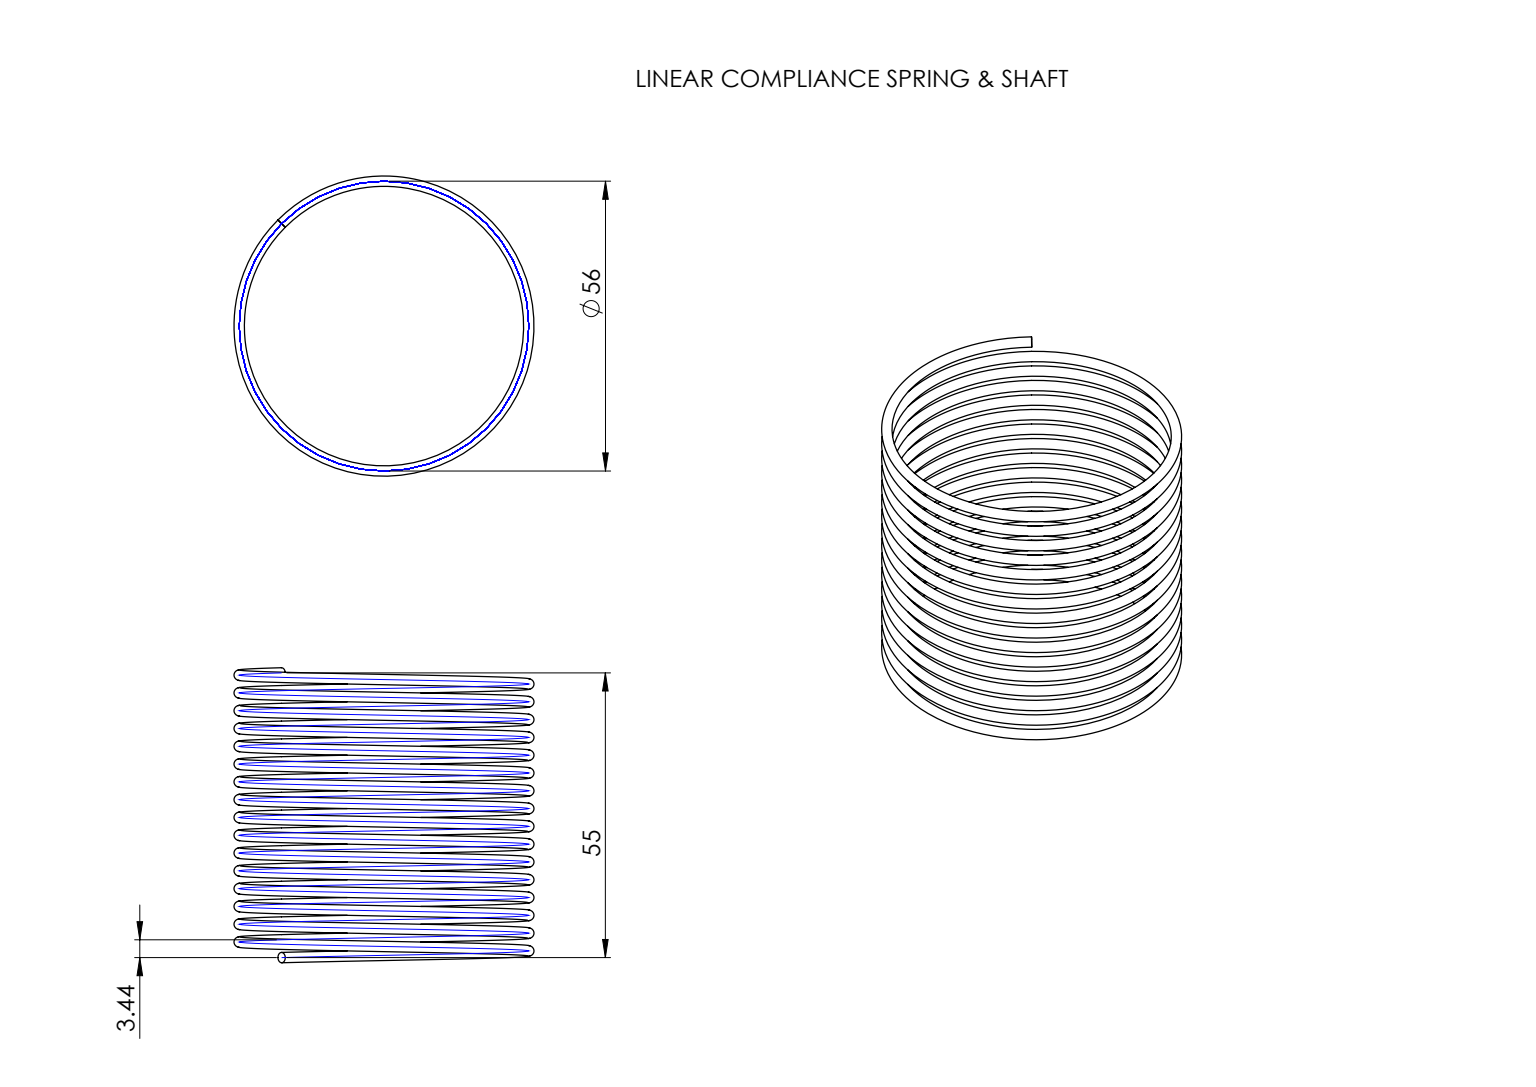
ISO-10303-21;
HEADER;
FILE_DESCRIPTION (('STEP AP214'),
    '1' );
FILE_NAME ('Linear Compliance Spring & Shaft.step',
    '2026-10-02T18:08:48',
    ( '' ),
    ( '' ),
    'SwSTEP 2.0',
    'SolidWorks 2026',
    '' );
FILE_SCHEMA (( 'AUTOMOTIVE_DESIGN' ));
ENDSEC;

DATA;
#1=CARTESIAN_POINT ( 'NONE',  ( -2.584737979205441561E-13, 22.74218749999999645, -30.02300923189239512 ) ) ;
#5=CARTESIAN_POINT ( 'NONE',  ( 0.04044903254992426173, 37.93006916759064495, -30.02300923189239867 ) ) ;
#8=CARTESIAN_POINT ( 'NONE',  ( -2.584737979205441561E-13, 43.36718749999999289, -30.02300923189239512 ) ) ;
#20=CARTESIAN_POINT ( 'NONE',  ( 28.01184896238290278, 23.45833333333333215, -7.505752307973347470 ) ) ;
#25=CARTESIAN_POINT ( 'NONE',  ( -13.94119854578892514, 33.62201416574269075, 24.22776226481266448 ) ) ;
#32=CARTESIAN_POINT ( 'NONE',  ( -26.07999730980477437, 56.11458333333332860, 6.988114217768305103 ) ) ;
#37=CARTESIAN_POINT ( 'NONE',  ( -6.988114217767819270, 38.35416666666666430, 26.07999730980490583 ) ) ;
#38=CARTESIAN_POINT ( 'NONE',  ( 30.02300923189239867, 28.47694416759064495, 0.04044903254992252006 ) ) ;
#39=CARTESIAN_POINT ( 'NONE',  ( 7.543491769121922985, 16.00482666574268720, 28.00173670424535644 ) ) ;
#44=CARTESIAN_POINT ( 'NONE',  ( -14.01125832528328985, 48.51784749907601935, -24.18731323226223040 ) ) ;
#50=CARTESIAN_POINT ( 'NONE',  ( -24.22776226481240514, 43.65923583425730925, 13.94119854578937812 ) ) ;
#54=CARTESIAN_POINT ( 'NONE',  ( 15.01150461594596308, 19.59114583333332149, -26.00068869287367335 ) ) ;
#58=CARTESIAN_POINT ( 'NONE',  ( -7.505752307973343918, 46.66145833333332860, -28.01184896238290989 ) ) ;
#63=CARTESIAN_POINT ( 'NONE',  ( 7.543491769121922985, 64.12982666574268364, 28.00173670424535644 ) ) ;
#69=CARTESIAN_POINT ( 'NONE',  ( 27.95245687107223276, 61.41406250000000711, -2.463307335887066074E-13 ) ) ;
#72=CARTESIAN_POINT ( 'NONE',  ( 24.20753774853731244, 30.19010416666665719, -13.97622843553632599 ) ) ;
#80=CARTESIAN_POINT ( 'NONE',  ( 13.94119854578937812, 56.54986083425731636, 24.22776226481240514 ) ) ;
#91=CARTESIAN_POINT ( 'NONE',  ( -0.04044903254992426173, 15.58631916759064495, 27.95245687107223276 ) ) ;
#95=CARTESIAN_POINT ( 'NONE',  ( 7.505752307972854531, 43.51041666666666430, -28.01184896238303423 ) ) ;
#99=CARTESIAN_POINT ( 'NONE',  ( 28.01184896238304134, 16.86979166666666075, 7.505752307972846538 ) ) ;
#104=CARTESIAN_POINT ( 'NONE',  ( -7.543491769121917656, 31.47357666574268364, -28.00173670424536354 ) ) ;
#106=CARTESIAN_POINT ( 'NONE',  ( 28.01184896238304134, 37.49479166666666430, 7.505752307972846538 ) ) ;
#111=CARTESIAN_POINT ( 'NONE',  ( -24.18731323226221974, 61.40847249907603356, 14.01125832528330406 ) ) ;
#116=CARTESIAN_POINT ( 'NONE',  ( 26.07999730980477437, 16.58333333333333215, -6.988114217768290004 ) ) ;
#125=CARTESIAN_POINT ( 'NONE',  ( 24.22776226481265383, 22.45013916574269075, 13.94119854578893580 ) ) ;
#129=CARTESIAN_POINT ( 'NONE',  ( -19.09188309203694445, 42.93750000000000000, -19.09188309203661049 ) ) ;
#134=CARTESIAN_POINT ( 'NONE',  ( -15.04653450569291984, 63.99777750092396644, 25.98046417659859486 ) ) ;
#135=CARTESIAN_POINT ( 'NONE',  ( -30.02300923189239867, 16.44569416759064140, -0.04044903254991731589 ) ) ;
#146=( LENGTH_UNIT ( ) NAMED_UNIT ( * ) SI_UNIT ( .MILLI., .METRE. ) );
#156=CARTESIAN_POINT ( 'NONE',  ( 0.04044903254993986036, 31.05506916759064495, -27.95245687107223986 ) ) ;
#164=CARTESIAN_POINT ( 'NONE',  ( -7.543491769121917656, 48.66107666574268364, -28.00173670424536354 ) ) ;
#168=CARTESIAN_POINT ( 'NONE',  ( 27.95245687107222921, 20.16406249999999645, -2.463307335887066074E-13 ) ) ;
#171=CARTESIAN_POINT ( 'NONE',  ( 15.01150461594596308, 19.59114583333332149, -26.00068869287367335 ) ) ;
#175=CARTESIAN_POINT ( 'NONE',  ( -0.04044903254990864921, 43.08631916759065916, 30.02300923189239867 ) ) ;
#177=CARTESIAN_POINT ( 'NONE',  ( -26.00068869287368756, 53.10677083333331439, -15.01150461594595775 ) ) ;
#189=CARTESIAN_POINT ( 'NONE',  ( -7.505752307973343918, 26.03645833333333215, -28.01184896238290989 ) ) ;
#194=CARTESIAN_POINT ( 'NONE',  ( 7.025853678916867295, 36.62982666574267654, 26.06988505166722803 ) ) ;
#201=CARTESIAN_POINT ( 'NONE',  ( 19.09188309203694800, 58.40625000000000711, 19.09188309203660694 ) ) ;
#205=CARTESIAN_POINT ( 'NONE',  ( -19.09188309203694445, 42.93750000000000000, -19.09188309203661049 ) ) ;
#206=CARTESIAN_POINT ( 'NONE',  ( -20.47846945139902175, 34.06288166759063785, -20.53372385742072481 ) ) ;
#207=CARTESIAN_POINT ( 'NONE',  ( -25.98046417659831420, 16.72097249907602290, 15.04653450569339945 ) ) ;
#212=CARTESIAN_POINT ( 'NONE',  ( 19.11951029504797006, 43.21836833240935505, 19.06425588902558133 ) ) ;
#218=CARTESIAN_POINT ( 'NONE',  ( -24.18731323226248264, 44.23215250092398065, -14.01125832528284931 ) ) ;
#222=CARTESIAN_POINT ( 'NONE',  ( 15.01150461594643204, 27.61197916666666430, 26.00068869287340334 ) ) ;
#227=CARTESIAN_POINT ( 'NONE',  ( -7.505752307972844761, 48.66666666666666430, 28.01184896238304134 ) ) ;
#235=CARTESIAN_POINT ( 'NONE',  ( -30.02300923189239867, 61.69493083240936926, 0.04044903255044988294 ) ) ;
#241=CARTESIAN_POINT ( 'NONE',  ( 13.97622843553589966, 57.40364583333332860, -24.20753774853756113 ) ) ;
#244=CARTESIAN_POINT ( 'NONE',  ( -27.95245687107222921, 32.19531250000000000, 2.498001805406602216E-13 ) ) ;
#251=CARTESIAN_POINT ( 'NONE',  ( -13.94119854578936923, 54.83111083425730214, -24.22776226481241224 ) ) ;
#262=CARTESIAN_POINT ( 'NONE',  ( 19.06425588902592239, 11.71913166759064318, 19.11951029504763611 ) ) ;
#267=CARTESIAN_POINT ( 'NONE',  ( 28.01184896238290278, 44.08333333333332860, -7.505752307973347470 ) ) ;
#271=CARTESIAN_POINT ( 'NONE',  ( -28.01184896238304134, 25.46354166666666430, -7.505752307972844761 ) ) ;
#277=CARTESIAN_POINT ( 'NONE',  ( -20.53372385742107653, 31.18711833240935150, -20.47846945139867003 ) ) ;
#279=CARTESIAN_POINT ( 'NONE',  ( -20.50609665441004736, 53.25000000000000000, -20.50609665440969565 ) ) ;
#285=CARTESIAN_POINT ( 'NONE',  ( 6.950374756619257965, 62.69753499907601224, -26.09010956794244507 ) ) ;
#291=CARTESIAN_POINT ( 'NONE',  ( -19.09188309203660694, 18.01562499999999645, 19.09188309203694800 ) ) ;
#299=CARTESIAN_POINT ( 'NONE',  ( -7.025853678916861966, 17.72357666574268720, -26.06988505166722803 ) ) ;
#303=CARTESIAN_POINT ( 'NONE',  ( 19.09188309203694800, 48.09375000000000000, 19.09188309203660694 ) ) ;
#307=CARTESIAN_POINT ( 'NONE',  ( -30.02300923189239512, 15.00781249999999467, 2.654126918244515359E-13 ) ) ;
#308=CARTESIAN_POINT ( 'NONE',  ( -25.98046417659859486, 13.29465250092397532, -15.04653450569291628 ) ) ;
#318=SURFACE_SIDE_STYLE ('',( #28646 ) ) ;
#331=CARTESIAN_POINT ( 'NONE',  ( 13.94119854578937812, 25.61236083425731636, 24.22776226481240514 ) ) ;
#339=CARTESIAN_POINT ( 'NONE',  ( 30.02300923189239867, 42.78868083240935505, -0.04044903255044467877 ) ) ;
#343=CARTESIAN_POINT ( 'NONE',  ( 13.97622843553633665, 13.86197916666666430, 24.20753774853730889 ) ) ;
#346=CARTESIAN_POINT ( 'NONE',  ( -7.505752307972844761, 21.16666666666666430, 28.01184896238304134 ) ) ;
#351=CARTESIAN_POINT ( 'NONE',  ( -26.02091320914849959, 36.78423583425730214, 14.97647472619947528 ) ) ;
#353=CARTESIAN_POINT ( 'NONE',  ( -28.01184896238304134, 52.96354166666666430, -7.505752307972844761 ) ) ;
#363=CARTESIAN_POINT ( 'NONE',  ( 7.505752307972854531, 22.88541666666666430, -28.01184896238303423 ) ) ;
#368=CARTESIAN_POINT ( 'NONE',  ( -0.04044903255042732459, 35.05430583240935505, -27.95245687107223986 ) ) ;
#376=CARTESIAN_POINT ( 'NONE',  ( -24.20753774853730889, 62.84635416666667851, 13.97622843553633842 ) ) ;
#380=CARTESIAN_POINT ( 'NONE',  ( -27.95245687107223276, 42.50781249999998579, 2.498001805406602216E-13 ) ) ;
#381=CARTESIAN_POINT ( 'NONE',  ( 0.04044903254992426173, 31.05506916759064495, -30.02300923189239867 ) ) ;
#383=CARTESIAN_POINT ( 'NONE',  ( -20.47846945139866648, 23.45274333240935150, 20.53372385742108008 ) ) ;
#387=CARTESIAN_POINT ( 'NONE',  ( -19.06425588902558133, 44.07774333240935505, 19.11951029504797006 ) ) ;
#393=CARTESIAN_POINT ( 'NONE',  ( 26.09010956794232428, 52.39621500092398065, -6.950374756619718042 ) ) ;
#397=CARTESIAN_POINT ( 'NONE',  ( -7.505752307972844761, 28.04166666666666075, 28.01184896238304134 ) ) ;
#400=CARTESIAN_POINT ( 'NONE',  ( -15.01150461594595775, 45.37239583333333570, 26.00068869287368756 ) ) ;
#407=CARTESIAN_POINT ( 'NONE',  ( -26.02091320914878025, 65.41888916574268364, -14.97647472619899389 ) ) ;
#412=CARTESIAN_POINT ( 'NONE',  ( -6.988114217767819270, 62.41666666666666430, 26.07999730980490583 ) ) ;
#415=CARTESIAN_POINT ( 'NONE',  ( -6.988114217767819270, 31.47916666666666075, 26.07999730980490583 ) ) ;
#420=CARTESIAN_POINT ( 'NONE',  ( -26.06988505166735237, 54.40142333425730925, -7.025853678916388567 ) ) ;
#434=CARTESIAN_POINT ( 'NONE',  ( 27.95245687107223986, 25.03944416759064495, 0.04044903254993640479 ) ) ;
#439=CARTESIAN_POINT ( 'NONE',  ( -28.01184896238304134, 46.08854166666666430, -7.505752307972844761 ) ) ;
#442=CARTESIAN_POINT ( 'NONE',  ( -7.505752307973343918, 19.16145833333332860, -28.01184896238290989 ) ) ;
#449=CARTESIAN_POINT ( 'NONE',  ( -7.468012846824272799, 36.91628499907601224, 28.02196122052058413 ) ) ;
#451=CARTESIAN_POINT ( 'NONE',  ( -26.00068869287340334, 49.09635416666666430, 15.01150461594643559 ) ) ;
#457=CARTESIAN_POINT ( 'NONE',  ( 26.06988505166722803, 63.27045166574269075, -7.025853678916862854 ) ) ;
#463=CARTESIAN_POINT ( 'NONE',  ( 19.09188309203694800, 24.03124999999999645, 19.09188309203660694 ) ) ;
#470=CARTESIAN_POINT ( 'NONE',  ( -19.06425588902558133, 26.89024333240934439, 19.11951029504797006 ) ) ;
#473=CARTESIAN_POINT ( 'NONE',  ( -13.97622843553588901, 48.80989583333332860, 24.20753774853756823 ) ) ;
#477=CARTESIAN_POINT ( 'NONE',  ( 28.01184896238304134, 16.86979166666666075, 7.505752307972846538 ) ) ;
#478=CARTESIAN_POINT ( 'NONE',  ( -7.543491769121417612, 15.72954833425730925, 28.00173670424549499 ) ) ;
#500=CARTESIAN_POINT ( 'NONE',  ( -26.09010956794232428, 36.92746500092395934, 6.950374756619732253 ) ) ;
#508=CARTESIAN_POINT ( 'NONE',  ( 26.02091320914876960, 53.38763916574269786, 14.97647472619900455 ) ) ;
#512=CARTESIAN_POINT ( 'NONE',  ( 19.09188309203694800, 13.71874999999999467, 19.09188309203660694 ) ) ;
#514=CARTESIAN_POINT ( 'NONE',  ( -15.01150461594595775, 17.87239583333332149, 26.00068869287368756 ) ) ;
#517=CARTESIAN_POINT ( 'NONE',  ( 28.02196122052045268, 42.08371500092398065, -7.468012846824774620 ) ) ;
#519=CARTESIAN_POINT ( 'NONE',  ( 28.01184896238304134, 51.24479166666666430, 7.505752307972846538 ) ) ;
#520=CARTESIAN_POINT ( 'NONE',  ( -26.00068869287340334, 66.28385416666662877, 15.01150461594643382 ) ) ;
#529=CARTESIAN_POINT ( 'NONE',  ( 7.505752307973351023, 20.88020833333333215, 28.01184896238290278 ) ) ;
#540=CARTESIAN_POINT ( 'NONE',  ( -2.428612866367529427E-13, 60.55468749999999289, -27.95245687107222921 ) ) ;
#544=CARTESIAN_POINT ( 'NONE',  ( -19.09188309203660694, 42.07812499999999289, 19.09188309203694800 ) ) ;
#546=CARTESIAN_POINT ( 'NONE',  ( -14.97647472619946285, 30.76861083425731280, -26.02091320914851025 ) ) ;
#547=CARTESIAN_POINT ( 'NONE',  ( 7.468012846824281681, 18.01003499907601935, -28.02196122052058058 ) ) ;
#553=CARTESIAN_POINT ( 'NONE',  ( 0.04044903255044120238, 47.08555583240935505, 27.95245687107223276 ) ) ;
#559=CARTESIAN_POINT ( 'NONE',  ( -24.22776226481240514, 50.53423583425731636, 13.94119854578937812 ) ) ;
#563=CARTESIAN_POINT ( 'NONE',  ( -20.50609665440969209, 24.89062500000000000, 20.50609665441005092 ) ) ;
#567=CARTESIAN_POINT ( 'NONE',  ( -7.505752307973343918, 50.09895833333332860, -28.01184896238290989 ) ) ;
#573=CARTESIAN_POINT ( 'NONE',  ( -7.543491769121917656, 58.97357666574269786, -28.00173670424536354 ) ) ;
#577=CARTESIAN_POINT ( 'NONE',  ( -19.09188309203694445, 63.56249999999999289, -19.09188309203661049 ) ) ;
#580=CARTESIAN_POINT ( 'NONE',  ( -24.20753774853756823, 29.04427083333332504, -13.97622843553588723 ) ) ;
#585=CARTESIAN_POINT ( 'NONE',  ( 27.95245687107223986, 59.41444416759064495, 0.04044903254993640479 ) ) ;
#596=CARTESIAN_POINT ( 'NONE',  ( 26.06988505166735592, 25.18267333425730214, 7.025853678916393896 ) ) ;
#600=AXIS2_PLACEMENT_3D ( 'NONE', #12178, #2052, #12527 ) ;
#602=CARTESIAN_POINT ( 'NONE',  ( -30.02300923189239512, 56.25781249999997868, 2.654126918244515359E-13 ) ) ;
#606=CARTESIAN_POINT ( 'NONE',  ( 20.50609665441005092, 24.03124999999999645, 20.50609665440969209 ) ) ;
#614=CARTESIAN_POINT ( 'NONE',  ( -28.02196122052058413, 30.90065999907601579, -7.468012846824272799 ) ) ;
#617=CARTESIAN_POINT ( 'NONE',  ( -15.01150461594595775, 45.37239583333332860, 26.00068869287368756 ) ) ;
#621=CARTESIAN_POINT ( 'NONE',  ( -14.01125832528328985, 62.26784749907602645, -24.18731323226223040 ) ) ;
#627=CARTESIAN_POINT ( 'NONE',  ( 24.20753774853731244, 23.31510416666666430, -13.97622843553633132 ) ) ;
#634=CARTESIAN_POINT ( 'NONE',  ( 7.025853678916867295, 29.75482666574269075, 26.06988505166722803 ) ) ;
#638=CARTESIAN_POINT ( 'NONE',  ( -26.07999730980490583, 52.96354166666666430, -6.988114217767815717 ) ) ;
#643=CARTESIAN_POINT ( 'NONE',  ( 26.00068869287340334, 19.87760416666666430, -15.01150461594642316 ) ) ;
#644=CARTESIAN_POINT ( 'NONE',  ( -20.53372385742071771, 19.45350666759063785, 20.47846945139902530 ) ) ;
#665=CARTESIAN_POINT ( 'NONE',  ( -14.01125832528285109, 43.37277750092397355, 24.18731323226248264 ) ) ;
#672=CARTESIAN_POINT ( 'NONE',  ( -26.02091320914878025, 58.54388916574269075, -14.97647472619899389 ) ) ;
#678=CARTESIAN_POINT ( 'NONE',  ( 6.988114217768294445, 24.31770833333332504, 26.07999730980477437 ) ) ;
#682=CARTESIAN_POINT ( 'NONE',  ( -15.01150461594642138, 32.76822916666666430, -26.00068869287340334 ) ) ;
#685=CARTESIAN_POINT ( 'NONE',  ( 30.02300923189239867, 42.22694416759065206, 0.04044903254992252006 ) ) ;
#687=CARTESIAN_POINT ( 'NONE',  ( 20.50609665441005092, 51.53124999999999289, 20.50609665440969209 ) ) ;
#688=CARTESIAN_POINT ( 'NONE',  ( 2.740863092043355209E-13, 65.71093749999997158, 30.02300923189239512 ) ) ;
#707=CARTESIAN_POINT ( 'NONE',  ( 26.09010956794232428, 14.58371500092397710, -6.950374756619718042 ) ) ;
#712=CARTESIAN_POINT ( 'NONE',  ( -13.97622843553632777, 53.39322916666665719, -24.20753774853731599 ) ) ;
#713=CARTESIAN_POINT ( 'NONE',  ( -15.04653450569291984, 33.06027750092398776, 25.98046417659859486 ) ) ;
#714=CARTESIAN_POINT ( 'NONE',  ( 28.02196122052058413, 32.61940999907601224, 7.468012846824272799 ) ) ;
#718=CARTESIAN_POINT ( 'NONE',  ( 24.22776226481265383, 43.07513916574269786, 13.94119854578893580 ) ) ;
#724=CARTESIAN_POINT ( 'NONE',  ( 26.09010956794232428, 48.95871500092396644, -6.950374756619718042 ) ) ;
#729=CARTESIAN_POINT ( 'NONE',  ( 30.02300923189239512, 23.60156250000000000, -2.619432448724977703E-13 ) ) ;
#733=CARTESIAN_POINT ( 'NONE',  ( 26.00068869287340334, 57.69010416666667140, -15.01150461594642316 ) ) ;
#738=CARTESIAN_POINT ( 'NONE',  ( -13.94119854578892514, 16.43451416574268720, 24.22776226481266448 ) ) ;
#746=CARTESIAN_POINT ( 'NONE',  ( 13.97622843553589966, 40.21614583333332860, -24.20753774853756113 ) ) ;
#753=CARTESIAN_POINT ( 'NONE',  ( 7.025853678916403666, 55.26079833425730214, -26.06988505166735237 ) ) ;
#758=CARTESIAN_POINT ( 'NONE',  ( -15.01150461594642138, 53.39322916666665009, -26.00068869287340334 ) ) ;
#770=CARTESIAN_POINT ( 'NONE',  ( -6.950374756619716266, 24.03684000092397000, -26.09010956794232428 ) ) ;
#775=CARTESIAN_POINT ( 'NONE',  ( -28.01184896238290278, 52.67708333333333570, 7.505752307973363457 ) ) ;
#779=CARTESIAN_POINT ( 'NONE',  ( -26.00068869287368756, 25.60677083333332149, -15.01150461594595775 ) ) ;
#785=CARTESIAN_POINT ( 'NONE',  ( -7.468012846824272799, 40.35378499907601935, 28.02196122052058413 ) ) ;
#787=CARTESIAN_POINT ( 'NONE',  ( -28.01184896238290278, 49.23958333333332860, 7.505752307973363457 ) ) ;
#790=CARTESIAN_POINT ( 'NONE',  ( 0.04044903255044120238, 60.83555583240935505, 27.95245687107223276 ) ) ;
#796=CARTESIAN_POINT ( 'NONE',  ( 13.97622843553589966, 19.59114583333332504, -24.20753774853756113 ) ) ;
#804=CARTESIAN_POINT ( 'NONE',  ( 19.06425588902558133, 28.60899333240935150, -19.11951029504797006 ) ) ;
#809=CARTESIAN_POINT ( 'NONE',  ( 6.988114217767829928, 50.38541666666666430, -26.07999730980489872 ) ) ;
#813=CARTESIAN_POINT ( 'NONE',  ( 26.00068869287340334, 26.75260416666666430, -15.01150461594642316 ) ) ;
#814=CARTESIAN_POINT ( 'NONE',  ( -15.04653450569291984, 22.74777750092397355, 25.98046417659859486 ) ) ;
#832=CARTESIAN_POINT ( 'NONE',  ( -27.95245687107223986, 37.07069416759063785, -0.04044903254993292840 ) ) ;
#839=CARTESIAN_POINT ( 'NONE',  ( -7.468012846824272799, 54.10378499907602645, 28.02196122052058413 ) ) ;
#845=CARTESIAN_POINT ( 'NONE',  ( -27.95245687107222921, 28.75781249999999645, 2.498001805406602216E-13 ) ) ;
#848=CARTESIAN_POINT ( 'NONE',  ( -7.505752307972844761, 28.04166666666666075, 28.01184896238304134 ) ) ;
#851=CARTESIAN_POINT ( 'NONE',  ( -28.00173670424549499, 50.96392333425730925, -7.543491769121417612 ) ) ;
#854=CARTESIAN_POINT ( 'NONE',  ( -28.01184896238290278, 56.11458333333332860, 7.505752307973363457 ) ) ;
#873=CARTESIAN_POINT ( 'NONE',  ( -6.950374756619716266, 13.72434000092397532, -26.09010956794232428 ) ) ;
#879=CARTESIAN_POINT ( 'NONE',  ( 19.09188309203661049, 54.10937499999999289, -19.09188309203694445 ) ) ;
#880=CARTESIAN_POINT ( 'NONE',  ( -20.53372385742071771, 43.51600666759065206, 20.47846945139902530 ) ) ;
#881=CARTESIAN_POINT ( 'NONE',  ( 28.02196122052058413, 25.74440999907601935, 7.468012846824272799 ) ) ;
#884=CARTESIAN_POINT ( 'NONE',  ( 13.94119854578893580, 59.40326416574269075, -24.22776226481265383 ) ) ;
#891=CARTESIAN_POINT ( 'NONE',  ( -24.22776226481240514, 47.09673583425730214, 13.94119854578937812 ) ) ;
#895=CARTESIAN_POINT ( 'NONE',  ( -30.02300923189239512, 25.32031250000000000, 2.654126918244515359E-13 ) ) ;
#899=CARTESIAN_POINT ( 'NONE',  ( -26.00068869287368756, 56.54427083333332149, -15.01150461594595775 ) ) ;
#905=CARTESIAN_POINT ( 'NONE',  ( -6.950374756619247307, 16.29128499907601579, 26.09010956794245217 ) ) ;
#913=CARTESIAN_POINT ( 'NONE',  ( -6.988114217768288228, 43.22395833333332860, -26.07999730980477437 ) ) ;
#919=CARTESIAN_POINT ( 'NONE',  ( -14.97647472619946285, 10.14361083425730925, -26.02091320914851025 ) ) ;
#920=CARTESIAN_POINT ( 'NONE',  ( 28.01184896238304134, 54.68229166666665719, 7.505752307972846538 ) ) ;
#931=CARTESIAN_POINT ( 'NONE',  ( 24.22776226481241224, 21.31548583425730925, -13.94119854578936923 ) ) ;
#937=CARTESIAN_POINT ( 'NONE',  ( -7.505752307972844761, 48.66666666666666430, 28.01184896238304134 ) ) ;
#941=CARTESIAN_POINT ( 'NONE',  ( 20.50609665441005092, 30.90624999999999645, 20.50609665440969209 ) ) ;
#946=CARTESIAN_POINT ( 'NONE',  ( 26.02091320914876960, 39.63763916574268364, 14.97647472619900455 ) ) ;
#948=CARTESIAN_POINT ( 'NONE',  ( 26.00068869287367690, 44.51302083333332860, 15.01150461594596486 ) ) ;
#951=CARTESIAN_POINT ( 'NONE',  ( -6.988114217768288228, 15.72395833333332860, -26.07999730980477437 ) ) ;
#957=CARTESIAN_POINT ( 'NONE',  ( -6.988114217767819270, 24.60416666666666430, 26.07999730980490583 ) ) ;
#964=CARTESIAN_POINT ( 'NONE',  ( 27.95245687107223276, 32.47618083240936215, -0.04044903255042905932 ) ) ;
#968=CARTESIAN_POINT ( 'NONE',  ( 27.95245687107222921, 51.10156249999998579, -2.463307335887066074E-13 ) ) ;
#973=CARTESIAN_POINT ( 'NONE',  ( -20.50609665440969209, 24.89062500000000000, 20.50609665441005092 ) ) ;
#974=CARTESIAN_POINT ( 'NONE',  ( 7.468012846824777284, 22.31809000092397000, 28.02196122052045268 ) ) ;
#982=CARTESIAN_POINT ( 'NONE',  ( -7.468012846824771955, 58.41184000092398065, -28.02196122052045624 ) ) ;
#987=CARTESIAN_POINT ( 'NONE',  ( -0.04044903255042732459, 41.92930583240936215, -27.95245687107223986 ) ) ;
#993=CARTESIAN_POINT ( 'NONE',  ( -14.01125832528285109, 39.93527750092397355, 24.18731323226248264 ) ) ;
#1001=CARTESIAN_POINT ( 'NONE',  ( 7.543491769121922985, 57.25482666574269075, 28.00173670424535644 ) ) ;
#1005=CARTESIAN_POINT ( 'NONE',  ( 26.07999730980477437, 26.89583333333332860, -6.988114217768290004 ) ) ;
#1007=CARTESIAN_POINT ( 'NONE',  ( 15.01150461594596308, 29.90364583333332504, -26.00068869287367335 ) ) ;
#1010=CARTESIAN_POINT ( 'NONE',  ( 26.02091320914851025, 48.81548583425731636, -14.97647472619946463 ) ) ;
#1012=CARTESIAN_POINT ( 'NONE',  ( -30.02300923189239512, 63.13281250000000000, 2.654126918244515359E-13 ) ) ;
#1024=EDGE_CURVE ( 'NONE', #11003, #21772, #28714, .T. ) ;
#1034=CARTESIAN_POINT ( 'NONE',  ( -26.09010956794232428, 16.30246500092397355, 6.950374756619732253 ) ) ;
#1039=CARTESIAN_POINT ( 'NONE',  ( 26.07999730980477437, 47.52083333333332860, -6.988114217768290004 ) ) ;
#1040=CARTESIAN_POINT ( 'NONE',  ( -7.543491769121417612, 36.35454833425730925, 28.00173670424549499 ) ) ;
#1041=CARTESIAN_POINT ( 'NONE',  ( -26.02091320914878025, 24.16888916574269075, -14.97647472619899389 ) ) ;
#1044=CARTESIAN_POINT ( 'NONE',  ( 24.22776226481265383, 60.26263916574269786, 13.94119854578893580 ) ) ;
#1053=CARTESIAN_POINT ( 'NONE',  ( -28.01184896238290278, 32.05208333333332860, 7.505752307973363457 ) ) ;
#1058=CARTESIAN_POINT ( 'NONE',  ( 7.505752307972854531, 53.82291666666666430, -28.01184896238303423 ) ) ;
#1066=CARTESIAN_POINT ( 'NONE',  ( 20.53372385742108008, 67.28086833240935505, 20.47846945139866648 ) ) ;
#1074=CARTESIAN_POINT ( 'NONE',  ( -6.988114217767819270, 38.35416666666666430, 26.07999730980490583 ) ) ;
#1080=CARTESIAN_POINT ( 'NONE',  ( 7.543491769121427382, 10.57329833425730747, -28.00173670424548433 ) ) ;
#1081=CARTESIAN_POINT ( 'NONE',  ( 7.505752307972854531, 50.38541666666666430, -28.01184896238303423 ) ) ;
#1092=CARTESIAN_POINT ( 'NONE',  ( -24.18731323226248264, 20.16965250092397355, -14.01125832528284931 ) ) ;
#1097=CARTESIAN_POINT ( 'NONE',  ( 28.01184896238304134, 51.24479166666666430, 7.505752307972846538 ) ) ;
#1101=CARTESIAN_POINT ( 'NONE',  ( 30.02300923189239512, 33.91406249999997158, -2.619432448724977703E-13 ) ) ;
#1106=CARTESIAN_POINT ( 'NONE',  ( 15.04653450569339945, 39.92409749907602645, 25.98046417659831775 ) ) ;
#1108=CARTESIAN_POINT ( 'NONE',  ( 2.740863092043355209E-13, 62.27343749999999289, 30.02300923189239867 ) ) ;
#1111=CARTESIAN_POINT ( 'NONE',  ( 19.09188309203694800, 17.15624999999999645, 19.09188309203660694 ) ) ;
#1117=CARTESIAN_POINT ( 'NONE',  ( 26.07999730980490227, 30.61979166666666075, 6.988114217767821046 ) ) ;
#1123=CARTESIAN_POINT ( 'NONE',  ( 30.02300923189239867, 22.16368083240936215, -0.04044903255044467877 ) ) ;
#1125=CARTESIAN_POINT ( 'NONE',  ( 0.04044903255044120238, 29.89805583240935860, 27.95245687107223276 ) ) ;
#1129=CARTESIAN_POINT ( 'NONE',  ( 24.20753774853731244, 50.81510416666667140, -13.97622843553632599 ) ) ;
#1134=CARTESIAN_POINT ( 'NONE',  ( 30.02300923189239512, 23.60156250000000000, -2.619432448724977703E-13 ) ) ;
#1135=CARTESIAN_POINT ( 'NONE',  ( -14.97647472619946285, 27.33111083425731280, -26.02091320914851025 ) ) ;
#1146=CARTESIAN_POINT ( 'NONE',  ( -15.04653450569291984, 60.56027750092398065, 25.98046417659859486 ) ) ;
#1149=CARTESIAN_POINT ( 'NONE',  ( -15.01150461594642316, 25.89322916666666430, -26.00068869287341045 ) ) ;
#1154=CARTESIAN_POINT ( 'NONE',  ( 27.95245687107223276, 42.78868083240935505, -0.04044903255042905932 ) ) ;
#1161=CARTESIAN_POINT ( 'NONE',  ( 24.18731323226247554, 42.51340250092398065, 14.01125832528285997 ) ) ;
#1171=CARTESIAN_POINT ( 'NONE',  ( 25.98046417659831775, 59.68972249907602645, -15.04653450569338879 ) ) ;
#1174=CARTESIAN_POINT ( 'NONE',  ( 13.97622843553633665, 24.17447916666666785, 24.20753774853730889 ) ) ;
#1177=CARTESIAN_POINT ( 'NONE',  ( 7.505752307973351023, 34.63020833333332860, 28.01184896238290278 ) ) ;
#1180=CARTESIAN_POINT ( 'NONE',  ( -0.04044903254990864921, 53.39881916759064495, 30.02300923189239867 ) ) ;
#1182=CARTESIAN_POINT ( 'NONE',  ( 20.50609665441005092, 58.40625000000000711, 20.50609665440969209 ) ) ;
#1201=CARTESIAN_POINT ( 'NONE',  ( -19.09188309203694445, 67.00000000000000000, -19.09188309203661049 ) ) ;
#1206=CARTESIAN_POINT ( 'NONE',  ( 19.09188309203661049, 50.67187500000000000, -19.09188309203694445 ) ) ;
#1207=CARTESIAN_POINT ( 'NONE',  ( 15.04653450569292872, 38.21652750092398065, -25.98046417659857710 ) ) ;
#1208=CARTESIAN_POINT ( 'NONE',  ( 25.98046417659831775, 28.75222249907602290, -15.04653450569338879 ) ) ;
#1211=CARTESIAN_POINT ( 'NONE',  ( 0.04044903255044120238, 57.39805583240935505, 27.95245687107223276 ) ) ;
#1215=EDGE_CURVE ( 'NONE', #11003, #16033, #29845, .T. ) ;
#1220=CARTESIAN_POINT ( 'NONE',  ( -28.01184896238304134, 32.33854166666666430, -7.505752307972844761 ) ) ;
#1226=CARTESIAN_POINT ( 'NONE',  ( 28.01184896238290278, 54.39583333333332860, -7.505752307973347470 ) ) ;
#1235=CARTESIAN_POINT ( 'NONE',  ( -19.11951029504797006, 13.99961833240935327, -19.06425588902558133 ) ) ;
#1243=CARTESIAN_POINT ( 'NONE',  ( 13.97622843553633665, 41.36197916666666430, 24.20753774853730889 ) ) ;
#1248=CARTESIAN_POINT ( 'NONE',  ( -14.01125832528285109, 63.99777750092396644, 24.18731323226248264 ) ) ;
#1249=CARTESIAN_POINT ( 'NONE',  ( 30.02300923189239512, 51.10156249999998579, -2.619432448724977703E-13 ) ) ;
#1261=CARTESIAN_POINT ( 'NONE',  ( 6.950374756619721595, 32.63059000092395934, 26.09010956794232428 ) ) ;
#1267=CARTESIAN_POINT ( 'NONE',  ( 15.01150461594643204, 48.23697916666665719, 26.00068869287340334 ) ) ;
#1271=CARTESIAN_POINT ( 'NONE',  ( 2.740863092043355209E-13, 31.33593749999999289, 30.02300923189239512 ) ) ;
#1276=CARTESIAN_POINT ( 'NONE',  ( -7.468012846824272799, 43.79128499907601935, 28.02196122052058413 ) ) ;
#1278=CARTESIAN_POINT ( 'NONE',  ( 30.02300923189239867, 61.41406250000000711, -2.619432448724978208E-13 ) ) ;
#1283=CARTESIAN_POINT ( 'NONE',  ( -27.95245687107223986, 68.56993083240934084, 0.04044903255043252877 ) ) ;
#1289=CARTESIAN_POINT ( 'NONE',  ( -26.07999730980490583, 35.77604166666666430, -6.988114217767815717 ) ) ;
#1294=CARTESIAN_POINT ( 'NONE',  ( 0.04044903255045854962, 26.46055583240935505, 30.02300923189239867 ) ) ;
#1296=CARTESIAN_POINT ( 'NONE',  ( -7.025853678916861966, 41.78607666574268364, -26.06988505166722803 ) ) ;
#1301=CARTESIAN_POINT ( 'NONE',  ( 24.20753774853731244, 54.25260416666666430, -13.97622843553632599 ) ) ;
#1306=CARTESIAN_POINT ( 'NONE',  ( -28.01184896238290278, 21.73958333333332860, 7.505752307973363457 ) ) ;
#1307=CARTESIAN_POINT ( 'NONE',  ( -26.02091320914849959, 26.47173583425730925, 14.97647472619947528 ) ) ;
#1316=CARTESIAN_POINT ( 'NONE',  ( 25.98046417659858420, 56.26340250092398065, 15.04653450569292872 ) ) ;
#1319=CARTESIAN_POINT ( 'NONE',  ( -15.01150461594595775, 31.62239583333333215, 26.00068869287368756 ) ) ;
#1323=MECHANICAL_DESIGN_GEOMETRIC_PRESENTATION_REPRESENTATION('',(#9004),#18345);
#1326=CARTESIAN_POINT ( 'NONE',  ( -27.95245687107223986, 41.06993083240934794, 0.04044903255043252877 ) ) ;
#1332=CARTESIAN_POINT ( 'NONE',  ( 24.18731323226247554, 49.38840250092398776, 14.01125832528285997 ) ) ;
#1340=CARTESIAN_POINT ( 'NONE',  ( 7.543491769121922985, 64.12982666574268364, 28.00173670424535644 ) ) ;
#1344=CARTESIAN_POINT ( 'NONE',  ( -27.95245687107222921, 21.88281249999999645, 2.498001805406602216E-13 ) ) ;
#1347=CARTESIAN_POINT ( 'NONE',  ( 2.740863092043355209E-13, 27.89843750000000000, 30.02300923189239512 ) ) ;
#1351=CARTESIAN_POINT ( 'NONE',  ( -28.02196122052045268, 47.23996500092398065, 7.468012846824790607 ) ) ;
#1354=CARTESIAN_POINT ( 'NONE',  ( 15.01150461594596308, 60.84114583333332860, -26.00068869287367335 ) ) ;
#1376=AXIS2_PLACEMENT_3D ( 'NONE', #6186, #27460, #21818 ) ;
#1377=CARTESIAN_POINT ( 'NONE',  ( 19.11951029504763611, 14.29725666759064318, -19.06425588902591173 ) ) ;
#1382=CARTESIAN_POINT ( 'NONE',  ( 2.584737979205442066E-13, 51.96093750000000000, 27.95245687107223276 ) ) ;
#1383=CARTESIAN_POINT ( 'NONE',  ( -30.02300923189239867, 37.07069416759063785, -0.04044903254991731589 ) ) ;
#1385=CARTESIAN_POINT ( 'NONE',  ( 7.468012846824281681, 28.32253499907601579, -28.02196122052058058 ) ) ;
#1389=CARTESIAN_POINT ( 'NONE',  ( -24.22776226481266448, 51.66888916574269075, -13.94119854578892514 ) ) ;
#1398=CARTESIAN_POINT ( 'NONE',  ( -20.50609665440969209, 38.64062500000000000, 20.50609665441005092 ) ) ;
#1402=CARTESIAN_POINT ( 'NONE',  ( 20.50609665440969565, 57.54687500000000000, -20.50609665441004736 ) ) ;
#1410=CARTESIAN_POINT ( 'NONE',  ( 24.18731323226221974, 18.43972249907602290, -14.01125832528328985 ) ) ;
#1418=CARTESIAN_POINT ( 'NONE',  ( 19.09188309203661049, 43.79687500000000000, -19.09188309203694445 ) ) ;
#1423=CARTESIAN_POINT ( 'NONE',  ( -20.47846945139902175, 13.43788166759064140, -20.53372385742072481 ) ) ;
#1424=CARTESIAN_POINT ( 'NONE',  ( 26.00068869287340334, 57.69010416666667140, -15.01150461594642316 ) ) ;
#1433=CARTESIAN_POINT ( 'NONE',  ( 26.06988505166735592, 28.62017333425730925, 7.025853678916393896 ) ) ;
#1441=CARTESIAN_POINT ( 'NONE',  ( 20.50609665441005092, 61.84374999999998579, 20.50609665440969209 ) ) ;
#1445=CARTESIAN_POINT ( 'NONE',  ( 28.01184896238304134, 27.18229166666666430, 7.505752307972846538 ) ) ;
#1450=CARTESIAN_POINT ( 'NONE',  ( -7.468012846824272799, 47.22878499907602645, 28.02196122052058413 ) ) ;
#1452=CARTESIAN_POINT ( 'NONE',  ( -15.01150461594595775, 62.55989583333332149, 26.00068869287368756 ) ) ;
#1456=CARTESIAN_POINT ( 'NONE',  ( 26.06988505166722803, 66.70795166574268364, -7.025853678916862854 ) ) ;
#1469=CARTESIAN_POINT ( 'NONE',  ( -7.543491769121917656, 21.16107666574269075, -28.00173670424536354 ) ) ;
#1472=CARTESIAN_POINT ( 'NONE',  ( -19.11951029504797006, 38.06211833240934084, -19.06425588902558133 ) ) ;
#1476=CARTESIAN_POINT ( 'NONE',  ( -13.97622843553588901, 62.55989583333332860, 24.20753774853756823 ) ) ;
#1481=CARTESIAN_POINT ( 'NONE',  ( -7.505752307973343918, 36.34895833333333570, -28.01184896238290989 ) ) ;
#1482=CARTESIAN_POINT ( 'NONE',  ( -28.02196122052045268, 30.05246500092397000, 7.468012846824790607 ) ) ;
#1491=CARTESIAN_POINT ( 'NONE',  ( -26.02091320914849959, 53.97173583425732346, 14.97647472619947528 ) ) ;
#1494=CARTESIAN_POINT ( 'NONE',  ( -20.50609665440969209, 31.76562499999999289, 20.50609665441005092 ) ) ;
#1498=CARTESIAN_POINT ( 'NONE',  ( -13.94119854578892514, 43.93451416574269075, 24.22776226481266448 ) ) ;
#1504=CARTESIAN_POINT ( 'NONE',  ( 24.22776226481241224, 45.37798583425732346, -13.94119854578936923 ) ) ;
#1511=CARTESIAN_POINT ( 'NONE',  ( -0.04044903255044120238, 62.55430583240935505, -30.02300923189239867 ) ) ;
#1516=CARTESIAN_POINT ( 'NONE',  ( 6.988114217768294445, 31.19270833333333215, 26.07999730980477437 ) ) ;
#1519=CARTESIAN_POINT ( 'NONE',  ( 7.505752307972854531, 36.63541666666666430, -28.01184896238303423 ) ) ;
#1523=CARTESIAN_POINT ( 'NONE',  ( 26.02091320914851025, 52.25298583425730925, -14.97647472619946463 ) ) ;
#1524=CARTESIAN_POINT ( 'NONE',  ( 26.09010956794232428, 55.83371500092398065, -6.950374756619718042 ) ) ;
#1526=CARTESIAN_POINT ( 'NONE',  ( 15.01150461594643204, 61.98697916666665009, 26.00068869287340334 ) ) ;
#1544=CARTESIAN_POINT ( 'NONE',  ( 26.06988505166735592, 21.74517333425730925, 7.025853678916393896 ) ) ;
#1549=CARTESIAN_POINT ( 'NONE',  ( 27.95245687107223276, 54.53906249999999289, -2.463307335887066074E-13 ) ) ;
#1550=CARTESIAN_POINT ( 'NONE',  ( -30.02300923189239867, 43.94569416759065206, -0.04044903254991731589 ) ) ;
#1551=CARTESIAN_POINT ( 'NONE',  ( -26.02091320914878025, 34.48138916574268364, -14.97647472619899389 ) ) ;
#1554=CARTESIAN_POINT ( 'NONE',  ( 26.06988505166722803, 66.70795166574268364, -7.025853678916862854 ) ) ;
#1556=CARTESIAN_POINT ( 'NONE',  ( 28.01184896238290278, 13.14583333333332860, -7.505752307973347470 ) ) ;
#1562=CARTESIAN_POINT ( 'NONE',  ( 26.00068869287340334, 33.62760416666665719, -15.01150461594642316 ) ) ;
#1568=CARTESIAN_POINT ( 'NONE',  ( 20.50609665440969565, 64.42187499999998579, -20.50609665441004736 ) ) ;
#1576=CARTESIAN_POINT ( 'NONE',  ( -24.22776226481266448, 20.73138916574268720, -13.94119854578892514 ) ) ;
#1584=CARTESIAN_POINT ( 'NONE',  ( 19.09188309203661049, 50.67187500000000000, -19.09188309203694445 ) ) ;
#1589=CARTESIAN_POINT ( 'NONE',  ( 28.00173670424549499, 14.87017333425730747, 7.543491769121417612 ) ) ;
#1590=CARTESIAN_POINT ( 'NONE',  ( 20.50609665440969565, 60.98437499999999289, -20.50609665441004736 ) ) ;
#1602=CARTESIAN_POINT ( 'NONE',  ( -26.09010956794232428, 36.92746500092395934, 6.950374756619732253 ) ) ;
#1606=CARTESIAN_POINT ( 'NONE',  ( 15.01150461594596308, 57.40364583333333570, -26.00068869287367335 ) ) ;
#1610=CARTESIAN_POINT ( 'NONE',  ( 30.02300923189239512, 27.03906250000000000, -2.619432448724977703E-13 ) ) ;
#1615=CARTESIAN_POINT ( 'NONE',  ( 20.53372385742108008, 53.53086833240935505, 20.47846945139866648 ) ) ;
#1617=CARTESIAN_POINT ( 'NONE',  ( 2.740863092043355209E-13, 55.39843749999999289, 30.02300923189239867 ) ) ;
#1622=CARTESIAN_POINT ( 'NONE',  ( -24.22776226481266448, 68.85638916574269786, -13.94119854578892514 ) ) ;
#1632=CARTESIAN_POINT ( 'NONE',  ( 28.00173670424535644, 25.45795166574268364, -7.543491769121920321 ) ) ;
#1635=CARTESIAN_POINT ( 'NONE',  ( -0.04044903255042732459, 38.49180583240935505, -27.95245687107223986 ) ) ;
#1640=CARTESIAN_POINT ( 'NONE',  ( 24.20753774853731244, 61.12760416666665719, -13.97622843553632599 ) ) ;
#1646=CARTESIAN_POINT ( 'NONE',  ( 26.00068869287340334, 37.06510416666666430, -15.01150461594642316 ) ) ;
#1647=CARTESIAN_POINT ( 'NONE',  ( 15.04653450569292872, 34.77902750092397355, -25.98046417659857710 ) ) ;
#1657=CARTESIAN_POINT ( 'NONE',  ( 25.98046417659858420, 59.70090250092397355, 15.04653450569292872 ) ) ;
#1660=CARTESIAN_POINT ( 'NONE',  ( 30.02300923189239867, 27.03906250000000000, -2.619432448724978208E-13 ) ) ;
#1665=CARTESIAN_POINT ( 'NONE',  ( 24.18731323226221974, 45.93972249907602645, -14.01125832528328985 ) ) ;
#1672=CARTESIAN_POINT ( 'NONE',  ( -6.950374756619716266, 51.53684000092397355, -26.09010956794232428 ) ) ;
#1679=CARTESIAN_POINT ( 'NONE',  ( -7.468012846824272799, 67.85378499907602645, 28.02196122052058413 ) ) ;
#1685=CARTESIAN_POINT ( 'NONE',  ( -19.09188309203660694, 31.76562499999999289, 19.09188309203694800 ) ) ;
#1688=CARTESIAN_POINT ( 'NONE',  ( 15.01150461594596308, 40.21614583333332860, -26.00068869287367335 ) ) ;
#1691=CARTESIAN_POINT ( 'NONE',  ( 15.04653450569292872, 58.84152750092397355, -25.98046417659857710 ) ) ;
#1692=CARTESIAN_POINT ( 'NONE',  ( -19.06425588902591173, 65.00038166759063074, -19.11951029504763611 ) ) ;
#1695=CARTESIAN_POINT ( 'NONE',  ( 26.00068869287367335, 58.26302083333332149, 15.01150461594596308 ) ) ;
#1714=CARTESIAN_POINT ( 'NONE',  ( -14.01125832528285109, 22.74777750092397355, 24.18731323226248264 ) ) ;
#1719=CARTESIAN_POINT ( 'NONE',  ( -30.02300923189239867, 47.38319416759065206, -0.04044903254991731589 ) ) ;
#1720=CARTESIAN_POINT ( 'NONE',  ( 7.543491769121922985, 40.06732666574268364, 28.00173670424535644 ) ) ;
#1723=CARTESIAN_POINT ( 'NONE',  ( 26.09010956794244507, 66.99440999907601224, 6.950374756619249084 ) ) ;
#1726=CARTESIAN_POINT ( 'NONE',  ( 28.01184896238290278, 16.58333333333333215, -7.505752307973347470 ) ) ;
#1733=CARTESIAN_POINT ( 'NONE',  ( -15.01150461594595775, 31.62239583333332860, 26.00068869287368756 ) ) ;
#1741=CARTESIAN_POINT ( 'NONE',  ( -20.50609665441004736, 15.43749999999999645, -20.50609665440969565 ) ) ;
#1746=CARTESIAN_POINT ( 'NONE',  ( 27.95245687107223276, 29.03868083240935505, -0.04044903255042905932 ) ) ;
#1754=CARTESIAN_POINT ( 'NONE',  ( -2.428612866367529427E-13, 46.80468750000000000, -27.95245687107222921 ) ) ;
#1759=CARTESIAN_POINT ( 'NONE',  ( 7.543491769121427382, 20.88579833425730925, -28.00173670424548433 ) ) ;
#1760=CARTESIAN_POINT ( 'NONE',  ( -28.01184896238290278, 59.55208333333332149, 7.505752307973363457 ) ) ;
#1772=CARTESIAN_POINT ( 'NONE',  ( 13.94119854578937812, 32.48736083425731636, 24.22776226481240514 ) ) ;
#1781=CARTESIAN_POINT ( 'NONE',  ( -7.505752307972844761, 38.35416666666666430, 28.01184896238304134 ) ) ;
#1787=CARTESIAN_POINT ( 'NONE',  ( 25.98046417659831775, 56.25222249907602645, -15.04653450569338879 ) ) ;
#1789=CARTESIAN_POINT ( 'NONE',  ( 28.01184896238290278, 61.27083333333332860, -7.505752307973347470 ) ) ;
#1795=CARTESIAN_POINT ( 'NONE',  ( 24.20753774853756113, 27.32552083333332860, 13.97622843553589789 ) ) ;
#1808=CARTESIAN_POINT ( 'NONE',  ( -28.00173670424535644, 27.17670166574268009, 7.543491769121936308 ) ) ;
#1810=CARTESIAN_POINT ( 'NONE',  ( 0.04044903255044120238, 33.33555583240935505, 27.95245687107223276 ) ) ;
#1814=CARTESIAN_POINT ( 'NONE',  ( 24.20753774853756113, 61.70052083333331439, 13.97622843553589789 ) ) ;
#1819=CARTESIAN_POINT ( 'NONE',  ( 15.01150461594596308, 29.90364583333332504, -26.00068869287367335 ) ) ;
#1820=CARTESIAN_POINT ( 'NONE',  ( -0.04044903254990864921, 29.33631916759064850, 30.02300923189239867 ) ) ;
#1831=CARTESIAN_POINT ( 'NONE',  ( 28.01184896238290278, 16.58333333333333215, -7.505752307973347470 ) ) ;
#1834=CARTESIAN_POINT ( 'NONE',  ( -15.01150461594642316, 32.76822916666666430, -26.00068869287341045 ) ) ;
#1839=CARTESIAN_POINT ( 'NONE',  ( 27.95245687107223276, 49.66368083240936215, -0.04044903255042905932 ) ) ;
#1846=CARTESIAN_POINT ( 'NONE',  ( 19.06425588902592239, 52.96913166759063785, 19.11951029504763611 ) ) ;
#1856=CARTESIAN_POINT ( 'NONE',  ( -14.97647472619899389, 67.99701416574269786, 26.02091320914878025 ) ) ;
#1861=CARTESIAN_POINT ( 'NONE',  ( -26.07999730980490583, 32.33854166666666430, -6.988114217767815717 ) ) ;
#1863=CARTESIAN_POINT ( 'NONE',  ( -28.01184896238304134, 39.21354166666666430, -7.505752307972844761 ) ) ;
#1866=CARTESIAN_POINT ( 'NONE',  ( -0.04044903254990864921, 56.83631916759064495, 30.02300923189239867 ) ) ;
#1867=CARTESIAN_POINT ( 'NONE',  ( -26.09010956794232428, 57.55246500092398065, 6.950374756619732253 ) ) ;
#1869=CARTESIAN_POINT ( 'NONE',  ( -0.04044903255044120238, 17.86680583240935860, -30.02300923189239867 ) ) ;
#1890=CARTESIAN_POINT ( 'NONE',  ( 7.025853678916403666, 17.44829833425730925, -26.06988505166735237 ) ) ;
#1896=CARTESIAN_POINT ( 'NONE',  ( -30.02300923189239867, 50.82069416759063785, -0.04044903254991731589 ) ) ;
#1899=CARTESIAN_POINT ( 'NONE',  ( -15.04653450569338524, 38.20534749907601935, -25.98046417659831775 ) ) ;
#1902=CARTESIAN_POINT ( 'NONE',  ( -14.01125832528328985, 65.70534749907602645, -24.18731323226223040 ) ) ;
#1911=CARTESIAN_POINT ( 'NONE',  ( 7.505752307972854531, 46.94791666666666430, -28.01184896238303423 ) ) ;
#1919=CARTESIAN_POINT ( 'NONE',  ( 20.50609665440969565, 12.85937500000000000, -20.50609665441004736 ) ) ;
#1925=CARTESIAN_POINT ( 'NONE',  ( 24.18731323226221974, 21.87722249907602290, -14.01125832528328985 ) ) ;
#1933=CARTESIAN_POINT ( 'NONE',  ( -19.09188309203694445, 49.81249999999999289, -19.09188309203661049 ) ) ;
#1937=CARTESIAN_POINT ( 'NONE',  ( -26.07999730980490583, 28.90104166666666785, -6.988114217767815717 ) ) ;
#1939=CARTESIAN_POINT ( 'NONE',  ( 20.47846945139902530, 22.03163166759064495, 20.53372385742071771 ) ) ;
#1941=CARTESIAN_POINT ( 'NONE',  ( -28.01184896238304134, 59.83854166666666430, -7.505752307972844761 ) ) ;
#1955=CARTESIAN_POINT ( 'NONE',  ( -14.01125832528285109, 33.06027750092398776, 24.18731323226248264 ) ) ;
#1959=CARTESIAN_POINT ( 'NONE',  ( -26.00068869287340334, 18.15885416666666075, 15.01150461594643382 ) ) ;
#1964=CARTESIAN_POINT ( 'NONE',  ( 15.01150461594596308, 36.77864583333332860, -26.00068869287367335 ) ) ;
#1969=CARTESIAN_POINT ( 'NONE',  ( 0.04044903255045854962, 53.96055583240936926, 30.02300923189239867 ) ) ;
#1971=CARTESIAN_POINT ( 'NONE',  ( 2.740863092043355209E-13, 65.71093749999998579, 30.02300923189239867 ) ) ;
#1976=CARTESIAN_POINT ( 'NONE',  ( -19.09188309203660694, 24.89062500000000000, 19.09188309203694800 ) ) ;
#1988=CARTESIAN_POINT ( 'NONE',  ( -13.94119854578892514, 37.05951416574268364, 24.22776226481266448 ) ) ;
#1992=CARTESIAN_POINT ( 'NONE',  ( 2.584737979205441561E-13, 62.27343749999999289, 27.95245687107222921 ) ) ;
#1997=CARTESIAN_POINT ( 'NONE',  ( -26.00068869287340334, 35.34635416666666430, 15.01150461594643382 ) ) ;
#1998=CARTESIAN_POINT ( 'NONE',  ( 7.543491769121427382, 31.19829833425730570, -28.00173670424548433 ) ) ;
#2008=CARTESIAN_POINT ( 'NONE',  ( 7.468012846824777284, 63.56809000092398065, 28.02196122052045268 ) ) ;
#2011=CARTESIAN_POINT ( 'NONE',  ( 2.740863092043355209E-13, 34.77343750000000000, 30.02300923189239867 ) ) ;
#2017=CARTESIAN_POINT ( 'NONE',  ( -19.11951029504797006, 48.37461833240936215, -19.06425588902558133 ) ) ;
#2030=DIRECTION ( 'NONE',  ( -0.7071067811865526798, 0.000000000000000000, -0.7071067811865423547 ) ) ;
#2032=CARTESIAN_POINT ( 'NONE',  ( -15.04653450569338524, 62.26784749907602645, -25.98046417659831775 ) ) ;
#2037=CARTESIAN_POINT ( 'NONE',  ( 26.07999730980477437, 33.77083333333333570, -6.988114217768290004 ) ) ;
#2040=CARTESIAN_POINT ( 'NONE',  ( -7.505752307973343918, 36.34895833333333570, -28.01184896238290989 ) ) ;
#2043=CARTESIAN_POINT ( 'NONE',  ( 7.543491769121427382, 55.26079833425730214, -28.00173670424548433 ) ) ;
#2044=CARTESIAN_POINT ( 'NONE',  ( -14.01125832528285109, 57.12277750092398065, 24.18731323226248264 ) ) ;
#2046=CARTESIAN_POINT ( 'NONE',  ( -0.04044903255044120238, 14.42930583240935505, -30.02300923189239867 ) ) ;
#2052=DIRECTION ( 'NONE',  ( -0.7069718413157907166, -0.01953538259431466736, 0.7069718413158010417 ) ) ;
#2065=CARTESIAN_POINT ( 'NONE',  ( 6.950374756619721595, 18.88059000092397355, 26.09010956794232428 ) ) ;
#2070=CARTESIAN_POINT ( 'NONE',  ( 15.04653450569292872, 45.09152750092398065, -25.98046417659857710 ) ) ;
#2072=CARTESIAN_POINT ( 'NONE',  ( 14.97647472619900455, 38.77826416574269075, -26.02091320914876960 ) ) ;
#2077=CARTESIAN_POINT ( 'NONE',  ( 7.025853678916867295, 67.56732666574268364, 26.06988505166722803 ) ) ;
#2080=CARTESIAN_POINT ( 'NONE',  ( -15.01150461594595775, 14.43489583333332682, 26.00068869287368756 ) ) ;
#2086=CARTESIAN_POINT ( 'NONE',  ( 28.01184896238304134, 40.93229166666666430, 7.505752307972846538 ) ) ;
#2093=ADVANCED_FACE ( 'NONE', ( #12724 ), #6400, .T. ) ;
#2096=CARTESIAN_POINT ( 'NONE',  ( -15.01150461594642316, 12.14322916666666430, -26.00068869287341045 ) ) ;
#2101=CARTESIAN_POINT ( 'NONE',  ( 26.06988505166722803, 22.02045166574269075, -7.025853678916862854 ) ) ;
#2109=CARTESIAN_POINT ( 'NONE',  ( -13.97622843553588901, 52.24739583333332860, 24.20753774853756823 ) ) ;
#2113=CARTESIAN_POINT ( 'NONE',  ( -24.20753774853730889, 31.90885416666666785, 13.97622843553634020 ) ) ;
#2114=CARTESIAN_POINT ( 'NONE',  ( 7.468012846824777284, 22.31809000092397000, 28.02196122052045268 ) ) ;
#2115=CARTESIAN_POINT ( 'NONE',  ( -30.02300923189239512, 63.13281250000000000, 2.654126918244515359E-13 ) ) ;
#2124=CARTESIAN_POINT ( 'NONE',  ( 6.950374756619721595, 39.50559000092398065, 26.09010956794232428 ) ) ;
#2128=CARTESIAN_POINT ( 'NONE',  ( -7.505752307972844761, 14.29166666666666430, 28.01184896238304134 ) ) ;
#2133=CARTESIAN_POINT ( 'NONE',  ( 28.01184896238290278, 37.20833333333332860, -7.505752307973347470 ) ) ;
#2138=CARTESIAN_POINT ( 'NONE',  ( 0.04044903255045854962, 50.52305583240934794, 30.02300923189239867 ) ) ;
#2145=CARTESIAN_POINT ( 'NONE',  ( 24.20753774853756113, 20.45052083333332504, 13.97622843553589789 ) ) ;
#2161=CARTESIAN_POINT ( 'NONE',  ( -24.22776226481240514, 16.15923583425731636, 13.94119854578937812 ) ) ;
#2165=CARTESIAN_POINT ( 'NONE',  ( -28.01184896238290278, 35.48958333333332860, 7.505752307973363457 ) ) ;
#2177=CARTESIAN_POINT ( 'NONE',  ( -15.01150461594642138, 12.14322916666666430, -26.00068869287340334 ) ) ;
#2180=CARTESIAN_POINT ( 'NONE',  ( -28.01184896238290278, 38.92708333333333570, 7.505752307973363457 ) ) ;
#2185=CARTESIAN_POINT ( 'NONE',  ( 26.09010956794244507, 56.68190999907602645, 6.950374756619249084 ) ) ;
#2190=CARTESIAN_POINT ( 'NONE',  ( 26.07999730980490227, 16.86979166666666075, 6.988114217767821046 ) ) ;
#2198=CARTESIAN_POINT ( 'NONE',  ( 24.18731323226221974, 15.00222249907602112, -14.01125832528328985 ) ) ;
#2202=CARTESIAN_POINT ( 'NONE',  ( 6.988114217767829928, 33.19791666666665719, -26.07999730980489872 ) ) ;
#2205=CARTESIAN_POINT ( 'NONE',  ( -20.50609665440969209, 48.95312500000000000, 20.50609665441005092 ) ) ;
#2208=CARTESIAN_POINT ( 'NONE',  ( 14.97647472619947351, 59.98736083425730925, 26.02091320914850314 ) ) ;
#2209=CARTESIAN_POINT ( 'NONE',  ( -0.04044903254992426173, 56.83631916759064495, 27.95245687107223276 ) ) ;
#2211=CARTESIAN_POINT ( 'NONE',  ( -20.50609665441004736, 67.00000000000000000, -20.50609665440969565 ) ) ;
#2216=CARTESIAN_POINT ( 'NONE',  ( -26.00068869287368756, 63.41927083333333570, -15.01150461594595775 ) ) ;
#2235=CARTESIAN_POINT ( 'NONE',  ( 27.95245687107223986, 25.03944416759064495, 0.04044903254993640479 ) ) ;
#2240=CARTESIAN_POINT ( 'NONE',  ( -28.00173670424549499, 50.96392333425730925, -7.543491769121417612 ) ) ;
#2243=CARTESIAN_POINT ( 'NONE',  ( -15.04653450569338524, 41.64284749907602645, -25.98046417659831775 ) ) ;
#2247=CARTESIAN_POINT ( 'NONE',  ( 14.01125832528330051, 63.98659749907601935, 24.18731323226221974 ) ) ;
#2250=CARTESIAN_POINT ( 'NONE',  ( 2.740863092043355209E-13, 14.14843749999999289, 30.02300923189239512 ) ) ;
#2257=CARTESIAN_POINT ( 'NONE',  ( -30.02300923189239512, 39.07031249999997868, 2.654126918244515359E-13 ) ) ;
#2258=CARTESIAN_POINT ( 'NONE',  ( -15.01150461594595775, 59.12239583333333570, 26.00068869287368756 ) ) ;
#2274=CARTESIAN_POINT ( 'NONE',  ( 13.94119854578893580, 21.59076416574269430, -24.22776226481265383 ) ) ;
#2282=CARTESIAN_POINT ( 'NONE',  ( 26.07999730980477437, 54.39583333333332860, -6.988114217768290004 ) ) ;
#2286=CARTESIAN_POINT ( 'NONE',  ( -2.428612866367529427E-13, 33.05468750000000000, -27.95245687107223276 ) ) ;
#2288=CARTESIAN_POINT ( 'NONE',  ( 28.02196122052045268, 18.02121500092397710, -7.468012846824774620 ) ) ;
#2289=CARTESIAN_POINT ( 'NONE',  ( 26.00068869287367335, 65.13802083333334281, 15.01150461594596308 ) ) ;
#2301=CARTESIAN_POINT ( 'NONE',  ( -19.11951029504763611, 40.07850666759064495, 19.06425588902592239 ) ) ;
#2305=CARTESIAN_POINT ( 'NONE',  ( 28.01184896238304134, 20.30729166666666430, 7.505752307972846538 ) ) ;
#2309=CARTESIAN_POINT ( 'NONE',  ( 15.01150461594643204, 37.92447916666666430, 26.00068869287340334 ) ) ;
#2314=CARTESIAN_POINT ( 'NONE',  ( -0.04044903255044120238, 52.24180583240936215, -30.02300923189239867 ) ) ;
#2321=CARTESIAN_POINT ( 'NONE',  ( 6.988114217767829928, 22.88541666666666430, -26.07999730980489872 ) ) ;
#2338=CARTESIAN_POINT ( 'NONE',  ( 26.06988505166735592, 11.43267333425730925, 7.025853678916393896 ) ) ;
#2343=CARTESIAN_POINT ( 'NONE',  ( 30.02300923189239512, 44.22656249999997868, -2.619432448724977703E-13 ) ) ;
#2354=CARTESIAN_POINT ( 'NONE',  ( 20.53372385742072481, 62.42225666759065206, -20.47846945139902175 ) ) ;
#2355=CARTESIAN_POINT ( 'NONE',  ( 15.01150461594596486, 40.21614583333332860, -26.00068869287367690 ) ) ;
#2362=CARTESIAN_POINT ( 'NONE',  ( -24.22776226481266448, 48.23138916574269786, -13.94119854578892514 ) ) ;
#2369=CARTESIAN_POINT ( 'NONE',  ( 13.97622843553633842, 17.29947916666666430, 24.20753774853730889 ) ) ;
#2376=CARTESIAN_POINT ( 'NONE',  ( 24.22776226481265383, 19.01263916574269075, 13.94119854578893580 ) ) ;
#2382=CARTESIAN_POINT ( 'NONE',  ( -13.97622843553632421, 43.08072916666666430, -24.20753774853731599 ) ) ;
#2386=CARTESIAN_POINT ( 'NONE',  ( 15.01150461594643204, 44.79947916666667140, 26.00068869287340334 ) ) ;
#2388=CARTESIAN_POINT ( 'NONE',  ( -25.98046417659859486, 61.41965250092398776, -15.04653450569291628 ) ) ;
#2389=CARTESIAN_POINT ( 'NONE',  ( -24.22776226481240514, 60.84673583425731636, 13.94119854578937812 ) ) ;
#2392=CARTESIAN_POINT ( 'NONE',  ( -28.00173670424535644, 20.30170166574269075, 7.543491769121936308 ) ) ;
#2398=CARTESIAN_POINT ( 'NONE',  ( -20.50609665441004736, 67.00000000000000000, -20.50609665440969565 ) ) ;
#2414=CARTESIAN_POINT ( 'NONE',  ( 27.95245687107223986, 31.91444416759064495, 0.04044903254993640479 ) ) ;
#2420=CARTESIAN_POINT ( 'NONE',  ( 20.47846945139867003, 49.23399333240936215, -20.53372385742107653 ) ) ;
#2424=CARTESIAN_POINT ( 'NONE',  ( -13.97622843553632421, 15.58072916666666607, -24.20753774853731599 ) ) ;
#2427=CARTESIAN_POINT ( 'NONE',  ( -28.01184896238304134, 22.02604166666666430, -7.505752307972844761 ) ) ;
#2434=CARTESIAN_POINT ( 'NONE',  ( -15.01150461594595775, 45.37239583333333570, 26.00068869287368756 ) ) ;
#2435=CARTESIAN_POINT ( 'NONE',  ( 26.00068869287367335, 61.70052083333331439, 15.01150461594596308 ) ) ;
#2450=CARTESIAN_POINT ( 'NONE',  ( -19.06425588902558133, 37.20274333240935505, 19.11951029504797006 ) ) ;
#2458=CARTESIAN_POINT ( 'NONE',  ( -2.428612866367529427E-13, 57.11718750000000711, -27.95245687107222921 ) ) ;
#2462=CARTESIAN_POINT ( 'NONE',  ( -6.988114217767819270, 41.79166666666666430, 26.07999730980490583 ) ) ;
#2463=CARTESIAN_POINT ( 'NONE',  ( 28.02196122052045268, 24.89621500092397710, -7.468012846824774620 ) ) ;
#2464=CARTESIAN_POINT ( 'NONE',  ( 26.02091320914876960, 19.01263916574269075, 14.97647472619900455 ) ) ;
#2475=CARTESIAN_POINT ( 'NONE',  ( -26.06988505166735237, 40.65142333425730214, -7.025853678916388567 ) ) ;
#2479=CARTESIAN_POINT ( 'NONE',  ( -28.01184896238304134, 18.58854166666666430, -7.505752307972844761 ) ) ;
#2484=CARTESIAN_POINT ( 'NONE',  ( -15.01150461594595775, 48.80989583333332860, 26.00068869287368756 ) ) ;
#2488=CARTESIAN_POINT ( 'NONE',  ( 7.543491769121922985, 60.69232666574269075, 28.00173670424535644 ) ) ;
#2490=CARTESIAN_POINT ( 'NONE',  ( -20.50609665441004736, 67.00000000000000000, -20.50609665440969565 ) ) ;
#2493=CARTESIAN_POINT ( 'NONE',  ( -13.97622843553632777, 56.83072916666665719, -24.20753774853731599 ) ) ;
#2496=CARTESIAN_POINT ( 'NONE',  ( 13.97622843553589966, 26.46614583333332149, -24.20753774853756113 ) ) ;
#2503=CARTESIAN_POINT ( 'NONE',  ( 7.025853678916403666, 44.94829833425730925, -26.06988505166735237 ) ) ;
#2516=CARTESIAN_POINT ( 'NONE',  ( 26.06988505166735592, 14.87017333425730747, 7.025853678916393896 ) ) ;
#2520=CARTESIAN_POINT ( 'NONE',  ( -20.50609665441004736, 42.93750000000000000, -20.50609665440969565 ) ) ;
#2531=CARTESIAN_POINT ( 'NONE',  ( 15.01150461594643204, 13.86197916666666430, 26.00068869287340334 ) ) ;
#2533=CARTESIAN_POINT ( 'NONE',  ( -20.50609665441004736, 39.49999999999999289, -20.50609665440969565 ) ) ;
#2540=CARTESIAN_POINT ( 'NONE',  ( -26.06988505166722803, 54.67670166574269075, 7.025853678916877953 ) ) ;
#2546=CARTESIAN_POINT ( 'NONE',  ( 19.09188309203661049, 12.85937500000000000, -19.09188309203694445 ) ) ;
#2554=CARTESIAN_POINT ( 'NONE',  ( -0.04044903255042732459, 21.30430583240935860, -27.95245687107223986 ) ) ;
#2558=CARTESIAN_POINT ( 'NONE',  ( -19.09188309203694445, 46.37500000000000000, -19.09188309203661049 ) ) ;
#2561=CARTESIAN_POINT ( 'NONE',  ( -15.01150461594642138, 46.51822916666666430, -26.00068869287340334 ) ) ;
#2563=CARTESIAN_POINT ( 'NONE',  ( 15.01150461594596308, 12.71614583333333037, -26.00068869287367335 ) ) ;
#2564=CARTESIAN_POINT ( 'NONE',  ( 0.04044903254992426173, 10.43006916759064495, -30.02300923189239867 ) ) ;
#2574=CARTESIAN_POINT ( 'NONE',  ( -28.01184896238290278, 66.42708333333332860, 7.505752307973363457 ) ) ;
#2588=CARTESIAN_POINT ( 'NONE',  ( -24.22776226481240514, 33.34673583425730214, 13.94119854578937812 ) ) ;
#2595=CARTESIAN_POINT ( 'NONE',  ( 0.04044903255045854962, 47.08555583240935505, 30.02300923189239867 ) ) ;
#2599=CARTESIAN_POINT ( 'NONE',  ( 19.09188309203694800, 20.59374999999999645, 19.09188309203660694 ) ) ;
#2603=CARTESIAN_POINT ( 'NONE',  ( 15.01150461594643204, 17.29947916666666430, 26.00068869287340334 ) ) ;
#2607=CARTESIAN_POINT ( 'NONE',  ( 20.47846945139902530, 42.65663166759063785, 20.53372385742071771 ) ) ;
#2609=CARTESIAN_POINT ( 'NONE',  ( -15.01150461594642138, 46.51822916666666430, -26.00068869287340334 ) ) ;
#2610=CARTESIAN_POINT ( 'NONE',  ( 26.00068869287367335, 65.13802083333334281, 15.01150461594596308 ) ) ;
#2619=CARTESIAN_POINT ( 'NONE',  ( -28.01184896238290278, 21.73958333333332860, 7.505752307973363457 ) ) ;
#2624=CARTESIAN_POINT ( 'NONE',  ( -24.22776226481266448, 37.91888916574269075, -13.94119854578892514 ) ) ;
#2632=CARTESIAN_POINT ( 'NONE',  ( 19.09188309203661049, 57.54687500000000000, -19.09188309203694445 ) ) ;
#2636=CARTESIAN_POINT ( 'NONE',  ( 2.584737979205442066E-13, 38.21093750000000000, 27.95245687107223276 ) ) ;
#2637=CARTESIAN_POINT ( 'NONE',  ( -20.53372385742071771, 29.76600666759063429, 20.47846945139902530 ) ) ;
#2638=CARTESIAN_POINT ( 'NONE',  ( 0.04044903255045854962, 19.58555583240935860, 30.02300923189239867 ) ) ;
#2642=CARTESIAN_POINT ( 'NONE',  ( 6.950374756619257965, 45.51003499907601935, -26.09010956794244507 ) ) ;
#2648=CARTESIAN_POINT ( 'NONE',  ( 26.09010956794232428, 42.08371500092398065, -6.950374756619718042 ) ) ;
#2653=CARTESIAN_POINT ( 'NONE',  ( 30.02300923189239512, 13.28906249999999289, -2.619432448724977703E-13 ) ) ;
#2657=CARTESIAN_POINT ( 'NONE',  ( -20.50609665440969209, 52.39062499999999289, 20.50609665441005092 ) ) ;
#2663=CARTESIAN_POINT ( 'NONE',  ( -28.00173670424535644, 61.55170166574269786, 7.543491769121936308 ) ) ;
#2669=CARTESIAN_POINT ( 'NONE',  ( 26.07999730980477437, 64.70833333333334281, -6.988114217768290004 ) ) ;
#2672=CARTESIAN_POINT ( 'NONE',  ( -2.428612866367529427E-13, 29.61718749999999645, -27.95245687107222921 ) ) ;
#2679=CARTESIAN_POINT ( 'NONE',  ( 27.95245687107223986, 55.97694416759064495, 0.04044903254993640479 ) ) ;
#2689=CARTESIAN_POINT ( 'NONE',  ( 26.09010956794232428, 11.14621500092397532, -6.950374756619718042 ) ) ;
#2693=CARTESIAN_POINT ( 'NONE',  ( -2.584737979205441561E-13, 43.36718749999999289, -30.02300923189239512 ) ) ;
#2697=CARTESIAN_POINT ( 'NONE',  ( -20.50609665441004736, 18.87499999999999645, -20.50609665440969565 ) ) ;
#2703=CARTESIAN_POINT ( 'NONE',  ( 7.543491769121922985, 33.19232666574268364, 28.00173670424535644 ) ) ;
#2705=CARTESIAN_POINT ( 'NONE',  ( 15.01150461594643382, 37.92447916666666430, 26.00068869287340334 ) ) ;
#2710=CARTESIAN_POINT ( 'NONE',  ( -6.950374756619247307, 64.41628499907602645, 26.09010956794245217 ) ) ;
#2714=DIRECTION ( 'NONE',  ( 0.7069718413157916048, 0.01953538259431456675, -0.7069718413158002646 ) ) ;
#2722=CARTESIAN_POINT ( 'NONE',  ( 24.22776226481265383, 15.57513916574268720, 13.94119854578893580 ) ) ;
#2726=CARTESIAN_POINT ( 'NONE',  ( 26.07999730980477437, 44.08333333333332860, -6.988114217768290004 ) ) ;
#2730=CARTESIAN_POINT ( 'NONE',  ( -15.01150461594642138, 19.01822916666666785, -26.00068869287340334 ) ) ;
#2731=CARTESIAN_POINT ( 'NONE',  ( -7.468012846824771955, 10.28684000092397532, -28.02196122052045624 ) ) ;
#2738=CARTESIAN_POINT ( 'NONE',  ( 15.01150461594596308, 64.27864583333332860, -26.00068869287367335 ) ) ;
#2750=CARTESIAN_POINT ( 'NONE',  ( 6.950374756619721595, 25.75559000092397710, 26.09010956794232428 ) ) ;
#2757=CARTESIAN_POINT ( 'NONE',  ( -14.97647472619899389, 43.93451416574269075, 26.02091320914878025 ) ) ;
#2761=CARTESIAN_POINT ( 'NONE',  ( -6.988114217768288228, 15.72395833333332860, -26.07999730980477437 ) ) ;
#2766=CARTESIAN_POINT ( 'NONE',  ( -28.01184896238304134, 18.58854166666666430, -7.505752307972844761 ) ) ;
#2771=CARTESIAN_POINT ( 'NONE',  ( 20.53372385742072481, 38.35975666759064495, -20.47846945139902175 ) ) ;
#2773=CARTESIAN_POINT ( 'NONE',  ( 2.740863092043355209E-13, 51.96093750000000000, 30.02300923189239512 ) ) ;
#2783=CARTESIAN_POINT ( 'NONE',  ( -30.02300923189239867, 25.32031250000000000, 2.654126918244514854E-13 ) ) ;
#2788=CARTESIAN_POINT ( 'NONE',  ( -19.11951029504797006, 34.62461833240934794, -19.06425588902558133 ) ) ;
#2795=CARTESIAN_POINT ( 'NONE',  ( 2.584737979205441561E-13, 55.39843749999999289, 27.95245687107222921 ) ) ;
#2799=CARTESIAN_POINT ( 'NONE',  ( -19.09188309203694445, 39.49999999999999289, -19.09188309203661049 ) ) ;
#2800=CARTESIAN_POINT ( 'NONE',  ( 7.468012846824777284, 32.63059000092395934, 28.02196122052045268 ) ) ;
#2801=CARTESIAN_POINT ( 'NONE',  ( 30.02300923189239867, 15.28868083240935505, -0.04044903255044467877 ) ) ;
#2805=CARTESIAN_POINT ( 'NONE',  ( 26.06988505166722803, 49.52045166574269075, -7.025853678916862854 ) ) ;
#2811=CARTESIAN_POINT ( 'NONE',  ( 7.025853678916403666, 41.51079833425730214, -26.06988505166735237 ) ) ;
#2815=CARTESIAN_POINT ( 'NONE',  ( -28.01184896238290278, 28.61458333333333215, 7.505752307973363457 ) ) ;
#2819=CARTESIAN_POINT ( 'NONE',  ( -30.02300923189239512, 52.82031249999997868, 2.654126918244515359E-13 ) ) ;
#2826=CARTESIAN_POINT ( 'NONE',  ( 26.02091320914876960, 60.26263916574269786, 14.97647472619900455 ) ) ;
#2831=CARTESIAN_POINT ( 'NONE',  ( -19.09188309203694445, 60.12500000000000000, -19.09188309203661049 ) ) ;
#2834=CARTESIAN_POINT ( 'NONE',  ( -24.20753774853730889, 35.34635416666666430, 13.97622843553633842 ) ) ;
#2841=CARTESIAN_POINT ( 'NONE',  ( 24.22776226481241224, 59.12798583425730925, -13.94119854578936923 ) ) ;
#2852=CARTESIAN_POINT ( 'NONE',  ( 7.025853678916403666, 14.01079833425730747, -26.06988505166735237 ) ) ;
#2858=CARTESIAN_POINT ( 'NONE',  ( 7.505752307973351023, 41.50520833333333570, 28.01184896238290278 ) ) ;
#2862=CARTESIAN_POINT ( 'NONE',  ( 7.505752307973351023, 17.44270833333333215, 28.01184896238290278 ) ) ;
#2870=CARTESIAN_POINT ( 'NONE',  ( -28.02196122052058413, 34.33815999907601224, -7.468012846824272799 ) ) ;
#2872=CARTESIAN_POINT ( 'NONE',  ( 28.01184896238290278, 44.08333333333332860, -7.505752307973347470 ) ) ;
#2879=CARTESIAN_POINT ( 'NONE',  ( -0.04044903255042732459, 62.55430583240935505, -27.95245687107223986 ) ) ;
#2886=CARTESIAN_POINT ( 'NONE',  ( -26.07999730980477437, 25.17708333333332860, 6.988114217768305103 ) ) ;
#2893=CARTESIAN_POINT ( 'NONE',  ( 6.950374756619257965, 18.01003499907601935, -26.09010956794244507 ) ) ;
#2897=CARTESIAN_POINT ( 'NONE',  ( 27.95245687107222921, 40.78906249999998579, -2.463307335887066074E-13 ) ) ;
#2901=CARTESIAN_POINT ( 'NONE',  ( -20.50609665440969209, 14.57812499999999645, 20.50609665441005092 ) ) ;
#2902=CARTESIAN_POINT ( 'NONE',  ( 7.543491769121427382, 17.44829833425730925, -28.00173670424548433 ) ) ;
#2923=CARTESIAN_POINT ( 'NONE',  ( -26.09010956794232428, 30.05246500092397000, 6.950374756619732253 ) ) ;
#2931=CARTESIAN_POINT ( 'NONE',  ( -0.04044903255044120238, 48.80430583240936215, -30.02300923189239867 ) ) ;
#2935=CARTESIAN_POINT ( 'NONE',  ( 27.95245687107222921, 13.28906249999999289, -2.463307335887066074E-13 ) ) ;
#2937=CARTESIAN_POINT ( 'NONE',  ( 28.01184896238304134, 20.30729166666666430, 7.505752307972846538 ) ) ;
#2941=CARTESIAN_POINT ( 'NONE',  ( -28.00173670424549499, 37.21392333425730214, -7.543491769121417612 ) ) ;
#2943=CARTESIAN_POINT ( 'NONE',  ( -20.50609665440969209, 52.39062499999999289, 20.50609665441005092 ) ) ;
#2944=CARTESIAN_POINT ( 'NONE',  ( -20.50609665441004736, 67.00000000000000000, -20.50609665440969565 ) ) ;
#2954=CARTESIAN_POINT ( 'NONE',  ( -15.01150461594595775, 21.30989583333332504, 26.00068869287368756 ) ) ;
#2960=CARTESIAN_POINT ( 'NONE',  ( -26.06988505166722803, 34.05170166574267654, 7.025853678916877953 ) ) ;
#2968=CARTESIAN_POINT ( 'NONE',  ( -13.97622843553588901, 62.55989583333332860, 24.20753774853756823 ) ) ;
#2972=CARTESIAN_POINT ( 'NONE',  ( 13.97622843553633842, 41.36197916666665719, 24.20753774853730889 ) ) ;
#2974=CARTESIAN_POINT ( 'NONE',  ( -30.02300923189239867, 30.19569416759064140, -0.04044903254991731589 ) ) ;
#2975=CARTESIAN_POINT ( 'NONE',  ( 15.04653450569339945, 22.73659749907601935, 25.98046417659831775 ) ) ;
#2980=CARTESIAN_POINT ( 'NONE',  ( 26.06988505166722803, 46.08295166574269075, -7.025853678916862854 ) ) ;
#2986=CARTESIAN_POINT ( 'NONE',  ( 27.95245687107223986, 49.10194416759064495, 0.04044903254993640479 ) ) ;
#2990=CARTESIAN_POINT ( 'NONE',  ( -15.01150461594595775, 24.74739583333332504, 26.00068869287368756 ) ) ;
#2993=CARTESIAN_POINT ( 'NONE',  ( -28.01184896238290278, 45.80208333333333570, 7.505752307973363457 ) ) ;
#3000=CARTESIAN_POINT ( 'NONE',  ( -30.02300923189239867, 58.25743083240935505, 0.04044903255044988294 ) ) ;
#3005=CARTESIAN_POINT ( 'NONE',  ( 26.07999730980490227, 61.55729166666666430, 6.988114217767821046 ) ) ;
#3009=CARTESIAN_POINT ( 'NONE',  ( 24.20753774853756113, 30.76302083333332504, 13.97622843553589789 ) ) ;
#3014=CARTESIAN_POINT ( 'NONE',  ( 14.01125832528286352, 58.84152750092397355, -24.18731323226246843 ) ) ;
#3027=CARTESIAN_POINT ( 'NONE',  ( -13.94119854578936923, 23.89361083425731280, -24.22776226481241224 ) ) ;
#3031=EDGE_LOOP ( 'NONE', ( #5870, #24956 ) ) ;
#3032=CARTESIAN_POINT ( 'NONE',  ( -15.01150461594595775, 45.37239583333333570, 26.00068869287368756 ) ) ;
#3036=CARTESIAN_POINT ( 'NONE',  ( 28.01184896238304134, 23.74479166666666430, 7.505752307972846538 ) ) ;
#3043=CARTESIAN_POINT ( 'NONE',  ( -15.04653450569338524, 31.33034749907602290, -25.98046417659831775 ) ) ;
#3045=CARTESIAN_POINT ( 'NONE',  ( 26.00068869287341045, 50.81510416666666430, -15.01150461594642493 ) ) ;
#3051=CARTESIAN_POINT ( 'NONE',  ( -13.94119854578892514, 61.12201416574268364, 24.22776226481266448 ) ) ;
#3057=CARTESIAN_POINT ( 'NONE',  ( 13.97622843553633842, 20.73697916666666075, 24.20753774853730889 ) ) ;
#3066=CARTESIAN_POINT ( 'NONE',  ( 14.01125832528330051, 26.17409749907601935, 24.18731323226221974 ) ) ;
#3069=CARTESIAN_POINT ( 'NONE',  ( 6.988114217768294445, 48.38020833333332860, 26.07999730980477437 ) ) ;
#3074=CARTESIAN_POINT ( 'NONE',  ( -2.584737979205441561E-13, 12.42968749999999289, -30.02300923189239512 ) ) ;
#3075=CARTESIAN_POINT ( 'NONE',  ( -0.04044903254990864921, 19.02381916759064495, 30.02300923189239867 ) ) ;
#3097=CARTESIAN_POINT ( 'NONE',  ( 19.06425588902592239, 28.90663166759063785, 19.11951029504763611 ) ) ;
#3105=CARTESIAN_POINT ( 'NONE',  ( 30.02300923189239867, 46.22618083240936215, -0.04044903255044467877 ) ) ;
#3109=CARTESIAN_POINT ( 'NONE',  ( 24.20753774853731244, 16.44010416666666430, -13.97622843553632599 ) ) ;
#3111=CARTESIAN_POINT ( 'NONE',  ( 26.00068869287340334, 19.87760416666666430, -15.01150461594642316 ) ) ;
#3114=CARTESIAN_POINT ( 'NONE',  ( 28.02196122052045268, 38.64621500092395934, -7.468012846824774620 ) ) ;
#3116=CARTESIAN_POINT ( 'NONE',  ( 2.740863092043355209E-13, 48.52343750000000000, 30.02300923189239512 ) ) ;
#3125=CARTESIAN_POINT ( 'NONE',  ( 20.50609665441005092, 17.15624999999999645, 20.50609665440969209 ) ) ;
#3137=CARTESIAN_POINT ( 'NONE',  ( 13.97622843553589966, 64.27864583333332860, -24.20753774853756113 ) ) ;
#3141=CARTESIAN_POINT ( 'NONE',  ( -24.20753774853730889, 42.22135416666666430, 13.97622843553634020 ) ) ;
#3142=CARTESIAN_POINT ( 'NONE',  ( -7.468012846824771955, 30.91184000092396644, -28.02196122052045624 ) ) ;
#3144=CARTESIAN_POINT ( 'NONE',  ( 28.00173670424535644, 18.58295166574268364, -7.543491769121920321 ) ) ;
#3148=CARTESIAN_POINT ( 'NONE',  ( 13.94119854578893580, 49.09076416574269786, -24.22776226481265383 ) ) ;
#3155=CARTESIAN_POINT ( 'NONE',  ( -26.06988505166735237, 54.40142333425730925, -7.025853678916388567 ) ) ;
#3160=CARTESIAN_POINT ( 'NONE',  ( 26.00068869287367335, 20.45052083333332504, 15.01150461594596308 ) ) ;
#3164=CARTESIAN_POINT ( 'NONE',  ( -15.01150461594642138, 49.95572916666665009, -26.00068869287340334 ) ) ;
#3171=CARTESIAN_POINT ( 'NONE',  ( 15.04653450569339945, 63.98659749907601935, 25.98046417659831775 ) ) ;
#3176=CARTESIAN_POINT ( 'NONE',  ( -26.07999730980477437, 62.98958333333332149, 6.988114217768305103 ) ) ;
#3179=CARTESIAN_POINT ( 'NONE',  ( 19.09188309203661049, 30.04687500000000000, -19.09188309203694445 ) ) ;
#3184=CARTESIAN_POINT ( 'NONE',  ( 24.18731323226247554, 59.70090250092397355, 14.01125832528285997 ) ) ;
#3197=CARTESIAN_POINT ( 'NONE',  ( -27.95245687107223986, 19.88319416759064495, -0.04044903254993292840 ) ) ;
#3203=CARTESIAN_POINT ( 'NONE',  ( 20.50609665441005092, 48.09375000000000000, 20.50609665440969209 ) ) ;
#3207=CARTESIAN_POINT ( 'NONE',  ( 26.00068869287367335, 20.45052083333332504, 15.01150461594596308 ) ) ;
#3213=CARTESIAN_POINT ( 'NONE',  ( 20.53372385742108008, 32.90586833240934794, 20.47846945139866648 ) ) ;
#3215=CARTESIAN_POINT ( 'NONE',  ( 20.50609665440969565, 47.23437499999999289, -20.50609665441004736 ) ) ;
#3218=CARTESIAN_POINT ( 'NONE',  ( 13.94119854578893580, 59.40326416574269075, -24.22776226481265383 ) ) ;
#3224=CARTESIAN_POINT ( 'NONE',  ( -6.988114217767819270, 21.16666666666666430, 26.07999730980490583 ) ) ;
#3231=CARTESIAN_POINT ( 'NONE',  ( 19.11951029504797006, 26.03086833240935860, 19.06425588902558133 ) ) ;
#3234=CARTESIAN_POINT ( 'NONE',  ( -26.07999730980477437, 52.67708333333333570, 6.988114217768305103 ) ) ;
#3238=CARTESIAN_POINT ( 'NONE',  ( 15.01150461594643204, 27.61197916666666430, 26.00068869287340334 ) ) ;
#3239=CARTESIAN_POINT ( 'NONE',  ( 28.02196122052045268, 28.33371500092397355, -7.468012846824774620 ) ) ;
#3258=CARTESIAN_POINT ( 'NONE',  ( 26.09010956794232428, 42.08371500092398065, -6.950374756619718042 ) ) ;
#3265=CARTESIAN_POINT ( 'NONE',  ( -15.04653450569338524, 55.39284749907604066, -25.98046417659831775 ) ) ;
#3269=CARTESIAN_POINT ( 'NONE',  ( 24.20753774853731244, 26.75260416666666430, -13.97622843553632599 ) ) ;
#3272=CARTESIAN_POINT ( 'NONE',  ( 15.01150461594643204, 34.48697916666667140, 26.00068869287340334 ) ) ;
#3275=CARTESIAN_POINT ( 'NONE',  ( 7.543491769121427382, 38.07329833425730925, -28.00173670424548433 ) ) ;
#3278=CARTESIAN_POINT ( 'NONE',  ( -15.01150461594595775, 55.68489583333332860, 26.00068869287368756 ) ) ;
#3279=CARTESIAN_POINT ( 'NONE',  ( -7.505752307972844761, 65.85416666666665719, 28.01184896238304134 ) ) ;
#3301=CARTESIAN_POINT ( 'NONE',  ( -24.18731323226248264, 13.29465250092397532, -14.01125832528284931 ) ) ;
#3306=CARTESIAN_POINT ( 'NONE',  ( 2.584737979205442066E-13, 48.52343749999999289, 27.95245687107223276 ) ) ;
#3308=CARTESIAN_POINT ( 'NONE',  ( -15.04653450569291984, 26.18527750092397710, 25.98046417659859486 ) ) ;
#3309=CARTESIAN_POINT ( 'NONE',  ( -26.02091320914878025, 31.04388916574268364, -14.97647472619899389 ) ) ;
#3313=CARTESIAN_POINT ( 'NONE',  ( 7.025853678916867295, 43.50482666574268364, 26.06988505166722803 ) ) ;
#3319=CARTESIAN_POINT ( 'NONE',  ( -7.025853678916393008, 50.10454833425731636, 26.06988505166735592 ) ) ;
#3323=CARTESIAN_POINT ( 'NONE',  ( -20.50609665440969209, 21.45312499999999645, 20.50609665441005092 ) ) ;
#3327=CARTESIAN_POINT ( 'NONE',  ( -28.01184896238290278, 56.11458333333332860, 7.505752307973363457 ) ) ;
#3332=CARTESIAN_POINT ( 'NONE',  ( -27.95245687107223986, 17.00743083240935860, 0.04044903255043252877 ) ) ;
#3339=CARTESIAN_POINT ( 'NONE',  ( -6.988114217768288228, 29.47395833333332860, -26.07999730980477437 ) ) ;
#3347=CARTESIAN_POINT ( 'NONE',  ( 19.11951029504763611, 55.54725666759064495, -19.06425588902591173 ) ) ;
#3359=CARTESIAN_POINT ( 'NONE',  ( -26.09010956794232428, 19.73996500092397355, 6.950374756619732253 ) ) ;
#3364=CARTESIAN_POINT ( 'NONE',  ( -7.505752307972844761, 52.10416666666666430, 28.01184896238304134 ) ) ;
#3368=CARTESIAN_POINT ( 'NONE',  ( -28.01184896238304134, 22.02604166666666430, -7.505752307972844761 ) ) ;
#3374=CARTESIAN_POINT ( 'NONE',  ( -20.47846945139866648, 47.51524333240936215, 20.53372385742108008 ) ) ;
#3377=CARTESIAN_POINT ( 'NONE',  ( -26.00068869287340334, 45.65885416666666430, 15.01150461594643559 ) ) ;
#3380=CARTESIAN_POINT ( 'NONE',  ( 0.04044903255044120238, 57.39805583240935505, 27.95245687107223276 ) ) ;
#3381=ADVANCED_FACE ( 'NONE', ( #15366 ), #7797, .T. ) ;
#3388=CARTESIAN_POINT ( 'NONE',  ( 13.97622843553633842, 24.17447916666666075, 24.20753774853730889 ) ) ;
#3395=CARTESIAN_POINT ( 'NONE',  ( -19.11951029504797006, 24.31211833240934794, -19.06425588902558133 ) ) ;
#3399=CARTESIAN_POINT ( 'NONE',  ( 6.988114217767829928, 57.26041666666666430, -26.07999730980489872 ) ) ;
#3403=CARTESIAN_POINT ( 'NONE',  ( 15.01150461594596308, 23.02864583333332149, -26.00068869287367335 ) ) ;
#3404=CARTESIAN_POINT ( 'NONE',  ( -28.02196122052045268, 19.73996500092397355, 7.468012846824790607 ) ) ;
#3423=CARTESIAN_POINT ( 'NONE',  ( -26.09010956794232428, 43.80246500092398776, 6.950374756619732253 ) ) ;
#3430=CARTESIAN_POINT ( 'NONE',  ( 30.02300923189239867, 59.97618083240934794, -0.04044903255044467877 ) ) ;
#3435=CARTESIAN_POINT ( 'NONE',  ( 24.20753774853731244, 23.31510416666666430, -13.97622843553632599 ) ) ;
#3439=CARTESIAN_POINT ( 'NONE',  ( 15.01150461594643204, 27.61197916666666430, 26.00068869287340334 ) ) ;
#3442=CARTESIAN_POINT ( 'NONE',  ( -30.02300923189239867, 47.38319416759065206, -0.04044903254991731589 ) ) ;
#3444=CARTESIAN_POINT ( 'NONE',  ( 26.00068869287340334, 54.25260416666666430, -15.01150461594642316 ) ) ;
#3464=CARTESIAN_POINT ( 'NONE',  ( 6.950374756619721595, 15.44309000092397355, 26.09010956794232428 ) ) ;
#3469=CARTESIAN_POINT ( 'NONE',  ( -24.20753774853730889, 49.09635416666666430, 13.97622843553634020 ) ) ;
#3470=CARTESIAN_POINT ( 'NONE',  ( -20.53372385742071771, 40.07850666759064495, 20.47846945139902530 ) ) ;
#3471=CARTESIAN_POINT ( 'NONE',  ( 7.468012846824281681, 31.76003499907602290, -28.02196122052058058 ) ) ;
#3474=CARTESIAN_POINT ( 'NONE',  ( 14.01125832528330051, 57.11159749907603356, 24.18731323226221974 ) ) ;
#3480=CARTESIAN_POINT ( 'NONE',  ( 19.11951029504763611, 55.54725666759064495, -19.06425588902591173 ) ) ;
#3484=AXIS2_PLACEMENT_3D ( 'NONE', #33078, #25029, #2030 ) ;
#3486=CARTESIAN_POINT ( 'NONE',  ( 26.00068869287340334, 26.75260416666666430, -15.01150461594642316 ) ) ;
#3490=CARTESIAN_POINT ( 'NONE',  ( 30.02300923189239512, 54.53906249999998579, -2.619432448724977703E-13 ) ) ;
#3496=CARTESIAN_POINT ( 'NONE',  ( 19.11951029504797006, 15.71836833240935327, 19.06425588902558133 ) ) ;
#3503=CARTESIAN_POINT ( 'NONE',  ( -24.20753774853730889, 45.65885416666666430, 13.97622843553633842 ) ) ;
#3509=CARTESIAN_POINT ( 'NONE',  ( 30.02300923189239867, 11.28944416759064140, 0.04044903254992252006 ) ) ;
#3511=CARTESIAN_POINT ( 'NONE',  ( -26.00068869287368756, 56.54427083333332149, -15.01150461594595775 ) ) ;
#3522=CARTESIAN_POINT ( 'NONE',  ( 27.95245687107223986, 21.60194416759064495, 0.04044903254993640479 ) ) ;
#3527=CARTESIAN_POINT ( 'NONE',  ( -15.01150461594642138, 53.39322916666665009, -26.00068869287340334 ) ) ;
#3531=CARTESIAN_POINT ( 'NONE',  ( -30.02300923189239512, 32.19531250000000000, 2.654126918244515359E-13 ) ) ;
#3537=CARTESIAN_POINT ( 'NONE',  ( -25.98046417659831420, 44.22097249907603356, 15.04653450569339945 ) ) ;
#3539=CARTESIAN_POINT ( 'NONE',  ( -15.01150461594595775, 52.24739583333332860, 26.00068869287368756 ) ) ;
#3542=CARTESIAN_POINT ( 'NONE',  ( 26.09010956794244507, 66.99440999907601224, 6.950374756619249084 ) ) ;
#3548=CARTESIAN_POINT ( 'NONE',  ( -19.09188309203694445, 18.87499999999999645, -19.09188309203661049 ) ) ;
#3555=CARTESIAN_POINT ( 'NONE',  ( 14.01125832528330051, 29.61159749907602290, 24.18731323226221974 ) ) ;
#3560=CARTESIAN_POINT ( 'NONE',  ( -2.428612866367529427E-13, 53.67968750000000000, -27.95245687107222921 ) ) ;
#3566=CARTESIAN_POINT ( 'NONE',  ( 2.740863092043355209E-13, 24.46093749999999645, 30.02300923189239512 ) ) ;
#3567=CARTESIAN_POINT ( 'NONE',  ( -25.98046417659859486, 20.16965250092397355, -15.04653450569291628 ) ) ;
#3577=CARTESIAN_POINT ( 'NONE',  ( 26.02091320914851025, 59.12798583425730925, -14.97647472619946463 ) ) ;
#3583=CARTESIAN_POINT ( 'NONE',  ( -24.18731323226221974, 33.90847249907601935, 14.01125832528330406 ) ) ;
#3588=CARTESIAN_POINT ( 'NONE',  ( 26.09010956794232428, 38.64621500092395934, -6.950374756619718042 ) ) ;
#3595=CARTESIAN_POINT ( 'NONE',  ( 20.53372385742108008, 56.96836833240936215, 20.47846945139866648 ) ) ;
#3600=CARTESIAN_POINT ( 'NONE',  ( 26.07999730980490227, 23.74479166666666430, 6.988114217767821046 ) ) ;
#3603=CARTESIAN_POINT ( 'NONE',  ( 26.00068869287367335, 30.76302083333332504, 15.01150461594596308 ) ) ;
#3607=CARTESIAN_POINT ( 'NONE',  ( 7.543491769121427382, 51.82329833425730925, -28.00173670424548433 ) ) ;
#3610=CARTESIAN_POINT ( 'NONE',  ( -30.02300923189239512, 59.69531250000000711, 2.654126918244515359E-13 ) ) ;
#3630=CARTESIAN_POINT ( 'NONE',  ( 0.04044903254993986036, 10.43006916759064495, -27.95245687107223986 ) ) ;
#3635=CARTESIAN_POINT ( 'NONE',  ( -19.09188309203660694, 45.51562500000000000, 19.09188309203694800 ) ) ;
#3636=CARTESIAN_POINT ( 'NONE',  ( -7.543491769121417612, 39.79204833425731636, 28.00173670424549499 ) ) ;
#3637=CARTESIAN_POINT ( 'NONE',  ( 7.543491769121922985, 29.75482666574269075, 28.00173670424535644 ) ) ;
#3640=CARTESIAN_POINT ( 'NONE',  ( 13.94119854578893580, 55.96576416574269786, -24.22776226481265383 ) ) ;
#3645=CARTESIAN_POINT ( 'NONE',  ( 14.01125832528286352, 55.40402750092397355, -24.18731323226246843 ) ) ;
#3649=CARTESIAN_POINT ( 'NONE',  ( 7.505752307972854531, 29.76041666666666430, -28.01184896238303423 ) ) ;
#3653=CARTESIAN_POINT ( 'NONE',  ( 15.01150461594643204, 58.54947916666665009, 26.00068869287340334 ) ) ;
#3661=CARTESIAN_POINT ( 'NONE',  ( -25.98046417659831420, 68.28347249907602645, 15.04653450569339945 ) ) ;
#3670=CARTESIAN_POINT ( 'NONE',  ( -27.95245687107222921, 45.94531249999997868, 2.498001805406602216E-13 ) ) ;
#3676=CARTESIAN_POINT ( 'NONE',  ( 24.22776226481241224, 62.56548583425730925, -13.94119854578936923 ) ) ;
#3677=CARTESIAN_POINT ( 'NONE',  ( -7.505752307972844761, 52.10416666666666430, 28.01184896238304134 ) ) ;
#3688=CARTESIAN_POINT ( 'NONE',  ( 0.04044903254993986036, 27.61756916759064140, -27.95245687107223986 ) ) ;
#3694=CARTESIAN_POINT ( 'NONE',  ( -7.505752307972844761, 55.54166666666667140, 28.01184896238304134 ) ) ;
#3698=CARTESIAN_POINT ( 'NONE',  ( -7.505752307972844761, 31.47916666666666075, 28.01184896238304134 ) ) ;
#3704=CARTESIAN_POINT ( 'NONE',  ( -26.02091320914878025, 48.23138916574269786, -14.97647472619899389 ) ) ;
#3706=CARTESIAN_POINT ( 'NONE',  ( -28.01184896238304134, 52.96354166666666430, -7.505752307972844761 ) ) ;
#3711=CARTESIAN_POINT ( 'NONE',  ( -19.09188309203660694, 14.57812499999999645, 19.09188309203694800 ) ) ;
#3717=CARTESIAN_POINT ( 'NONE',  ( 13.97622843553633842, 34.48697916666666430, 24.20753774853730889 ) ) ;
#3724=CARTESIAN_POINT ( 'NONE',  ( 20.53372385742108008, 26.03086833240935860, 20.47846945139866648 ) ) ;
#3726=CARTESIAN_POINT ( 'NONE',  ( -13.94119854578892514, 30.18451416574268720, 24.22776226481266448 ) ) ;
#3730=CARTESIAN_POINT ( 'NONE',  ( 26.07999730980477437, 50.95833333333332860, -6.988114217768290004 ) ) ;
#3735=CARTESIAN_POINT ( 'NONE',  ( 20.50609665441005092, 27.46875000000000000, 20.50609665440969209 ) ) ;
#3736=CARTESIAN_POINT ( 'NONE',  ( -28.00173670424549499, 26.90142333425731280, -7.543491769121417612 ) ) ;
#3744=CARTESIAN_POINT ( 'NONE',  ( 0.04044903254992426173, 55.11756916759064495, -30.02300923189239867 ) ) ;
#3746=CARTESIAN_POINT ( 'NONE',  ( -28.01184896238290278, 25.17708333333332860, 7.505752307973363457 ) ) ;
#3750=CARTESIAN_POINT ( 'NONE',  ( -6.950374756619247307, 47.22878499907602645, 26.09010956794245217 ) ) ;
#3756=CARTESIAN_POINT ( 'NONE',  ( -13.94119854578936923, 37.64361083425730925, -24.22776226481241224 ) ) ;
#3766=CARTESIAN_POINT ( 'NONE',  ( -28.00173670424535644, 54.67670166574269075, 7.543491769121936308 ) ) ;
#3769=CARTESIAN_POINT ( 'NONE',  ( 26.07999730980477437, 23.45833333333333215, -6.988114217768290004 ) ) ;
#3772=CARTESIAN_POINT ( 'NONE',  ( -2.584737979205441561E-13, 29.61718749999999645, -30.02300923189239512 ) ) ;
#3775=CARTESIAN_POINT ( 'NONE',  ( -15.04653450569291984, 50.24777750092398065, 25.98046417659859486 ) ) ;
#3777=CARTESIAN_POINT ( 'NONE',  ( -7.505752307972844761, 62.41666666666666430, 28.01184896238304134 ) ) ;
#3796=CARTESIAN_POINT ( 'NONE',  ( -26.07999730980490583, 66.71354166666665719, -6.988114217767815717 ) ) ;
#3802=CARTESIAN_POINT ( 'NONE',  ( 6.988114217767829928, 50.38541666666666430, -26.07999730980489872 ) ) ;
#3803=CARTESIAN_POINT ( 'NONE',  ( -7.468012846824771955, 37.78684000092396644, -28.02196122052045624 ) ) ;
#3805=CARTESIAN_POINT ( 'NONE',  ( 14.97647472619900455, 28.46576416574268720, -26.02091320914876960 ) ) ;
#3808=CARTESIAN_POINT ( 'NONE',  ( 24.18731323226221974, 52.81472249907603356, -14.01125832528328985 ) ) ;
#3816=CARTESIAN_POINT ( 'NONE',  ( 7.505752307972854531, 33.19791666666665719, -28.01184896238303423 ) ) ;
#3820=CARTESIAN_POINT ( 'NONE',  ( -20.50609665440969209, 59.26562500000000000, 20.50609665441005092 ) ) ;
#3827=CARTESIAN_POINT ( 'NONE',  ( -19.11951029504797006, 17.43711833240935505, -19.06425588902558133 ) ) ;
#3835=CARTESIAN_POINT ( 'NONE',  ( 24.20753774853731244, 37.06510416666666430, -13.97622843553632599 ) ) ;
#3840=CARTESIAN_POINT ( 'NONE',  ( 26.06988505166735592, 62.99517333425730214, 7.025853678916393896 ) ) ;
#3841=CARTESIAN_POINT ( 'NONE',  ( -28.01184896238304134, 52.96354166666666430, -7.505752307972844761 ) ) ;
#3852=CARTESIAN_POINT ( 'NONE',  ( 26.06988505166735592, 35.49517333425730214, 7.025853678916393896 ) ) ;
#3860=CARTESIAN_POINT ( 'NONE',  ( 7.505752307973351023, 48.38020833333332860, 28.01184896238290278 ) ) ;
#3864=CARTESIAN_POINT ( 'NONE',  ( 26.00068869287367335, 30.76302083333332504, 15.01150461594596308 ) ) ;
#3869=CARTESIAN_POINT ( 'NONE',  ( 0.04044903255045854962, 43.64805583240936215, 30.02300923189239867 ) ) ;
#3871=CARTESIAN_POINT ( 'NONE',  ( -2.584737979205442066E-13, 53.67968750000000000, -30.02300923189239867 ) ) ;
#3875=CARTESIAN_POINT ( 'NONE',  ( 2.584737979205441561E-13, 14.14843749999999289, 27.95245687107222921 ) ) ;
#3881=CARTESIAN_POINT ( 'NONE',  ( -26.07999730980477437, 35.48958333333332860, 6.988114217768305103 ) ) ;
#3886=CARTESIAN_POINT ( 'NONE',  ( -0.04044903255044120238, 21.30430583240935860, -30.02300923189239867 ) ) ;
#3889=CARTESIAN_POINT ( 'NONE',  ( -24.22776226481266448, 41.35638916574269075, -13.94119854578892514 ) ) ;
#3893=CARTESIAN_POINT ( 'NONE',  ( 24.20753774853731244, 57.69010416666667140, -13.97622843553632599 ) ) ;
#3899=CARTESIAN_POINT ( 'NONE',  ( 15.01150461594643204, 20.73697916666666075, 26.00068869287340334 ) ) ;
#3900=CARTESIAN_POINT ( 'NONE',  ( -28.00173670424549499, 20.02642333425731280, -7.543491769121417612 ) ) ;
#3910=CARTESIAN_POINT ( 'NONE',  ( -25.98046417659859486, 57.98215250092397355, -15.04653450569291628 ) ) ;
#3913=CARTESIAN_POINT ( 'NONE',  ( 28.01184896238304134, 30.61979166666666075, 7.505752307972846538 ) ) ;
#3917=CARTESIAN_POINT ( 'NONE',  ( -14.01125832528328985, 45.08034749907603356, -24.18731323226223040 ) ) ;
#3923=CARTESIAN_POINT ( 'NONE',  ( 24.22776226481241224, 35.06548583425731636, -13.94119854578936923 ) ) ;
#3931=CARTESIAN_POINT ( 'NONE',  ( -25.98046417659831420, 54.53347249907601935, 15.04653450569339945 ) ) ;
#3935=CARTESIAN_POINT ( 'NONE',  ( 24.20753774853731244, 30.19010416666665719, -13.97622843553632599 ) ) ;
#3938=CARTESIAN_POINT ( 'NONE',  ( -20.50609665441004736, 32.62500000000000000, -20.50609665440969565 ) ) ;
#3941=CARTESIAN_POINT ( 'NONE',  ( -28.00173670424549499, 54.40142333425730925, -7.543491769121417612 ) ) ;
#3943=CARTESIAN_POINT ( 'NONE',  ( 30.02300923189239512, 64.85156249999998579, -2.619432448724977703E-13 ) ) ;
#3962=CARTESIAN_POINT ( 'NONE',  ( 24.22776226481241224, 14.44048583425730925, -13.94119854578936923 ) ) ;
#3968=CARTESIAN_POINT ( 'NONE',  ( 24.20753774853756113, 51.38802083333332860, 13.97622843553589789 ) ) ;
#3969=CARTESIAN_POINT ( 'NONE',  ( -14.97647472619946285, 37.64361083425730925, -26.02091320914851025 ) ) ;
#3971=CARTESIAN_POINT ( 'NONE',  ( -14.97647472619899389, 30.18451416574268720, 26.02091320914878025 ) ) ;
#3974=CARTESIAN_POINT ( 'NONE',  ( -24.22776226481266448, 58.54388916574269075, -13.94119854578892514 ) ) ;
#3982=CARTESIAN_POINT ( 'NONE',  ( 20.50609665440969565, 33.48437500000000000, -20.50609665441004736 ) ) ;
#3987=CARTESIAN_POINT ( 'NONE',  ( -2.584737979205441561E-13, 60.55468749999999289, -30.02300923189239512 ) ) ;
#3995=CARTESIAN_POINT ( 'NONE',  ( -26.06988505166722803, 16.86420166574268720, 7.025853678916877953 ) ) ;
#4003=CARTESIAN_POINT ( 'NONE',  ( -24.20753774853756823, 42.79427083333331439, -13.97622843553588723 ) ) ;
#4008=CARTESIAN_POINT ( 'NONE',  ( -28.02196122052045268, 12.86496500092397710, 7.468012846824790607 ) ) ;
#4009=CARTESIAN_POINT ( 'NONE',  ( -26.00068869287340334, 55.97135416666665719, 15.01150461594643382 ) ) ;
#4020=CARTESIAN_POINT ( 'NONE',  ( 0.04044903254993986036, 31.05506916759064495, -27.95245687107223986 ) ) ;
#4025=CARTESIAN_POINT ( 'NONE',  ( 15.01150461594643204, 58.54947916666665009, 26.00068869287340334 ) ) ;
#4029=CARTESIAN_POINT ( 'NONE',  ( 15.01150461594596308, 33.34114583333332860, -26.00068869287367335 ) ) ;
#4034=CARTESIAN_POINT ( 'NONE',  ( -28.02196122052058413, 41.21315999907602645, -7.468012846824272799 ) ) ;
#4036=CARTESIAN_POINT ( 'NONE',  ( 7.505752307973351023, 55.25520833333333570, 28.01184896238290278 ) ) ;
#4041=CARTESIAN_POINT ( 'NONE',  ( -13.97622843553632421, 15.58072916666666607, -24.20753774853731599 ) ) ;
#4051=CARTESIAN_POINT ( 'NONE',  ( -0.04044903255044120238, 24.74180583240935505, -30.02300923189239867 ) ) ;
#4054=CARTESIAN_POINT ( 'NONE',  ( 7.025853678916867295, 36.62982666574267654, 26.06988505166722803 ) ) ;
#4060=CARTESIAN_POINT ( 'NONE',  ( 6.988114217768294445, 62.13020833333334281, 26.07999730980477437 ) ) ;
#4065=CARTESIAN_POINT ( 'NONE',  ( 26.00068869287367335, 37.63802083333331439, 15.01150461594596308 ) ) ;
#4066=CARTESIAN_POINT ( 'NONE',  ( 25.98046417659858420, 35.63840250092398065, 15.04653450569292872 ) ) ;
#4075=CARTESIAN_POINT ( 'NONE',  ( -28.02196122052045268, 57.55246500092398065, 7.468012846824790607 ) ) ;
#4078=CARTESIAN_POINT ( 'NONE',  ( -15.01150461594595775, 35.05989583333332860, 26.00068869287368756 ) ) ;
#4084=CARTESIAN_POINT ( 'NONE',  ( -24.22776226481266448, 41.35638916574269075, -13.94119854578892514 ) ) ;
#4090=CARTESIAN_POINT ( 'NONE',  ( 24.22776226481241224, 48.81548583425731636, -13.94119854578936923 ) ) ;
#4097=CARTESIAN_POINT ( 'NONE',  ( -30.02300923189239867, 65.13243083240935505, 0.04044903255044988294 ) ) ;
#4102=CARTESIAN_POINT ( 'NONE',  ( -19.09188309203694445, 32.62500000000000000, -19.09188309203661049 ) ) ;
#4105=CARTESIAN_POINT ( 'NONE',  ( -2.584737979205441561E-13, 43.36718749999999289, -30.02300923189239512 ) ) ;
#4109=CARTESIAN_POINT ( 'NONE',  ( 20.53372385742072481, 48.67225666759065206, -20.47846945139902175 ) ) ;
#4111=CARTESIAN_POINT ( 'NONE',  ( 7.505752307973351023, 65.56770833333332860, 28.01184896238290278 ) ) ;
#4132=CARTESIAN_POINT ( 'NONE',  ( 0.04044903254993986036, 17.30506916759064140, -27.95245687107223986 ) ) ;
#4137=CARTESIAN_POINT ( 'NONE',  ( -6.988114217767819270, 55.54166666666667140, 26.07999730980490583 ) ) ;
#4138=CARTESIAN_POINT ( 'NONE',  ( 28.02196122052045268, 42.08371500092398065, -7.468012846824774620 ) ) ;
#4139=CARTESIAN_POINT ( 'NONE',  ( 20.47846945139867003, 38.92149333240934794, -20.53372385742107653 ) ) ;
#4143=CARTESIAN_POINT ( 'NONE',  ( -14.01125832528328985, 55.39284749907604066, -24.18731323226223040 ) ) ;
#4152=CARTESIAN_POINT ( 'NONE',  ( -7.505752307972844761, 31.47916666666666075, 28.01184896238304134 ) ) ;
#4167=CARTESIAN_POINT ( 'NONE',  ( -14.01125832528328985, 24.45534749907602290, -24.18731323226223040 ) ) ;
#4175=CARTESIAN_POINT ( 'NONE',  ( -26.07999730980490583, 42.65104166666666430, -6.988114217767815717 ) ) ;
#4180=CARTESIAN_POINT ( 'NONE',  ( -0.04044903254990864921, 15.58631916759064495, 30.02300923189239867 ) ) ;
#4181=CARTESIAN_POINT ( 'NONE',  ( 2.740863092043355209E-13, 51.96093750000000000, 30.02300923189239512 ) ) ;
#4192=CARTESIAN_POINT ( 'NONE',  ( 26.06988505166735592, 32.05767333425730214, 7.025853678916393896 ) ) ;
#4198=CARTESIAN_POINT ( 'NONE',  ( -20.50609665440969209, 62.70312500000000000, 20.50609665441005092 ) ) ;
#4201=CARTESIAN_POINT ( 'NONE',  ( -28.01184896238290278, 28.61458333333333215, 7.505752307973363457 ) ) ;
#4206=CARTESIAN_POINT ( 'NONE',  ( -28.00173670424535644, 54.67670166574269075, 7.543491769121936308 ) ) ;
#4208=CARTESIAN_POINT ( 'NONE',  ( 28.01184896238304134, 54.68229166666665719, 7.505752307972846538 ) ) ;
#4213=CARTESIAN_POINT ( 'NONE',  ( -27.95245687107222921, 15.00781249999999467, 2.498001805406602216E-13 ) ) ;
#4224=CARTESIAN_POINT ( 'NONE',  ( -28.02196122052058413, 24.02565999907602290, -7.468012846824272799 ) ) ;
#4227=CARTESIAN_POINT ( 'NONE',  ( 14.01125832528330051, 36.48659749907601935, 24.18731323226221974 ) ) ;
#4230=CARTESIAN_POINT ( 'NONE',  ( -24.20753774853756823, 66.85677083333334281, -13.97622843553588723 ) ) ;
#4235=CARTESIAN_POINT ( 'NONE',  ( 30.02300923189239512, 33.91406249999997158, -2.619432448724977703E-13 ) ) ;
#4236=CARTESIAN_POINT ( 'NONE',  ( -20.53372385742071771, 33.20350666759063074, 20.47846945139902530 ) ) ;
#4245=CARTESIAN_POINT ( 'NONE',  ( 20.53372385742072481, 52.10975666759065206, -20.47846945139902175 ) ) ;
#4248=CARTESIAN_POINT ( 'NONE',  ( 20.50609665440969565, 33.48437500000000000, -20.50609665441004736 ) ) ;
#4252=CARTESIAN_POINT ( 'NONE',  ( 19.06425588902558133, 45.79649333240935505, -19.11951029504797006 ) ) ;
#4259=CARTESIAN_POINT ( 'NONE',  ( -26.09010956794232428, 47.23996500092398065, 6.950374756619732253 ) ) ;
#4266=CARTESIAN_POINT ( 'NONE',  ( 7.468012846824281681, 66.13503499907601224, -28.02196122052058058 ) ) ;
#4271=CARTESIAN_POINT ( 'NONE',  ( 13.97622843553633665, 37.92447916666666430, 24.20753774853730889 ) ) ;
#4274=CARTESIAN_POINT ( 'NONE',  ( 28.01184896238304134, 44.36979166666666430, 7.505752307972846538 ) ) ;
#4277=CARTESIAN_POINT ( 'NONE',  ( -14.97647472619946285, 58.26861083425732346, -26.02091320914851025 ) ) ;
#4278=CARTESIAN_POINT ( 'NONE',  ( -26.06988505166735237, 64.71392333425730214, -7.025853678916388567 ) ) ;
#4280=CARTESIAN_POINT ( 'NONE',  ( 2.740863092043355209E-13, 62.27343749999999289, 30.02300923189239512 ) ) ;
#4299=CARTESIAN_POINT ( 'NONE',  ( -26.06988505166735237, 16.58892333425730570, -7.025853678916388567 ) ) ;
#4304=CARTESIAN_POINT ( 'NONE',  ( -7.543491769121417612, 46.66704833425730925, 28.00173670424549499 ) ) ;
#4305=CARTESIAN_POINT ( 'NONE',  ( 30.02300923189239867, 39.35118083240935505, -0.04044903255044467877 ) ) ;
#4308=CARTESIAN_POINT ( 'NONE',  ( -7.025853678916861966, 65.84857666574268364, -26.06988505166722803 ) ) ;
#4320=CARTESIAN_POINT ( 'NONE',  ( 7.505752307973351023, 34.63020833333332860, 28.01184896238290278 ) ) ;
#4326=CARTESIAN_POINT ( 'NONE',  ( -28.01184896238290278, 62.98958333333332149, 7.505752307973363457 ) ) ;
#4330=CARTESIAN_POINT ( 'NONE',  ( -2.584737979205442066E-13, 12.42968749999999822, -30.02300923189239867 ) ) ;
#4335=CARTESIAN_POINT ( 'NONE',  ( 7.025853678916867295, 22.87982666574268720, 26.06988505166722803 ) ) ;
#4342=CARTESIAN_POINT ( 'NONE',  ( -26.07999730980490583, 46.08854166666666430, -6.988114217767815717 ) ) ;
#4347=CARTESIAN_POINT ( 'NONE',  ( 0.04044903254992426173, 20.74256916759064495, -30.02300923189239867 ) ) ;
#4348=CARTESIAN_POINT ( 'NONE',  ( -20.50609665440969209, 66.14062500000000000, 20.50609665441005092 ) ) ;
#4355=CARTESIAN_POINT ( 'NONE',  ( -13.97622843553588901, 65.99739583333332860, 24.20753774853756823 ) ) ;
#4361=CARTESIAN_POINT ( 'NONE',  ( 26.09010956794232428, 31.77121500092397000, -6.950374756619718042 ) ) ;
#4368=CARTESIAN_POINT ( 'NONE',  ( -30.02300923189239512, 42.50781249999997868, 2.654126918244515359E-13 ) ) ;
#4374=CARTESIAN_POINT ( 'NONE',  ( -26.02091320914878025, 51.66888916574269075, -14.97647472619899389 ) ) ;
#4376=CARTESIAN_POINT ( 'NONE',  ( -2.584737979205442066E-13, 60.55468749999998579, -30.02300923189239867 ) ) ;
#4380=CARTESIAN_POINT ( 'NONE',  ( 26.07999730980490227, 27.18229166666666430, 6.988114217767821046 ) ) ;
#4391=CARTESIAN_POINT ( 'NONE',  ( 7.468012846824281681, 28.32253499907601579, -28.02196122052058058 ) ) ;
#4392=CARTESIAN_POINT ( 'NONE',  ( 6.988114217768294445, 20.88020833333333215, 26.07999730980477437 ) ) ;
#4394=CARTESIAN_POINT ( 'NONE',  ( 19.06425588902558133, 35.48399333240935505, -19.11951029504797006 ) ) ;
#4398=CARTESIAN_POINT ( 'NONE',  ( -13.97622843553632421, 63.70572916666667140, -24.20753774853731599 ) ) ;
#4403=CARTESIAN_POINT ( 'NONE',  ( -26.00068869287368756, 29.04427083333332504, -15.01150461594595775 ) ) ;
#4404=CARTESIAN_POINT ( 'NONE',  ( -15.04653450569291984, 33.06027750092398776, 25.98046417659859486 ) ) ;
#4414=CARTESIAN_POINT ( 'NONE',  ( 14.97647472619947351, 63.42486083425730925, 26.02091320914850314 ) ) ;
#4417=CARTESIAN_POINT ( 'NONE',  ( 26.00068869287367690, 30.76302083333332860, 15.01150461594596486 ) ) ;
#4422=CARTESIAN_POINT ( 'NONE',  ( 19.06425588902558133, 52.67149333240935505, -19.11951029504797006 ) ) ;
#4429=CARTESIAN_POINT ( 'NONE',  ( -24.22776226481240514, 50.53423583425731636, 13.94119854578937812 ) ) ;
#4435=CARTESIAN_POINT ( 'NONE',  ( 28.02196122052058413, 63.55690999907603356, 7.468012846824272799 ) ) ;
#4439=CARTESIAN_POINT ( 'NONE',  ( -27.95245687107222921, 39.07031249999997868, 2.498001805406602216E-13 ) ) ;
#4442=CARTESIAN_POINT ( 'NONE',  ( -2.584737979205441561E-13, 36.49218750000000000, -30.02300923189239512 ) ) ;
#4445=CARTESIAN_POINT ( 'NONE',  ( -20.53372385742071771, 60.70350666759063785, 20.47846945139902530 ) ) ;
#4446=CARTESIAN_POINT ( 'NONE',  ( -14.01125832528285109, 60.56027750092398065, 24.18731323226248264 ) ) ;
#4448=CARTESIAN_POINT ( 'NONE',  ( 26.02091320914876960, 15.57513916574268720, 14.97647472619900455 ) ) ;
#4472=CARTESIAN_POINT ( 'NONE',  ( -19.11951029504763611, 19.45350666759063785, 19.06425588902592239 ) ) ;
#4477=CARTESIAN_POINT ( 'NONE',  ( -20.53372385742071771, 46.95350666759064495, 20.47846945139902530 ) ) ;
#4479=CARTESIAN_POINT ( 'NONE',  ( -20.53372385742107653, 38.06211833240934084, -20.47846945139867003 ) ) ;
#4482=CARTESIAN_POINT ( 'NONE',  ( 19.11951029504797006, 60.40586833240935505, 19.06425588902558133 ) ) ;
#4485=CARTESIAN_POINT ( 'NONE',  ( -20.50609665441004736, 15.43749999999999645, -20.50609665440969565 ) ) ;
#4491=CARTESIAN_POINT ( 'NONE',  ( -26.00068869287340334, 42.22135416666666430, 15.01150461594643382 ) ) ;
#4505=CARTESIAN_POINT ( 'NONE',  ( 7.025853678916867295, 29.75482666574269075, 26.06988505166722803 ) ) ;
#4513=CARTESIAN_POINT ( 'NONE',  ( -6.988114217767819270, 52.10416666666666430, 26.07999730980490583 ) ) ;
#4517=CARTESIAN_POINT ( 'NONE',  ( -6.988114217767819270, 28.04166666666666075, 26.07999730980490583 ) ) ;
#4519=CARTESIAN_POINT ( 'NONE',  ( -28.00173670424549499, 23.46392333425730570, -7.543491769121417612 ) ) ;
#4520=CARTESIAN_POINT ( 'NONE',  ( 7.505752307972854531, 64.13541666666667140, -28.01184896238303423 ) ) ;
#4533=CARTESIAN_POINT ( 'NONE',  ( -19.06425588902591173, 37.50038166759063074, -19.11951029504763611 ) ) ;
#4541=CARTESIAN_POINT ( 'NONE',  ( -30.02300923189239512, 35.63281249999998579, 2.654126918244515359E-13 ) ) ;
#4545=CARTESIAN_POINT ( 'NONE',  ( -0.04044903255044120238, 48.80430583240936215, -30.02300923189239867 ) ) ;
#4547=CARTESIAN_POINT ( 'NONE',  ( -7.505752307972844761, 65.85416666666665719, 28.01184896238304134 ) ) ;
#4552=CARTESIAN_POINT ( 'NONE',  ( 19.09188309203694800, 24.03124999999999645, 19.09188309203660694 ) ) ;
#4566=CARTESIAN_POINT ( 'NONE',  ( -14.01125832528328985, 34.76784749907601935, -24.18731323226223040 ) ) ;
#4570=CARTESIAN_POINT ( 'NONE',  ( -6.988114217767819270, 58.97916666666666430, 26.07999730980490583 ) ) ;
#4575=CARTESIAN_POINT ( 'NONE',  ( -2.584737979205441561E-13, 33.05468750000000000, -30.02300923189239512 ) ) ;
#4576=CARTESIAN_POINT ( 'NONE',  ( 7.468012846824777284, 36.06809000092397355, 28.02196122052045268 ) ) ;
#4587=CARTESIAN_POINT ( 'NONE',  ( 20.47846945139902530, 63.28163166759064495, 20.53372385742071771 ) ) ;
#4589=CARTESIAN_POINT ( 'NONE',  ( 20.50609665441005092, 34.34374999999999289, 20.50609665440969209 ) ) ;
#4594=CARTESIAN_POINT ( 'NONE',  ( 14.01125832528330051, 53.67409749907601935, 24.18731323226221974 ) ) ;
#4607=CARTESIAN_POINT ( 'NONE',  ( -20.47846945139866648, 61.26524333240935505, 20.53372385742108008 ) ) ;
#4612=CARTESIAN_POINT ( 'NONE',  ( 24.20753774853731244, 37.06510416666666430, -13.97622843553632599 ) ) ;
#4616=CARTESIAN_POINT ( 'NONE',  ( -15.01150461594595775, 41.93489583333333570, 26.00068869287368756 ) ) ;
#4619=CARTESIAN_POINT ( 'NONE',  ( 28.00173670424549499, 56.12017333425732346, 7.543491769121417612 ) ) ;
#4620=CARTESIAN_POINT ( 'NONE',  ( -19.11951029504763611, 60.70350666759063785, 19.06425588902592239 ) ) ;
#4622=CARTESIAN_POINT ( 'NONE',  ( -20.47846945139866648, 16.57774333240934794, 20.53372385742108008 ) ) ;
#4628=FACE_OUTER_BOUND ( 'NONE', #33439, .T. ) ;
#4642=CARTESIAN_POINT ( 'NONE',  ( -26.09010956794232428, 23.17746500092398065, 6.950374756619732253 ) ) ;
#4647=CARTESIAN_POINT ( 'NONE',  ( 7.543491769121427382, 48.38579833425730925, -28.00173670424548433 ) ) ;
#4649=CARTESIAN_POINT ( 'NONE',  ( 26.02091320914876960, 36.20013916574269075, 14.97647472619900455 ) ) ;
#4654=CARTESIAN_POINT ( 'NONE',  ( 19.06425588902558133, 66.42149333240935505, -19.11951029504797006 ) ) ;
#4663=CARTESIAN_POINT ( 'NONE',  ( 7.505752307972854531, 40.07291666666666430, -28.01184896238303423 ) ) ;
#4677=CARTESIAN_POINT ( 'NONE',  ( -13.94119854578892514, 26.74701416574268720, 24.22776226481266448 ) ) ;
#4685=CARTESIAN_POINT ( 'NONE',  ( -6.988114217768288228, 50.09895833333332860, -26.07999730980477437 ) ) ;
#4689=CARTESIAN_POINT ( 'NONE',  ( 27.95245687107223276, 30.47656250000000355, -2.463307335887066074E-13 ) ) ;
#4690=CARTESIAN_POINT ( 'NONE',  ( 20.53372385742072481, 21.17225666759064850, -20.47846945139902175 ) ) ;
#4691=CARTESIAN_POINT ( 'NONE',  ( -15.01150461594642138, 63.70572916666667140, -26.00068869287340334 ) ) ;
#4701=CARTESIAN_POINT ( 'NONE',  ( -19.06425588902591173, 40.93788166759063785, -19.11951029504763611 ) ) ;
#4705=CARTESIAN_POINT ( 'NONE',  ( 26.00068869287340334, 19.87760416666666430, -15.01150461594642316 ) ) ;
#4710=CARTESIAN_POINT ( 'NONE',  ( 26.00068869287340334, 43.94010416666665719, -15.01150461594642316 ) ) ;
#4715=CARTESIAN_POINT ( 'NONE',  ( -20.53372385742107653, 48.37461833240936215, -20.47846945139867003 ) ) ;
#4717=CARTESIAN_POINT ( 'NONE',  ( -26.00068869287340334, 62.84635416666667140, 15.01150461594643559 ) ) ;
#4722=CARTESIAN_POINT ( 'NONE',  ( 13.97622843553633665, 20.73697916666666075, 24.20753774853730889 ) ) ;
#4733=CARTESIAN_POINT ( 'NONE',  ( 6.950374756619257965, 42.07253499907601935, -26.09010956794244507 ) ) ;
#4737=CARTESIAN_POINT ( 'NONE',  ( -26.07999730980490583, 63.27604166666667140, -6.988114217767815717 ) ) ;
#4742=CARTESIAN_POINT ( 'NONE',  ( 15.01150461594596308, 36.77864583333332860, -26.00068869287367335 ) ) ;
#4743=CARTESIAN_POINT ( 'NONE',  ( 0.04044903254992426173, 31.05506916759064495, -30.02300923189239867 ) ) ;
#4756=CARTESIAN_POINT ( 'NONE',  ( -25.98046417659859486, 61.41965250092398776, -15.04653450569291628 ) ) ;
#4759=CARTESIAN_POINT ( 'NONE',  ( 26.00068869287341045, 37.06510416666667140, -15.01150461594642493 ) ) ;
#4764=CARTESIAN_POINT ( 'NONE',  ( 7.025853678916867295, 50.37982666574269075, 26.06988505166722803 ) ) ;
#4770=CARTESIAN_POINT ( 'NONE',  ( -27.95245687107223276, 15.00781249999999645, 2.498001805406602216E-13 ) ) ;
#4778=CARTESIAN_POINT ( 'NONE',  ( -14.97647472619899389, 61.12201416574268364, 26.02091320914878025 ) ) ;
#4782=CARTESIAN_POINT ( 'NONE',  ( -24.20753774853756823, 35.91927083333332860, -13.97622843553588723 ) ) ;
#4785=CARTESIAN_POINT ( 'NONE',  ( -15.01150461594642138, 43.08072916666666430, -26.00068869287340334 ) ) ;
#4788=CARTESIAN_POINT ( 'NONE',  ( -7.468012846824771955, 54.97434000092398065, -28.02196122052045624 ) ) ;
#4789=CARTESIAN_POINT ( 'NONE',  ( -7.025853678916393008, 56.97954833425730925, 26.06988505166735592 ) ) ;
#4792=CARTESIAN_POINT ( 'NONE',  ( -28.01184896238304134, 66.71354166666665719, -7.505752307972844761 ) ) ;
#4812=CARTESIAN_POINT ( 'NONE',  ( -27.95245687107223986, 16.44569416759064140, -0.04044903254993292840 ) ) ;
#4817=CARTESIAN_POINT ( 'NONE',  ( -0.04044903254990864921, 49.96131916759065206, 30.02300923189239867 ) ) ;
#4819=CARTESIAN_POINT ( 'NONE',  ( -14.97647472619899389, 40.49701416574269786, 26.02091320914878025 ) ) ;
#4823=CARTESIAN_POINT ( 'NONE',  ( 19.11951029504797006, 67.28086833240935505, 19.06425588902558133 ) ) ;
#4826=CARTESIAN_POINT ( 'NONE',  ( 30.02300923189239512, 13.28906249999999289, -2.619432448724977703E-13 ) ) ;
#4832=CARTESIAN_POINT ( 'NONE',  ( 28.01184896238304134, 44.36979166666666430, 7.505752307972846538 ) ) ;
#4833=CARTESIAN_POINT ( 'NONE',  ( -7.505752307973343918, 56.97395833333333570, -28.01184896238290989 ) ) ;
#4849=CARTESIAN_POINT ( 'NONE',  ( -19.06425588902558133, 23.45274333240935150, 19.11951029504797006 ) ) ;
#4858=CARTESIAN_POINT ( 'NONE',  ( 6.988114217767829928, 53.82291666666666430, -26.07999730980489872 ) ) ;
#4862=CARTESIAN_POINT ( 'NONE',  ( 24.20753774853756113, 27.32552083333333215, 13.97622843553589789 ) ) ;
#4863=CARTESIAN_POINT ( 'NONE',  ( -25.98046417659859486, 20.16965250092397355, -15.04653450569291628 ) ) ;
#4864=CARTESIAN_POINT ( 'NONE',  ( -26.00068869287368756, 63.41927083333333570, -15.01150461594595775 ) ) ;
#4875=CARTESIAN_POINT ( 'NONE',  ( 24.18731323226247554, 45.95090250092398065, 14.01125832528285997 ) ) ;
#4879=CARTESIAN_POINT ( 'NONE',  ( -20.50609665441004736, 11.99999999999999645, -20.50609665440969565 ) ) ;
#4883=CARTESIAN_POINT ( 'NONE',  ( 30.02300923189239512, 37.35156249999997868, -2.619432448724977703E-13 ) ) ;
#4888=CARTESIAN_POINT ( 'NONE',  ( 30.02300923189239867, 56.53868083240936215, -0.04044903255044467877 ) ) ;
#4890=CARTESIAN_POINT ( 'NONE',  ( 26.00068869287367690, 65.13802083333334281, 15.01150461594596486 ) ) ;
#4896=CARTESIAN_POINT ( 'NONE',  ( -24.20753774853756823, 22.16927083333332504, -13.97622843553588723 ) ) ;
#4912=CARTESIAN_POINT ( 'NONE',  ( 26.09010956794232428, 18.02121500092397710, -6.950374756619718042 ) ) ;
#4917=CARTESIAN_POINT ( 'NONE',  ( -26.00068869287340334, 38.78385416666665719, 15.01150461594643382 ) ) ;
#4928=CARTESIAN_POINT ( 'NONE',  ( -28.02196122052045268, 60.98996500092398065, 7.468012846824790607 ) ) ;
#4930=CARTESIAN_POINT ( 'NONE',  ( -20.50609665440969209, 38.64062500000000000, 20.50609665441005092 ) ) ;
#4935=CARTESIAN_POINT ( 'NONE',  ( -26.09010956794245217, 54.96315999907602645, -6.950374756619243755 ) ) ;
#4940=CARTESIAN_POINT ( 'NONE',  ( 6.988114217767829928, 16.01041666666666075, -26.07999730980489872 ) ) ;
#4949=CARTESIAN_POINT ( 'NONE',  ( 27.95245687107223276, 15.28868083240935505, -0.04044903255042905932 ) ) ;
#4954=CARTESIAN_POINT ( 'NONE',  ( 6.988114217767829928, 43.51041666666666430, -26.07999730980489872 ) ) ;
#4958=CARTESIAN_POINT ( 'NONE',  ( 26.00068869287367335, 47.95052083333331439, 15.01150461594596308 ) ) ;
#4960=CARTESIAN_POINT ( 'NONE',  ( 26.02091320914851025, 62.56548583425730925, -14.97647472619946463 ) ) ;
#4961=CARTESIAN_POINT ( 'NONE',  ( 24.22776226481241224, 59.12798583425730925, -13.94119854578936923 ) ) ;
#4966=CARTESIAN_POINT ( 'NONE',  ( 7.468012846824281681, 14.57253499907601935, -28.02196122052058058 ) ) ;
#4985=CARTESIAN_POINT ( 'NONE',  ( -27.95245687107223986, 30.19569416759064140, -0.04044903254993292840 ) ) ;
#4991=CARTESIAN_POINT ( 'NONE',  ( 28.02196122052058413, 46.36940999907602645, 7.468012846824272799 ) ) ;
#4994=CARTESIAN_POINT ( 'NONE',  ( -19.06425588902558133, 64.70274333240935505, 19.11951029504797006 ) ) ;
#4997=CARTESIAN_POINT ( 'NONE',  ( -15.01150461594595775, 21.30989583333331794, 26.00068869287368756 ) ) ;
#5003=CARTESIAN_POINT ( 'NONE',  ( 30.02300923189239512, 40.78906249999998579, -2.619432448724977703E-13 ) ) ;
#5004=CARTESIAN_POINT ( 'NONE',  ( 28.01184896238304134, 64.99479166666665719, 7.505752307972846538 ) ) ;
#5014=CARTESIAN_POINT ( 'NONE',  ( -7.505752307973343918, 12.28645833333333037, -28.01184896238290989 ) ) ;
#5019=CARTESIAN_POINT ( 'NONE',  ( 26.06988505166722803, 32.33295166574267654, -7.025853678916862854 ) ) ;
#5027=CARTESIAN_POINT ( 'NONE',  ( -13.97622843553632421, 56.83072916666665009, -24.20753774853731599 ) ) ;
#5031=CARTESIAN_POINT ( 'NONE',  ( -24.20753774853756823, 39.35677083333333570, -13.97622843553588723 ) ) ;
#5033=CARTESIAN_POINT ( 'NONE',  ( -20.53372385742071771, 19.45350666759063785, 20.47846945139902530 ) ) ;
#5034=CARTESIAN_POINT ( 'NONE',  ( -28.00173670424535644, 23.73920166574268364, 7.543491769121936308 ) ) ;
#5040=CARTESIAN_POINT ( 'NONE',  ( 2.584737979205442066E-13, 65.71093749999998579, 27.95245687107223276 ) ) ;
#5045=CARTESIAN_POINT ( 'NONE',  ( 0.04044903254993986036, 37.93006916759064495, -27.95245687107223986 ) ) ;
#5050=CARTESIAN_POINT ( 'NONE',  ( -20.50609665440969209, 14.57812499999999645, 20.50609665441005092 ) ) ;
#5054=CARTESIAN_POINT ( 'NONE',  ( -7.505752307973343918, 36.34895833333333570, -28.01184896238290989 ) ) ;
#5058=CARTESIAN_POINT ( 'NONE',  ( -26.02091320914878025, 61.98138916574268364, -14.97647472619899389 ) ) ;
#5063=CARTESIAN_POINT ( 'NONE',  ( -6.988114217768288228, 60.41145833333332149, -26.07999730980477437 ) ) ;
#5066=CARTESIAN_POINT ( 'NONE',  ( -19.09188309203694445, 25.74999999999999645, -19.09188309203661049 ) ) ;
#5073=CARTESIAN_POINT ( 'NONE',  ( 19.06425588902592239, 46.09413166759064495, 19.11951029504763611 ) ) ;
#5085=CARTESIAN_POINT ( 'NONE',  ( -13.94119854578936923, 17.01861083425731280, -24.22776226481241224 ) ) ;
#5089=CARTESIAN_POINT ( 'NONE',  ( 20.50609665441005092, 41.21875000000000000, 20.50609665440969209 ) ) ;
#5100=CARTESIAN_POINT ( 'NONE',  ( -20.50609665440969209, 14.57812499999999645, 20.50609665441005092 ) ) ;
#5102=CARTESIAN_POINT ( 'NONE',  ( -15.01150461594595775, 41.93489583333333570, 26.00068869287368756 ) ) ;
#5103=PRODUCT_CONTEXT ( 'NONE', #5706, 'mechanical' ) ;
#5109=CARTESIAN_POINT ( 'NONE',  ( 13.94119854578893580, 52.52826416574268364, -24.22776226481265383 ) ) ;
#5122=CARTESIAN_POINT ( 'NONE',  ( 13.94119854578893580, 18.15326416574268720, -24.22776226481265383 ) ) ;
#5126=CARTESIAN_POINT ( 'NONE',  ( 13.97622843553633665, 41.36197916666666430, 24.20753774853730889 ) ) ;
#5130=CARTESIAN_POINT ( 'NONE',  ( -30.02300923189239512, 45.94531249999997868, 2.654126918244515359E-13 ) ) ;
#5132=CARTESIAN_POINT ( 'NONE',  ( 26.00068869287340334, 16.44010416666666430, -15.01150461594642316 ) ) ;
#5133=CARTESIAN_POINT ( 'NONE',  ( 7.468012846824777284, 18.88059000092397355, 28.02196122052045268 ) ) ;
#5139=CARTESIAN_POINT ( 'NONE',  ( 7.505752307972854531, 64.13541666666667140, -28.01184896238303423 ) ) ;
#5155=CARTESIAN_POINT ( 'NONE',  ( -19.11951029504763611, 29.76600666759063429, 19.06425588902592239 ) ) ;
#5162=CARTESIAN_POINT ( 'NONE',  ( -14.97647472619899389, 50.80951416574269075, 26.02091320914878025 ) ) ;
#5166=CARTESIAN_POINT ( 'NONE',  ( 6.988114217767829928, 19.44791666666666075, -26.07999730980489872 ) ) ;
#5170=CARTESIAN_POINT ( 'NONE',  ( -15.01150461594642138, 25.89322916666666430, -26.00068869287340334 ) ) ;
#5176=CARTESIAN_POINT ( 'NONE',  ( -20.47846945139902175, 37.50038166759063074, -20.53372385742072481 ) ) ;
#5179=CARTESIAN_POINT ( 'NONE',  ( -20.50609665441004736, 46.37500000000000000, -20.50609665440969565 ) ) ;
#5180=CARTESIAN_POINT ( 'NONE',  ( -30.02300923189239512, 63.13281250000000000, 2.654126918244515359E-13 ) ) ;
#5190=CARTESIAN_POINT ( 'NONE',  ( -28.01184896238304134, 22.02604166666666430, -7.505752307972844761 ) ) ;
#5194=CARTESIAN_POINT ( 'NONE',  ( -24.18731323226221974, 37.34597249907603356, 14.01125832528330406 ) ) ;
#5202=CARTESIAN_POINT ( 'NONE',  ( 13.97622843553589966, 57.40364583333333570, -24.20753774853756113 ) ) ;
#5206=CARTESIAN_POINT ( 'NONE',  ( 27.95245687107223276, 40.78906249999999289, -2.463307335887066074E-13 ) ) ;
#5207=CARTESIAN_POINT ( 'NONE',  ( 15.04653450569292872, 27.90402750092397355, -25.98046417659857710 ) ) ;
#5208=CARTESIAN_POINT ( 'NONE',  ( -28.02196122052058413, 17.15065999907602290, -7.468012846824272799 ) ) ;
#5217=CARTESIAN_POINT ( 'NONE',  ( -13.94119854578936923, 41.08111083425730214, -24.22776226481241224 ) ) ;
#5221=FACE_OUTER_BOUND ( 'NONE', #20420, .T. ) ;
#5222=MECHANICAL_DESIGN_GEOMETRIC_PRESENTATION_REPRESENTATION('',(#26044),#27111);
#5226=CARTESIAN_POINT ( 'NONE',  ( -26.00068869287340334, 52.53385416666666430, 15.01150461594643382 ) ) ;
#5231=CARTESIAN_POINT ( 'NONE',  ( 14.97647472619900455, 59.40326416574269075, -26.02091320914876960 ) ) ;
#5236=CARTESIAN_POINT ( 'NONE',  ( 24.20753774853731244, 61.12760416666666430, -13.97622843553633132 ) ) ;
#5239=CARTESIAN_POINT ( 'NONE',  ( 19.09188309203694800, 34.34374999999999289, 19.09188309203660694 ) ) ;
#5247=CARTESIAN_POINT ( 'NONE',  ( 0.04044903254993986036, 51.68006916759063785, -27.95245687107223986 ) ) ;
#5258=CARTESIAN_POINT ( 'NONE',  ( 0.04044903254993986036, 13.86756916759064318, -27.95245687107223986 ) ) ;
#5262=CARTESIAN_POINT ( 'NONE',  ( -7.505752307973343918, 43.22395833333332860, -28.01184896238290989 ) ) ;
#5266=CARTESIAN_POINT ( 'NONE',  ( 20.50609665440969565, 23.17187499999999289, -20.50609665441004736 ) ) ;
#5273=CARTESIAN_POINT ( 'NONE',  ( -28.02196122052058413, 37.77565999907600514, -7.468012846824272799 ) ) ;
#5275=CARTESIAN_POINT ( 'NONE',  ( -26.00068869287368756, 42.79427083333332149, -15.01150461594595775 ) ) ;
#5281=CARTESIAN_POINT ( 'NONE',  ( 27.95245687107223276, 63.41368083240934794, -0.04044903255042905932 ) ) ;
#5287=CARTESIAN_POINT ( 'NONE',  ( -6.988114217767819270, 14.29166666666666430, 26.07999730980490583 ) ) ;
#5295=CARTESIAN_POINT ( 'NONE',  ( -13.94119854578892514, 19.87201416574269075, 24.22776226481266448 ) ) ;
#5299=CARTESIAN_POINT ( 'NONE',  ( 19.09188309203694800, 41.21875000000000000, 19.09188309203660694 ) ) ;
#5303=CARTESIAN_POINT ( 'NONE',  ( 7.505752307972854531, 19.44791666666666075, -28.01184896238303423 ) ) ;
#5304=CARTESIAN_POINT ( 'NONE',  ( -0.04044903254990864921, 15.58631916759064495, 30.02300923189239867 ) ) ;
#5326=CARTESIAN_POINT ( 'NONE',  ( 27.95245687107223986, 28.47694416759064495, 0.04044903254993640479 ) ) ;
#5333=CARTESIAN_POINT ( 'NONE',  ( 7.543491769121922985, 43.50482666574268364, 28.00173670424535644 ) ) ;
#5336=CARTESIAN_POINT ( 'NONE',  ( -6.988114217767819270, 14.29166666666666430, 26.07999730980490583 ) ) ;
#5340=CARTESIAN_POINT ( 'NONE',  ( -26.00068869287340334, 25.03385416666666785, 15.01150461594643382 ) ) ;
#5345=CARTESIAN_POINT ( 'NONE',  ( -14.97647472619946285, 44.51861083425730214, -26.02091320914851025 ) ) ;
#5347=CARTESIAN_POINT ( 'NONE',  ( 15.01150461594596308, 53.96614583333333570, -26.00068869287367335 ) ) ;
#5348=CARTESIAN_POINT ( 'NONE',  ( -26.00068869287368756, 66.85677083333334281, -15.01150461594595775 ) ) ;
#5357=CARTESIAN_POINT ( 'NONE',  ( -20.50609665441004736, 22.31250000000000000, -20.50609665440969565 ) ) ;
#5362=CARTESIAN_POINT ( 'NONE',  ( 0.04044903255044120238, 33.33555583240935505, 27.95245687107223276 ) ) ;
#5369=CARTESIAN_POINT ( 'NONE',  ( -26.07999730980490583, 63.27604166666667140, -6.988114217767815717 ) ) ;
#5373=CARTESIAN_POINT ( 'NONE',  ( -13.97622843553588901, 38.49739583333332860, 24.20753774853756823 ) ) ;
#5375=CARTESIAN_POINT ( 'NONE',  ( 14.97647472619947351, 29.04986083425730570, 26.02091320914850314 ) ) ;
#5377=CARTESIAN_POINT ( 'NONE',  ( 20.47846945139867003, 14.85899333240935505, -20.53372385742107653 ) ) ;
#5381=CARTESIAN_POINT ( 'NONE',  ( 19.06425588902558133, 49.23399333240936215, -19.11951029504797006 ) ) ;
#5388=CARTESIAN_POINT ( 'NONE',  ( -0.04044903254992426173, 43.08631916759065916, 27.95245687107223276 ) ) ;
#5393=CARTESIAN_POINT ( 'NONE',  ( -7.505752307973343918, 15.72395833333332860, -28.01184896238290989 ) ) ;
#5398=CARTESIAN_POINT ( 'NONE',  ( 2.740863092043355209E-13, 51.96093750000000000, 30.02300923189239512 ) ) ;
#5403=CARTESIAN_POINT ( 'NONE',  ( 30.02300923189239867, 59.97618083240934794, -0.04044903255044467877 ) ) ;
#5407=CARTESIAN_POINT ( 'NONE',  ( -24.20753774853756823, 56.54427083333332860, -13.97622843553588723 ) ) ;
#5410=CARTESIAN_POINT ( 'NONE',  ( -19.09188309203660694, 31.76562499999999289, 19.09188309203694800 ) ) ;
#5416=CARTESIAN_POINT ( 'NONE',  ( -7.025853678916393008, 53.54204833425730925, 26.06988505166735592 ) ) ;
#5427=CARTESIAN_POINT ( 'NONE',  ( 14.01125832528286352, 17.59152750092397355, -24.18731323226246843 ) ) ;
#5432=CARTESIAN_POINT ( 'NONE',  ( -20.50609665441004736, 46.37500000000000000, -20.50609665440969565 ) ) ;
#5435=DIRECTION ( 'NONE',  ( -0.7071067811865526798, 0.000000000000000000, -0.7071067811865423547 ) ) ;
#5436=CARTESIAN_POINT ( 'NONE',  ( 15.01150461594643204, 24.17447916666666785, 26.00068869287340334 ) ) ;
#5442=CARTESIAN_POINT ( 'NONE',  ( -14.97647472619899389, 37.05951416574268364, 26.02091320914878025 ) ) ;
#5444=CARTESIAN_POINT ( 'NONE',  ( 26.00068869287341045, 40.50260416666666430, -15.01150461594642493 ) ) ;
#5450=CARTESIAN_POINT ( 'NONE',  ( -26.09010956794245217, 61.83815999907601935, -6.950374756619243755 ) ) ;
#5456=CARTESIAN_POINT ( 'NONE',  ( 6.988114217768294445, 17.44270833333333215, 26.07999730980477437 ) ) ;
#5463=CARTESIAN_POINT ( 'NONE',  ( 19.06425588902558133, 21.73399333240935505, -19.11951029504797006 ) ) ;
#5467=CARTESIAN_POINT ( 'NONE',  ( 13.97622843553589966, 40.21614583333332860, -24.20753774853756113 ) ) ;
#5473=CARTESIAN_POINT ( 'NONE',  ( 7.505752307972854531, 12.57291666666666252, -28.01184896238303423 ) ) ;
#5474=CARTESIAN_POINT ( 'NONE',  ( 25.98046417659858420, 11.57590250092397355, 15.04653450569292872 ) ) ;
#5485=( LENGTH_UNIT ( ) NAMED_UNIT ( * ) SI_UNIT ( .MILLI., .METRE. ) );
#5495=CARTESIAN_POINT ( 'NONE',  ( -19.06425588902591173, 27.18788166759063785, -19.11951029504763611 ) ) ;
#5503=CARTESIAN_POINT ( 'NONE',  ( 28.00173670424535644, 42.64545166574268364, -7.543491769121920321 ) ) ;
#5506=PRODUCT_DEFINITION_FORMATION_WITH_SPECIFIED_SOURCE ( 'ANY', '', #23326, .NOT_KNOWN. ) ;
#5507=CARTESIAN_POINT ( 'NONE',  ( -26.07999730980490583, 15.15104166666666252, -6.988114217767815717 ) ) ;
#5509=CARTESIAN_POINT ( 'NONE',  ( 30.02300923189239512, 23.60156250000000000, -2.619432448724977703E-13 ) ) ;
#5513=CARTESIAN_POINT ( 'NONE',  ( 20.53372385742072481, 45.23475666759063785, -20.47846945139902175 ) ) ;
#5515=CARTESIAN_POINT ( 'NONE',  ( 15.01150461594596308, 50.52864583333333570, -26.00068869287367335 ) ) ;
#5527=CARTESIAN_POINT ( 'NONE',  ( -30.02300923189239867, 21.88281249999999289, 2.654126918244514854E-13 ) ) ;
#5532=CARTESIAN_POINT ( 'NONE',  ( -27.95245687107223986, 37.63243083240935505, 0.04044903255043252877 ) ) ;
#5539=CARTESIAN_POINT ( 'NONE',  ( 24.20753774853756113, 61.70052083333331439, 13.97622843553589789 ) ) ;
#5543=CARTESIAN_POINT ( 'NONE',  ( 26.07999730980490227, 40.93229166666666430, 6.988114217767821046 ) ) ;
#5544=CARTESIAN_POINT ( 'NONE',  ( 7.543491769121427382, 27.76079833425730925, -28.00173670424548433 ) ) ;
#5545=CARTESIAN_POINT ( 'NONE',  ( 14.97647472619900455, 18.15326416574268720, -26.02091320914876960 ) ) ;
#5549=CARTESIAN_POINT ( 'NONE',  ( -24.22776226481266448, 48.23138916574269786, -13.94119854578892514 ) ) ;
#5557=CARTESIAN_POINT ( 'NONE',  ( 13.94119854578937812, 49.67486083425730925, 24.22776226481240514 ) ) ;
#5561=CARTESIAN_POINT ( 'NONE',  ( -15.01150461594595775, 21.30989583333331794, 26.00068869287368756 ) ) ;
#5565=CARTESIAN_POINT ( 'NONE',  ( -20.50609665440969209, 45.51562500000000000, 20.50609665441005092 ) ) ;
#5571=CARTESIAN_POINT ( 'NONE',  ( 28.00173670424535644, 63.27045166574269075, -7.543491769121920321 ) ) ;
#5576=CARTESIAN_POINT ( 'NONE',  ( -2.428612866367529427E-13, 57.11718750000000711, -27.95245687107223276 ) ) ;
#5579=CARTESIAN_POINT ( 'NONE',  ( 13.97622843553589966, 36.77864583333332860, -24.20753774853756113 ) ) ;
#5585=CARTESIAN_POINT ( 'NONE',  ( 0.04044903254993986036, 61.99256916759065206, -27.95245687107223986 ) ) ;
#5596=CARTESIAN_POINT ( 'NONE',  ( 24.18731323226247554, 15.01340250092397888, 14.01125832528285997 ) ) ;
#5602=CARTESIAN_POINT ( 'NONE',  ( -7.505752307972844761, 38.35416666666666430, 28.01184896238304134 ) ) ;
#5605=CARTESIAN_POINT ( 'NONE',  ( -19.79898987322349768, 67.00000000000000000, -19.79898987322315307 ) ) ;
#5606=CARTESIAN_POINT ( 'NONE',  ( 26.00068869287367335, 17.01302083333332504, 15.01150461594596308 ) ) ;
#5612=CARTESIAN_POINT ( 'NONE',  ( 15.04653450569339945, 33.04909749907601935, 25.98046417659831775 ) ) ;
#5614=CARTESIAN_POINT ( 'NONE',  ( 26.00068869287367690, 47.95052083333332149, 15.01150461594596486 ) ) ;
#5620=CARTESIAN_POINT ( 'NONE',  ( 19.06425588902558133, 66.42149333240935505, -19.11951029504797006 ) ) ;
#5626=CARTESIAN_POINT ( 'NONE',  ( -13.97622843553632777, 25.89322916666666430, -24.20753774853731599 ) ) ;
#5633=CARTESIAN_POINT ( 'NONE',  ( 24.22776226481265383, 32.76263916574268364, 13.94119854578893580 ) ) ;
#5636=CARTESIAN_POINT ( 'NONE',  ( -27.95245687107222921, 42.50781249999997868, 2.498001805406602216E-13 ) ) ;
#5640=CARTESIAN_POINT ( 'NONE',  ( -15.01150461594642138, 15.58072916666666607, -26.00068869287340334 ) ) ;
#5641=CARTESIAN_POINT ( 'NONE',  ( 15.04653450569292872, 14.15402750092397532, -25.98046417659857710 ) ) ;
#5664=CARTESIAN_POINT ( 'NONE',  ( -13.94119854578936923, 30.76861083425731280, -24.22776226481241224 ) ) ;
#5674=CARTESIAN_POINT ( 'NONE',  ( -0.04044903255044120238, 45.36680583240934794, -30.02300923189239867 ) ) ;
#5678=SURFACE_STYLE_FILL_AREA ( #15651 ) ;
#5679=CARTESIAN_POINT ( 'NONE',  ( 2.584737979205441561E-13, 17.58593749999999645, 27.95245687107222921 ) ) ;
#5681=CARTESIAN_POINT ( 'NONE',  ( 26.00068869287367335, 23.88802083333331794, 15.01150461594596308 ) ) ;
#5685=CARTESIAN_POINT ( 'NONE',  ( -7.468012846824771955, 41.22434000092397355, -28.02196122052045624 ) ) ;
#5687=CARTESIAN_POINT ( 'NONE',  ( 7.505752307972854531, 50.38541666666666430, -28.01184896238303423 ) ) ;
#5698=CARTESIAN_POINT ( 'NONE',  ( 28.01184896238304134, 23.74479166666666430, 7.505752307972846538 ) ) ;
#5706=APPLICATION_CONTEXT ( 'automotive_design' ) ;
#5710=CARTESIAN_POINT ( 'NONE',  ( -6.988114217768288228, 63.84895833333332860, -26.07999730980477437 ) ) ;
#5715=CARTESIAN_POINT ( 'NONE',  ( 24.20753774853731244, 37.06510416666667140, -13.97622843553633132 ) ) ;
#5716=CARTESIAN_POINT ( 'NONE',  ( 20.47846945139902530, 25.46913166759064140, 20.53372385742071771 ) ) ;
#5717=CARTESIAN_POINT ( 'NONE',  ( -30.02300923189239867, 20.44493083240935150, 0.04044903255044988294 ) ) ;
#5721=CARTESIAN_POINT ( 'NONE',  ( 7.025853678916867295, 46.94232666574269075, 26.06988505166722803 ) ) ;
#5727=CARTESIAN_POINT ( 'NONE',  ( 24.18731323226247554, 52.82590250092398065, 14.01125832528285997 ) ) ;
#5731=CARTESIAN_POINT ( 'NONE',  ( -20.50609665440969209, 28.32812499999999645, 20.50609665441005092 ) ) ;
#5735=CARTESIAN_POINT ( 'NONE',  ( -20.50609665441004736, 49.81249999999999289, -20.50609665440969565 ) ) ;
#5741=CARTESIAN_POINT ( 'NONE',  ( -20.53372385742107653, 65.56211833240934084, -20.47846945139867003 ) ) ;
#5745=CARTESIAN_POINT ( 'NONE',  ( -13.97622843553632777, 60.26822916666665719, -24.20753774853731599 ) ) ;
#5748=CARTESIAN_POINT ( 'NONE',  ( -13.97622843553632421, 32.76822916666666430, -24.20753774853731599 ) ) ;
#5753=CARTESIAN_POINT ( 'NONE',  ( 6.950374756619721595, 53.25559000092396644, 26.09010956794232428 ) ) ;
#5765=CARTESIAN_POINT ( 'NONE',  ( 24.18731323226247554, 25.32590250092397710, 14.01125832528285997 ) ) ;
#5770=CARTESIAN_POINT ( 'NONE',  ( -20.50609665441004736, 53.25000000000000000, -20.50609665440969565 ) ) ;
#5774=CARTESIAN_POINT ( 'NONE',  ( 26.00068869287340334, 19.87760416666666430, -15.01150461594642316 ) ) ;
#5780=CARTESIAN_POINT ( 'NONE',  ( -25.98046417659831420, 37.34597249907603356, 15.04653450569339945 ) ) ;
#5782=CARTESIAN_POINT ( 'NONE',  ( 15.01150461594596486, 50.52864583333332149, -26.00068869287367690 ) ) ;
#5785=CARTESIAN_POINT ( 'NONE',  ( 13.94119854578893580, 62.84076416574269786, -24.22776226481265383 ) ) ;
#5791=CARTESIAN_POINT ( 'NONE',  ( -13.97622843553588901, 21.30989583333332504, 24.20753774853756823 ) ) ;
#5800=CARTESIAN_POINT ( 'NONE',  ( -26.06988505166722803, 23.73920166574268364, 7.025853678916877953 ) ) ;
#5803=CARTESIAN_POINT ( 'NONE',  ( -26.07999730980490583, 49.52604166666666430, -6.988114217767815717 ) ) ;
#5809=CARTESIAN_POINT ( 'NONE',  ( -30.02300923189239512, 18.44531249999999645, 2.654126918244515359E-13 ) ) ;
#5810=CARTESIAN_POINT ( 'NONE',  ( 28.02196122052045268, 11.14621500092397532, -7.468012846824774620 ) ) ;
#5832=CARTESIAN_POINT ( 'NONE',  ( 13.94119854578937812, 42.79986083425731636, 24.22776226481240514 ) ) ;
#5835=PRODUCT_DEFINITION_CONTEXT ( 'detailed design', #9647, 'design' ) ;
#5840=CARTESIAN_POINT ( 'NONE',  ( -30.02300923189239867, 54.81993083240935505, 0.04044903255044988294 ) ) ;
#5843=CARTESIAN_POINT ( 'NONE',  ( 2.584737979205441561E-13, 14.14843749999999289, 27.95245687107222921 ) ) ;
#5846=CARTESIAN_POINT ( 'NONE',  ( 30.02300923189239512, 33.91406249999997158, -2.619432448724977703E-13 ) ) ;
#5849=CARTESIAN_POINT ( 'NONE',  ( -0.04044903254990864921, 39.64881916759063074, 30.02300923189239867 ) ) ;
#5851=CARTESIAN_POINT ( 'NONE',  ( -26.00068869287340334, 52.53385416666666430, 15.01150461594643382 ) ) ;
#5870=ORIENTED_EDGE ( 'NONE', *, *, #30899, .F. ) ;
#5872=CARTESIAN_POINT ( 'NONE',  ( -13.94119854578936923, 13.58111083425730925, -24.22776226481241224 ) ) ;
#5878=CARTESIAN_POINT ( 'NONE',  ( 27.95245687107223276, 51.10156249999998579, -2.463307335887066074E-13 ) ) ;
#5879=CARTESIAN_POINT ( 'NONE',  ( -26.02091320914849959, 29.90923583425730925, 14.97647472619947528 ) ) ;
#5881=CARTESIAN_POINT ( 'NONE',  ( 28.00173670424535644, 32.33295166574267654, -7.543491769121920321 ) ) ;
#5885=CARTESIAN_POINT ( 'NONE',  ( 24.18731323226221974, 42.50222249907603356, -14.01125832528328985 ) ) ;
#5891=CARTESIAN_POINT ( 'NONE',  ( -27.95245687107223986, 47.38319416759065206, -0.04044903254993292840 ) ) ;
#5895=CARTESIAN_POINT ( 'NONE',  ( 20.50609665440969565, 23.17187499999999289, -20.50609665441004736 ) ) ;
#5899=CARTESIAN_POINT ( 'NONE',  ( 30.02300923189239512, 51.10156249999998579, -2.619432448724977703E-13 ) ) ;
#5907=CARTESIAN_POINT ( 'NONE',  ( 28.00173670424535644, 66.70795166574268364, -7.543491769121920321 ) ) ;
#5914=CARTESIAN_POINT ( 'NONE',  ( -26.07999730980490583, 32.33854166666666430, -6.988114217767815717 ) ) ;
#5920=CARTESIAN_POINT ( 'NONE',  ( -14.01125832528285109, 60.56027750092398065, 24.18731323226248264 ) ) ;
#5933=CARTESIAN_POINT ( 'NONE',  ( -19.11951029504763611, 19.45350666759063785, 19.06425588902592239 ) ) ;
#5937=CARTESIAN_POINT ( 'NONE',  ( 7.505752307972854531, 53.82291666666666430, -28.01184896238303423 ) ) ;
#5940=CARTESIAN_POINT ( 'NONE',  ( -30.02300923189239512, 21.88281249999999645, 2.654126918244515359E-13 ) ) ;
#5948=CARTESIAN_POINT ( 'NONE',  ( -28.00173670424535644, 30.61420166574267654, 7.543491769121936308 ) ) ;
#5950=CARTESIAN_POINT ( 'NONE',  ( -20.50609665440969209, 45.51562500000000000, 20.50609665441005092 ) ) ;
#5952=CARTESIAN_POINT ( 'NONE',  ( -24.22776226481266448, 65.41888916574268364, -13.94119854578892514 ) ) ;
#5958=CARTESIAN_POINT ( 'NONE',  ( 6.988114217767829928, 19.44791666666666075, -26.07999730980489872 ) ) ;
#5966=CARTESIAN_POINT ( 'NONE',  ( 13.94119854578893580, 31.90326416574268364, -24.22776226481265383 ) ) ;
#5971=CARTESIAN_POINT ( 'NONE',  ( -19.09188309203694445, 49.81249999999999289, -19.09188309203661049 ) ) ;
#5975=CARTESIAN_POINT ( 'NONE',  ( -7.505752307973343918, 22.59895833333332860, -28.01184896238290989 ) ) ;
#5976=CARTESIAN_POINT ( 'NONE',  ( 26.02091320914851025, 24.75298583425730925, -14.97647472619946463 ) ) ;
#5994=CARTESIAN_POINT ( 'NONE',  ( 26.09010956794232428, 35.20871500092396644, -6.950374756619718042 ) ) ;
#6002=CARTESIAN_POINT ( 'NONE',  ( 7.468012846824281681, 55.82253499907601935, -28.02196122052058058 ) ) ;
#6006=CARTESIAN_POINT ( 'NONE',  ( 2.584737979205441561E-13, 27.89843750000000000, 27.95245687107222921 ) ) ;
#6009=CARTESIAN_POINT ( 'NONE',  ( 20.50609665441005092, 27.46875000000000000, 20.50609665440969209 ) ) ;
#6012=CARTESIAN_POINT ( 'NONE',  ( 0.04044903254992426173, 48.24256916759064495, -30.02300923189239867 ) ) ;
#6014=CARTESIAN_POINT ( 'NONE',  ( 15.01150461594643204, 51.67447916666665719, 26.00068869287340334 ) ) ;
#6032=CARTESIAN_POINT ( 'NONE',  ( 27.95245687107223986, 11.28944416759064140, 0.04044903254993640479 ) ) ;
#6037=CARTESIAN_POINT ( 'NONE',  ( 13.97622843553633842, 48.23697916666665009, 24.20753774853730889 ) ) ;
#6038=CARTESIAN_POINT ( 'NONE',  ( -7.543491769121417612, 43.22954833425730925, 28.00173670424549499 ) ) ;
#6039=CARTESIAN_POINT ( 'NONE',  ( 20.47846945139867003, 25.17149333240934439, -20.53372385742107653 ) ) ;
#6041=CARTESIAN_POINT ( 'NONE',  ( -19.11951029504797006, 55.24961833240936926, -19.06425588902558133 ) ) ;
#6047=CARTESIAN_POINT ( 'NONE',  ( -19.06425588902591173, 47.81288166759064495, -19.11951029504763611 ) ) ;
#6051=CARTESIAN_POINT ( 'NONE',  ( 2.740863092043355209E-13, 27.89843750000000000, 30.02300923189239512 ) ) ;
#6055=CARTESIAN_POINT ( 'NONE',  ( -7.505752307973343918, 56.97395833333333570, -28.01184896238290989 ) ) ;
#6062=CARTESIAN_POINT ( 'NONE',  ( -28.00173670424535644, 68.42670166574269786, 7.543491769121936308 ) ) ;
#6069=CARTESIAN_POINT ( 'NONE',  ( -19.09188309203660694, 38.64062500000000000, 19.09188309203694800 ) ) ;
#6075=CARTESIAN_POINT ( 'NONE',  ( -26.02091320914849959, 16.15923583425731636, 14.97647472619947528 ) ) ;
#6077=CARTESIAN_POINT ( 'NONE',  ( 28.01184896238290278, 54.39583333333332860, -7.505752307973347470 ) ) ;
#6090=CARTESIAN_POINT ( 'NONE',  ( -26.06988505166735237, 23.46392333425730570, -7.025853678916388567 ) ) ;
#6096=CARTESIAN_POINT ( 'NONE',  ( 2.740863092043355209E-13, 51.96093750000000000, 30.02300923189239512 ) ) ;
#6100=CARTESIAN_POINT ( 'NONE',  ( 28.01184896238290278, 30.33333333333332860, -7.505752307973347470 ) ) ;
#6106=CARTESIAN_POINT ( 'NONE',  ( 14.97647472619900455, 45.65326416574269786, -26.02091320914876960 ) ) ;
#6109=CARTESIAN_POINT ( 'NONE',  ( 30.02300923189239867, 51.10156249999998579, -2.619432448724978208E-13 ) ) ;
#6111=CARTESIAN_POINT ( 'NONE',  ( -26.06988505166722803, 68.42670166574269786, 7.025853678916877953 ) ) ;
#6117=CARTESIAN_POINT ( 'NONE',  ( -24.20753774853730889, 25.03385416666666430, 13.97622843553634020 ) ) ;
#6125=CARTESIAN_POINT ( 'NONE',  ( -24.22776226481266448, 31.04388916574268364, -13.94119854578892514 ) ) ;
#6129=CARTESIAN_POINT ( 'NONE',  ( 19.09188309203661049, 54.10937499999999289, -19.09188309203694445 ) ) ;
#6133=CARTESIAN_POINT ( 'NONE',  ( 28.01184896238304134, 27.18229166666666430, 7.505752307972846538 ) ) ;
#6134=CARTESIAN_POINT ( 'NONE',  ( -20.47846945139902175, 20.31288166759063785, -20.53372385742072481 ) ) ;
#6143=CARTESIAN_POINT ( 'NONE',  ( -20.53372385742071771, 57.26600666759063785, 20.47846945139902530 ) ) ;
#6148=CARTESIAN_POINT ( 'NONE',  ( 19.06425588902558133, 35.48399333240935505, -19.11951029504797006 ) ) ;
#6155=CARTESIAN_POINT ( 'NONE',  ( 14.01125832528286352, 41.65402750092398065, -24.18731323226246843 ) ) ;
#6159=UNCERTAINTY_MEASURE_WITH_UNIT (LENGTH_MEASURE( 1.000000000000000082E-05 ), #146, 'distance_accuracy_value', 'NONE');
#6165=CARTESIAN_POINT ( 'NONE',  ( 26.02091320914876960, 60.26263916574269786, 14.97647472619900455 ) ) ;
#6170=CARTESIAN_POINT ( 'NONE',  ( -26.07999730980490583, 25.46354166666666430, -6.988114217767815717 ) ) ;
#6173=CARTESIAN_POINT ( 'NONE',  ( 26.00068869287340334, 30.19010416666665719, -15.01150461594642316 ) ) ;
#6176=CARTESIAN_POINT ( 'NONE',  ( -28.00173670424549499, 47.52642333425731636, -7.543491769121417612 ) ) ;
#6178=CARTESIAN_POINT ( 'NONE',  ( 28.01184896238290278, 61.27083333333332860, -7.505752307973347470 ) ) ;
#6186=CARTESIAN_POINT ( 'NONE',  ( 0.000000000000000000, 0.000000000000000000, 0.000000000000000000 ) ) ;
#6199=CARTESIAN_POINT ( 'NONE',  ( 26.07999730980490227, 64.99479166666665719, 6.988114217767821046 ) ) ;
#6204=CARTESIAN_POINT ( 'NONE',  ( -13.97622843553588901, 45.37239583333332860, 24.20753774853756823 ) ) ;
#6205=CARTESIAN_POINT ( 'NONE',  ( 30.02300923189239867, 38.78944416759064495, 0.04044903254992252006 ) ) ;
#6206=CARTESIAN_POINT ( 'NONE',  ( -28.02196122052058413, 24.02565999907602290, -7.468012846824272799 ) ) ;
#6209=CARTESIAN_POINT ( 'NONE',  ( 24.18731323226221974, 59.68972249907602645, -14.01125832528328985 ) ) ;
#6216=CARTESIAN_POINT ( 'NONE',  ( -13.94119854578936923, 54.83111083425730214, -24.22776226481241224 ) ) ;
#6222=CARTESIAN_POINT ( 'NONE',  ( -15.01150461594595775, 28.18489583333332860, 26.00068869287368756 ) ) ;
#6227=CARTESIAN_POINT ( 'NONE',  ( -7.505752307972844761, 62.41666666666666430, 28.01184896238304134 ) ) ;
#6233=CARTESIAN_POINT ( 'NONE',  ( -26.09010956794245217, 20.58815999907601935, -6.950374756619243755 ) ) ;
#6241=CARTESIAN_POINT ( 'NONE',  ( 6.988114217768294445, 44.94270833333332860, 26.07999730980477437 ) ) ;
#6248=CARTESIAN_POINT ( 'NONE',  ( 19.11951029504763611, 62.42225666759065206, -19.06425588902591173 ) ) ;
#6250=CARTESIAN_POINT ( 'NONE',  ( 28.01184896238290278, 57.83333333333333570, -7.505752307973347470 ) ) ;
#6261=CARTESIAN_POINT ( 'NONE',  ( -24.22776226481240514, 26.47173583425730925, 13.94119854578937812 ) ) ;
#6268=CARTESIAN_POINT ( 'NONE',  ( 20.50609665440969565, 50.67187500000000000, -20.50609665441004736 ) ) ;
#6272=CARTESIAN_POINT ( 'NONE',  ( -15.01150461594642138, 29.33072916666665719, -26.00068869287340334 ) ) ;
#6278=CARTESIAN_POINT ( 'NONE',  ( -30.02300923189239867, 47.94493083240935505, 0.04044903255044988294 ) ) ;
#6280=CARTESIAN_POINT ( 'NONE',  ( -28.01184896238290278, 52.67708333333333570, 7.505752307973363457 ) ) ;
#6283=CARTESIAN_POINT ( 'NONE',  ( -6.988114217767819270, 14.29166666666666430, 26.07999730980490583 ) ) ;
#6289=CARTESIAN_POINT ( 'NONE',  ( -13.97622843553588901, 24.74739583333332860, 24.20753774853756823 ) ) ;
#6295=CARTESIAN_POINT ( 'NONE',  ( -7.468012846824272799, 23.16628499907601579, 28.02196122052058413 ) ) ;
#6297=CARTESIAN_POINT ( 'NONE',  ( -14.01125832528328985, 27.89284749907601935, -24.18731323226223040 ) ) ;
#6301=CARTESIAN_POINT ( 'NONE',  ( 13.97622843553633665, 55.11197916666664298, 24.20753774853730889 ) ) ;
#6306=CARTESIAN_POINT ( 'NONE',  ( 20.50609665440969565, 23.17187499999999289, -20.50609665441004736 ) ) ;
#6307=CARTESIAN_POINT ( 'NONE',  ( 20.47846945139902530, 22.03163166759064495, 20.53372385742071771 ) ) ;
#6318=CARTESIAN_POINT ( 'NONE',  ( 7.543491769121427382, 58.69829833425730925, -28.00173670424548433 ) ) ;
#6320=CARTESIAN_POINT ( 'NONE',  ( 15.01150461594596486, 19.59114583333332504, -26.00068869287367690 ) ) ;
#6326=CARTESIAN_POINT ( 'NONE',  ( -27.95245687107223986, 44.50743083240935505, 0.04044903255043252877 ) ) ;
#6332=CARTESIAN_POINT ( 'NONE',  ( -6.950374756619716266, 41.22434000092397355, -26.09010956794232428 ) ) ;
#6339=CARTESIAN_POINT ( 'NONE',  ( 0.04044903255045854962, 57.39805583240935505, 30.02300923189239867 ) ) ;
#6342=CARTESIAN_POINT ( 'NONE',  ( -26.07999730980490583, 28.90104166666666785, -6.988114217767815717 ) ) ;
#6345=CARTESIAN_POINT ( 'NONE',  ( -15.01150461594595775, 35.05989583333332860, 26.00068869287368756 ) ) ;
#6348=CARTESIAN_POINT ( 'NONE',  ( -20.53372385742071771, 50.39100666759063785, 20.47846945139902530 ) ) ;
#6351=CARTESIAN_POINT ( 'NONE',  ( 20.50609665440969565, 57.54687500000000000, -20.50609665441004736 ) ) ;
#6371=CARTESIAN_POINT ( 'NONE',  ( 24.20753774853731244, 64.56510416666667140, -13.97622843553632599 ) ) ;
#6376=CARTESIAN_POINT ( 'NONE',  ( -19.09188309203694445, 49.81249999999999289, -19.09188309203661049 ) ) ;
#6377=CARTESIAN_POINT ( 'NONE',  ( 28.02196122052045268, 35.20871500092396644, -7.468012846824774620 ) ) ;
#6378=CARTESIAN_POINT ( 'NONE',  ( -20.53372385742107653, 27.74961833240935505, -20.47846945139867003 ) ) ;
#6382=CARTESIAN_POINT ( 'NONE',  ( 6.950374756619257965, 52.38503499907601224, -26.09010956794244507 ) ) ;
#6390=CARTESIAN_POINT ( 'NONE',  ( -26.00068869287368756, 32.48177083333332860, -15.01150461594595775 ) ) ;
#6395=CARTESIAN_POINT ( 'NONE',  ( 30.02300923189239512, 57.97656249999997868, -2.619432448724977703E-13 ) ) ;
#6400=( BOUNDED_SURFACE ( )  B_SPLINE_SURFACE ( 3, 2, ( 
 ( #33481, #14619, #27656, #9983, #19937, #28341, #22502, #27829, #1556, #4826, #32953, #20114, #25251, #9455, #14787, #2250, #30559, #2080, #15306, #23195, #33657, #30732, #6885, #27998, #4485, #25427, #12382, #22851, #7225, #17711, #17366, #10155, #1726, #12206, #22677, #33128, #31749, #2603, #25933, #24045, #26613, #514, #23705, #29176, #15655, #13064, #2766, #11000, #10491, #33831, #18055, #8081, #20804, #171, #18566, #3111, #29009, #31248, #2937, #13407, #23876, #10661, #31419, #15822, #346, #4997, #28500, #10830, #10328, #21309, #2427, #18229, #7575, #8241, #15480, #1, #26105, #12895, #28675, #16159, #20968, #5509, #18734, #5681, #13583, #21140, #23370, #7912, #18396, #28842, #13230, #5340, #31581, #26276, #7740, #31080, #15990, #5170, #23540, #26446, #22139, #26939, #16325, #14413, #16988, #24866, #14077, #19564, #6009, #3439, #27110, #1347, #848, #24209, #8410, #32417, #11168, #24536, #8913, #27446, #19396, #21639, #27279, #3772, #14243, #1007, #21804, #6173, #32085, #19230, #16483, #3603, #30011, #6517, #13909, #9082, #11328, #29844, #18898, #16655, #32253, #24700, #8581, #21471, #3938, #682, #32583, #24375, #31917, #21969, #19065, #29504, #29345, #5846, #8746, #26781, #11490, #3272, #1177, #29667, #13740, #6345, #16823, #11658, #17498, #12515, #12164, #14748, #25726, #25560, #2040, #4442, #1519, #20074, #30689, #17162, #22982, #20247, #22462, #14918, #27619, #9592, #7015, #11994, #32913, #25386, #33090, #30517, #27960, #22305, #1863, #9412, #25210, #30346, #6678, #19896, #30865, #1688, #33269, #33441, #9939, #28128, #12340, #30175, #22638, #22810, #9762, #7186, #17667, #4616, #15092, #9243, #20414, #7357, #6847, #17844, #28298, #4785, #17325, #4105, #15264, #11828, #32750, #19730, #14578, #27789, #4274, #25039, #7869, #2386, #20594, #12683, #18190, #31040, #31211, #28631, #20932, #5130, #7535, #15616, #26068, #2561, #7703, #12856, #33795, #18019, #23331, #28465, #20767, #33959, #10453, #4958, #23502, #25890, #13028, #23150, #10289, #31379, #2205, #15438, #33615, #10115, #24607, #32822, #21715, #11399, #11728, #21876, #1081, #22210, #27356, #32657, #8654, #1249, #19798, #9313, #30247, #9152, #16561, #4181, #3677, #6751, #17231, #19139, #19635, #24286, #3841, #19300, #22043, #758, #11561, #30079, #27691, #11239, #27522, #29576, #6077, #32161, #920, #27014, #6422, #16893, #29744, #32326, #14316, #32487, #6585, #4009, #14483, #8989, #24771, #3511, #17061, #24939, #19470, #29919, #13982, #24444, #8817, #1424, #6250, #11902, #22374, #16729, #27185, #14151, #25288, #17745, #19975, #12418, #9842, #14824, #1760, #28205, #1941, #22888, #33345, #25115, #20320, #12240, #30944, #22538, #1590, #7441, #27866, #17925, #30421, #22717, #12068, #28376, #32988, #17574, #33166, #9493, #9669, #33696, #28033, #2115, #25799, #4864, #15345, #4691, #6920, #25465, #4520, #30769, #7259, #15170, #25636, #12588, #17402, #2289, #23058, #20150, #10197, #31117, #12763, #30594, #4348, #7610, #20677, #18091, #33518, #23236, #7090 ),
 ( #10022, #14995, #20495, #28538, #14655, #18603, #5377, #23743, #28710, #2801, #23574, #21176, #13616, #24081, #39, #26649, #18435, #13444, #25971, #207, #28879, #10868, #5208, #26142, #13268, #13101, #20839, #31454, #547, #5545, #18264, #15692, #3144, #11034, #15856, #2464, #8115, #10361, #18767, #2638, #12931, #23407, #31284, #10528, #10695, #5717, #26312, #7947, #18936, #29211, #16195, #31618, #21005, #15519, #31784, #33868, #29042, #16026, #7777, #26481, #21503, #2975, #23911, #31952, #8444, #21342, #383, #8275, #5034, #8777, #6206, #1041, #27143, #8950, #16686, #26813, #11689, #16856, #6039, #14443, #11859, #30043, #881, #24243, #22337, #24899, #32782, #22001, #27481, #13941, #11363, #11521, #9276, #19260, #32119, #16358, #6378, #19098, #32449, #27314, #1385, #3805, #29536, #1208, #22173, #32617, #19428, #29702, #14111, #16518, #3637, #24405, #29878, #3971, #29381, #21839, #17022, #24569, #14276, #3309, #24733, #9114, #19595, #26970, #3471, #6548, #32284, #11200, #5881, #13773, #714, #8616, #21671, #7394, #17879, #9625, #6712, #22843, #25070, #33474, #32946, #17193, #27651, #1551, #19931, #25420, #20450, #20107, #22671, #33650, #9974, #30901, #12374, #9449, #27992, #4649, #12027, #28333, #28163, #30377, #33302, #22496, #17531, #14955, #6878, #17359, #9802, #7049, #4479, #1899, #30210, #20278, #27823, #2072, #4139, #14614, #12548, #4305, #23019, #14780, #25245, #30725, #1720, #7219, #12199, #4819, #33122, #17704, #30553, #15130, #25593, #15298, #25758, #2243, #12717, #23188, #19760, #23871, #28669, #21304, #5503, #339, #28494, #23698, #26607, #10824, #5333, #31744, #26269, #2757, #8235, #10654, #18050, #28835, #18729, #29166, #10484, #13576, #21132, #5674, #16154, #8072, #25926, #23531, #31574, #3105, #4991, #24039, #7567, #15814, #10147, #2595, #18558, #20962, #23363, #13401, #20629, #18389, #31072, #24675, #29002, #7733, #164, #2931, #13223, #15473, #2420, #15983, #31412, #12887, #7905, #20797, #26439, #33824, #10318, #31241, #18223, #5162, #15647, #26098, #13058, #32410, #18891, #11485, #30004, #19557, #9076, #21962, #26776, #14406, #13903, #6509, #16982, #29338, #8905, #508, #14069, #29498, #32248, #10993, #839, #19390, #27439, #3931, #3766, #5840, #16318, #21466, #11161, #3265, #16649, #27103, #6002, #21631, #24530, #21797, #29837, #14237, #24694, #8740, #3595, #31908, #1001, #6339, #11321, #19224, #8403, #13734, #26932, #24203, #16817, #672, #32077, #22134, #32577, #24369, #8575, #27272, #19058, #1171, #16476, #3430, #29661, #6165, #11650, #30509, #25552, #25201, #27780, #4778, #4607, #15084, #17491, #14571, #33082, #9754, #30167, #2032, #33260, #1511, #27953, #6671, #22628, #20065, #25031, #11986, #4435, #12154, #9585, #7008, #1340, #14911, #22455, #7178, #32743, #11821, #17659, #4097, #28120, #17152, #32904, #22298, #12507, #9236, #4266, #9404, #19720, #19886, #9930, #14740, #12333, #22974, #33433, #20406, #25375, #27610, #1679, #1856, #22803, #20240, #30680, #30857, #7350, #30340, #17834 ),
 ( #28290, #6838, #17318, #24860, #18691, #28624, #18011, #2198, #26233, #4949, #18353, #2722, #10786, #13185, #15430, #21095, #31540, #8034, #28796, #15606, #33952, #25883, #13021, #33788, #31371, #23834, #299, #10280, #2893, #5122, #23662, #12673, #10445, #26061, #18521, #2376, #12849, #23493, #23323, #31031, #23141, #5295, #20586, #28967, #28458, #33607, #10107, #7528, #20760, #20922, #15944, #2554, #18181, #29130, #5463, #26400, #7862, #31204, #15777, #125, #7695, #13360, #10616, #21263, #31708, #8200, #15256, #25718, #5800, #26738, #8701, #26896, #3395, #13865, #16116, #24330, #16280, #21921, #13536, #26570, #32371, #18852, #8867, #10953, #3231, #3066, #19351, #23999, #8537, #24164, #470, #13700, #24652, #19023, #27062, #16773, #29793, #6297, #19184, #21429, #16444, #29463, #804, #11286, #21765, #29622, #32208, #31869, #27233, #3555, #634, #1125, #22092, #3726, #11124, #8364, #32536, #11610, #9036, #6125, #14196, #21592, #32038, #16609, #19515, #5966, #29300, #14028, #24491, #964, #11445, #5633, #25508, #6966, #19680, #1810, #12286, #22760, #9539, #30295, #14700, #30126, #27737, #14528, #12112, #4566, #15044, #24989, #17615, #9361, #4394, #16942, #25158, #19842, #33211, #6629, #17108, #4227, #4054, #11778, #22416, #1988, #30467, #9195, #27567, #28077, #12463, #6796, #1472, #9713, #22933, #1635, #6469, #17275, #14867, #11947, #20021, #20195, #22584, #33389, #9888, #25332, #33035, #22258, #17451, #32864, #27911, #29963, #27399, #30639, #7135, #3889, #14361, #24819, #1296, #32701, #4733, #31788, #16362, #5885, #29385, #8279, #13105, #718, #212, #26817, #3313, #15214, #29215, #20365, #387, #15860, #18607, #30813, #21180, #18771, #13779, #24247, #24085, #26146, #2642, #7306, #31459, #23578, #2980, #13448, #26316, #7952, #10872, #8120, #5721, #553, #11039, #29046, #23915, #17790, #21347, #16199, #31622, #5549, #28250, #44, #18439, #26653, #10532, #3148, #5381, #21507, #2805, #13620, #21009, #31956, #16030, #8449, #28883, #18940, #13272, #23747, #10699, #26485, #29706, #22340, #6551, #1389, #29539, #24736, #27654, #11862, #6382, #32786, #27318, #3808, #9279, #11692, #19101, #29881, #19763, #24904, #11524, #14617, #22176, #30213, #6715, #9117, #26974, #24572, #32621, #17196, #6041, #4143, #8619, #16859, #25073, #3640, #19599, #22005, #16522, #11204, #30046, #21842, #14279, #3474, #8953, #1211, #11366, #32287, #17025, #32452, #19432, #27484, #21675, #3974, #8780, #14446, #13945, #32123, #24408, #884, #19264, #6209, #16690, #27147, #14114, #1044, #4482, #20111, #30381, #33125, #20634, #14958, #23023, #12721, #15303, #17885, #15134, #19934, #12378, #25424, #22847, #7222, #33306, #25597, #9805, #32949, #28337, #33478, #12203, #31076, #18053, #2247, #7052, #6882, #28498, #7571, #4994, #28167, #33654, #30556, #17534, #17708, #15477, #1902, #4308, #22500, #12552, #25248, #4654, #9978, #1554, #20454, #1723, #7399, #4823, #25762, #2077, #20281, #30728, #22674, #30905, #27995, #23192, #10152, #12031, #9452, #17362 ),
 ( #27826, #9629, #14783, #23536, #26273, #13405, #29006, #23874, #10324, #2935, #21469, #10998, #512, #343, #18226, #5843, #5336, #31913, #8407, #20801, #10827, #25930, #5507, #20965, #23702, #2424, #2761, #15987, #18895, #16157, #21137, #3109, #8077, #18563, #26611, #26444, #33827, #10658, #13580, #5679, #13227, #29343, #21307, #12892, #24043, #31747, #7737, #15819, #8239, #23367, #31245, #28672, #5166, #31578, #15652, #18393, #18732, #168, #26102, #29172, #2599, #13061, #4392, #10488, #31416, #7909, #28839, #9079, #24534, #1344, #11825, #24697, #29665, #8579, #27107, #26936, #16653, #24863, #13737, #3435, #3769, #13907, #3600, #14240, #19394, #1174, #678, #27276, #22302, #32747, #9240, #11654, #19061, #30172, #6170, #19725, #16322, #11165, #22137, #26779, #29840, #11324, #14074, #3269, #1005, #32580, #24206, #21636, #19561, #32082, #29501, #6006, #24373, #16480, #32415, #8909, #21801, #845, #6342, #11488, #30009, #6514, #16986, #21966, #16820, #32251, #27443, #3935, #14409, #8744, #19227, #14575, #27785, #33265, #1516, #28124, #25207, #9936, #1685, #9759, #6843, #17663, #1861, #22979, #4102, #7183, #17322, #32910, #2202, #20411, #12160, #17840, #2037, #30861, #25036, #7354, #11991, #20244, #23147, #33611, #28294, #22634, #22459, #10112, #12679, #20591, #30685, #4782, #33087, #9589, #12337, #6675, #20070, #9409, #27615, #4612, #30343, #15088, #25556, #17158, #12511, #4271, #33438, #15261, #25722, #19892, #7012, #25381, #14745, #4439, #30514, #22807, #17495, #27957, #14915, #18694, #10450, #5467, #18016, #15781, #20928, #2897, #31208, #18186, #5299, #5126, #12853, #23498, #26572, #31543, #10285, #7699, #29134, #5636, #31375, #28462, #129, #2382, #10791, #20764, #4954, #15435, #23328, #28628, #2726, #31712, #7866, #33956, #10956, #21269, #8204, #23667, #15613, #26237, #15949, #33792, #16119, #26405, #26065, #10620, #2558, #28802, #13190, #13025, #18357, #21099, #8039, #18525, #28971, #7532, #13364, #23838, #303, #25887, #3069, #13539, #24002, #473, #31036, #8541, #31873, #14201, #5803, #24335, #5971, #16283, #19025, #6474, #809, #8871, #32541, #1129, #3730, #968, #26741, #32212, #11290, #8705, #27067, #19188, #11449, #29626, #18855, #24495, #3234, #11614, #638, #8369, #29303, #13702, #21597, #3560, #22096, #21769, #6129, #1301, #9040, #19519, #14033, #11127, #16613, #6301, #24167, #29967, #29798, #32041, #21925, #29466, #32375, #19355, #16448, #26900, #16777, #27237, #24656, #16946, #3399, #27404, #13869, #3893, #14365, #24822, #21431, #24993, #15048, #17112, #32868, #22262, #4570, #30130, #14704, #30299, #6633, #9365, #30818, #25162, #33217, #22937, #25512, #28081, #25336, #27571, #22588, #1640, #33040, #17455, #9544, #1814, #20025, #9199, #4060, #1992, #12116, #1476, #28254, #12467, #17279, #14532, #4737, #7310, #15218, #4398, #9892, #6800, #27740, #27915, #25681, #30471, #11950, #32704, #22764, #22419, #14872, #9716, #17795, #20199, #19847, #17620, #33393, #20369, #12291, #6970, #30642, #4230, #7139 ),
 ( #11782, #19684, #23283, #10407, #10244, #17972, #28587, #31670, #2689, #15392, #2338, #23796, #262, #26024, #23105, #15907, #20724, #13323, #31507, #26363, #10749, #18144, #28762, #21057, #31335, #21226, #18316, #5258, #2852, #13149, #10067, #20886, #8164, #18654, #2516, #5596, #23623, #29092, #16078, #91, #28423, #15570, #10579, #2161, #20547, #12635, #33569, #7827, #30993, #5085, #8000, #12982, #25848, #5427, #7492, #15739, #4912, #23456, #18484, #33749, #26194, #28928, #12811, #31165, #7657, #33918, #5933, #18818, #3359, #3197, #26864, #1092, #23964, #13666, #13995, #24130, #13829, #24456, #29588, #931, #10918, #3522, #22055, #11575, #32500, #11411, #29261, #6433, #16411, #9000, #19481, #21390, #21887, #26533, #6090, #21558, #24298, #3027, #770, #32337, #29930, #13498, #29756, #31835, #8329, #434, #596, #5765, #8666, #19150, #32002, #11087, #16572, #11251, #8830, #6261, #16740, #21728, #27027, #16245, #19314, #27198, #32173, #3688, #26700, #8498, #18986, #14162, #29430, #24618, #1433, #20162, #11912, #9505, #17072, #27877, #12079, #33178, #14327, #17415, #27532, #9163, #12429, #25302, #30260, #19647, #27702, #4020, #17242, #25476, #24783, #14494, #4361, #24952, #4192, #14836, #19986, #1772, #1261, #12252, #22898, #1955, #33356, #22729, #30089, #30780, #6763, #9853, #20330, #11741, #9680, #16905, #30433, #22384, #14664, #27367, #25124, #30606, #3852, #22221, #7102, #32668, #6595, #32833, #9323, #19810, #32998, #6932, #1602, #22547, #17585, #28046, #4533, #15007, #31466, #5045, #23415, #21186, #7786, #33877, #18100, #25982, #15866, #15181, #28386, #10370, #2124, #28722, #25810, #10538, #2301, #20848, #7451, #18275, #2475, #23585, #4701, #5217, #17936, #33530, #2811, #21015, #12773, #18445, #2648, #7958, #28888, #23247, #31294, #26154, #12942, #5388, #15700, #13111, #26323, #50, #25646, #13278, #23753, #218, #7620, #10705, #7273, #17756, #28214, #12599, #23069, #20687, #10033, #20508, #30954, #4875, #15356, #33708, #10206, #31128, #28548, #15529, #10878, #891, #24578, #5891, #8126, #21514, #6047, #29221, #21683, #24414, #16369, #16697, #27153, #18614, #724, #2986, #11372, #21353, #29052, #5557, #13455, #31795, #3319, #32293, #31962, #559, #11998, #21848, #8787, #24254, #8287, #26823, #16530, #23923, #19271, #26981, #18777, #11210, #393, #29391, #13786, #5727, #16205, #32130, #18946, #8625, #19108, #16036, #29546, #26659, #13951, #26491, #3155, #29712, #13627, #6216, #24091, #11049, #8457, #3645, #3480, #14121, #1524, #31628, #20078, #7538, #25390, #9943, #33619, #2209, #4789, #2044, #6852, #33273, #1867, #9767, #28133, #20251, #12519, #30693, #19901, #17329, #25730, #12345, #12168, #4961, #23154, #27964, #27793, #15441, #18022, #25893, #15098, #20598, #7020, #4446, #4620, #2389, #22814, #25214, #9416, #33445, #22642, #25564, #20418, #28468, #30869, #33094, #28302, #15268, #12688, #22986, #7190, #17671, #9597, #7362, #17502, #17848, #31044, #22467, #14923, #10119, #32917, #30350, #4278, #14752, #1692 ),
 ( #30521, #10961, #2731, #2564, #29308, #13544, #18363, #7706, #5810, #8374, #16288, #5474, #21436, #31382, #28808, #18530, #26746, #26243, #15619, #33798, #23843, #13032, #15954, #308, #18861, #10796, #23505, #18700, #29139, #5641, #26410, #13195, #31548, #33962, #10627, #7873, #28976, #31879, #12859, #5304, #478, #23672, #21274, #10293, #8044, #135, #16125, #10456, #20935, #21104, #15786, #28634, #2902, #23335, #13372, #26071, #31717, #20770, #31214, #8209, #18193, #26579, #5133, #3075, #24007, #24172, #644, #19032, #3404, #8877, #3900, #3567, #6134, #17119, #16952, #27411, #29806, #26905, #11457, #22102, #8546, #14371, #11620, #13874, #6307, #29471, #974, #32381, #24342, #814, #16784, #24501, #21931, #19361, #13707, #27243, #11295, #19525, #11133, #21603, #29974, #16453, #6480, #5976, #21774, #32046, #24828, #32220, #16618, #8710, #19193, #29631, #22268, #27073, #24663, #1307, #11788, #32710, #3736, #14039, #14207, #1135, #32547, #9046, #9206, #19690, #30136, #6639, #3239, #15054, #9551, #22943, #33401, #20031, #14540, #1820, #22426, #25519, #19853, #25000, #1482, #32874, #6806, #14879, #12473, #30477, #33047, #4743, #1998, #9898, #25343, #30307, #17461, #7145, #9371, #20375, #30648, #17285, #12298, #27748, #27921, #4404, #4236, #14710, #22770, #6978, #33223, #9722, #27577, #20208, #25168, #30823, #11956, #1647, #7316, #12122, #17801, #22595, #17626, #4066, #28088, #28259, #4576, #26617, #13412, #18572, #26280, #351, #7916, #18738, #2941, #24048, #5176, #8245, #18400, #5, #3275, #21474, #2771, #18902, #3114, #31921, #29348, #23709, #10834, #13586, #23880, #5849, #21313, #31754, #8413, #29180, #15659, #26450, #16328, #26784, #8085, #11171, #5685, #13743, #24213, #16163, #23544, #21144, #517, #685, #26109, #21642, #2607, #11004, #7744, #175, #18233, #29013, #20972, #28679, #13068, #15994, #10495, #31585, #31423, #5345, #28846, #15826, #13235, #10665, #5513, #6520, #11493, #24379, #8916, #8749, #32420, #6681, #29508, #19233, #19567, #29670, #24869, #11331, #1351, #3442, #6176, #8584, #11831, #16486, #22308, #6012, #17165, #27622, #4109, #1010, #30016, #9247, #32754, #14416, #11661, #26942, #19399, #21972, #29849, #3775, #6348, #22142, #16827, #13912, #851, #19733, #27283, #21807, #14581, #30178, #3607, #32256, #25042, #1523, #11997, #24703, #32088, #16658, #14080, #14246, #19068, #1180, #27115, #24539, #9085, #32587, #16991, #27450, #3941, #33444, #12167, #28301, #4788, #15267, #2043, #22813, #7189, #22641, #20250, #7019, #4619, #31043, #7537, #17501, #10118, #1866, #30868, #9415, #17670, #12344, #25729, #33093, #9596, #30692, #30520, #4277, #14922, #18021, #22985, #1691, #20077, #20597, #28467, #33272, #19900, #25563, #27792, #2208, #27963, #30349, #6851, #14751, #4445, #28132, #23153, #9766, #25389, #2388, #12687, #33618, #15097, #12518, #9942, #7361, #25213, #4960, #17847, #20417, #15440, #25892, #22466, #32916, #17328, #33961, #15953, #134, #10626, #21103, #23334, #31547, #23504, #29138, #20769 ),
 ( #15785, #26745, #26578, #3074, #5473, #2563, #8043, #31716, #18192, #13543, #21273, #10455, #26409, #28633, #18529, #28975, #13031, #20934, #2901, #13371, #23842, #307, #33797, #10795, #31381, #5640, #31213, #10292, #16124, #26070, #24006, #5132, #7872, #7705, #477, #15618, #10960, #18362, #31878, #8373, #18860, #26242, #8208, #21435, #29307, #5809, #18699, #28807, #23671, #2730, #16287, #12858, #5303, #13194, #24500, #643, #21602, #6479, #27072, #26904, #19689, #3899, #8709, #32045, #30135, #32709, #6638, #29805, #1306, #21773, #19192, #8876, #17118, #16617, #5975, #24171, #14206, #3403, #6306, #24662, #9205, #1134, #13873, #9045, #19524, #29973, #16783, #3566, #21930, #24341, #973, #32219, #19360, #11787, #22267, #29630, #24827, #14038, #11619, #11132, #32380, #11456, #16951, #813, #11294, #27242, #6133, #19031, #3735, #3238, #22101, #16452, #32546, #13706, #8545, #27410, #29470, #14370, #11955, #4403, #6977, #14878, #33222, #25342, #7144, #1819, #24999, #22425, #30822, #17460, #17284, #10071, #28258, #33046, #32873, #20552, #23109, #30998, #20207, #25685, #12121, #9550, #9721, #7496, #27920, #30306, #14539, #4575, #27747, #30647, #15053, #33573, #25518, #4235, #33400, #9897, #20374, #17625, #12297, #22769, #14709, #28087, #22594, #1997, #2165, #12639, #20030, #15222, #12472, #22942, #1481, #7315, #17800, #4742, #25167, #1646, #27576, #30476, #9370, #4065, #19852, #6805, #31170, #18148, #5602, #16084, #7831, #4917, #21061, #23288, #31675, #7661, #15397, #25852, #33756, #28591, #23628, #18659, #18320, #20890, #31841, #8169, #29097, #10584, #5089, #26199, #2858, #10248, #26538, #26369, #15574, #31511, #20729, #15744, #13153, #26028, #2520, #8005, #5262, #2693, #95, #28427, #18490, #12989, #267, #2343, #12815, #10754, #23460, #21232, #33922, #10412, #31339, #3032, #28766, #13505, #28933, #23969, #439, #10923, #5432, #15913, #21395, #17977, #13328, #23801, #11580, #32178, #32008, #24788, #9006, #13834, #3203, #1267, #3860, #11747, #937, #6439, #26869, #24302, #13999, #22226, #21733, #11094, #29267, #19319, #8503, #11417, #29761, #14332, #6268, #18991, #14167, #24624, #1097, #21892, #8673, #27032, #29435, #6096, #3364, #24461, #16910, #27372, #775, #29935, #19155, #16745, #5770, #3527, #29594, #22061, #5937, #16417, #16577, #11257, #24135, #32342, #8334, #8836, #21563, #27203, #18824, #16250, #3694, #26706, #32505, #13671, #19486, #602, #19652, #30094, #14500, #32838, #4833, #33838, #33005, #1606, #13071, #12902, #23377, #25772, #22389, #6938, #18062, #4025, #10335, #7584, #9329, #2258, #24957, #30439, #27882, #19815, #30267, #12732, #19992, #17421, #15313, #9168, #23203, #6767, #15487, #6601, #17078, #25941, #11918, #2435, #1441, #17248, #27538, #20811, #27708, #31255, #4198, #18236, #28682, #5180, #12084, #20644, #7747, #15663, #26112, #33665, #14669, #9510, #22552, #10162, #31087, #28507, #5004, #2610, #25129, #32672, #8248, #688, #3279, #23883, #26945, #520, #8587, #11174, #21477, #5348, #2944 ) ),
 .UNSPECIFIED., .T., .F., .T. ) 
 B_SPLINE_SURFACE_WITH_KNOTS ( ( 4, 3, 4 ),
 ( 3, 2, 2, 2, 2, 2, 2, 2, 2, 2, 2, 2, 2, 2, 2, 2, 2, 2, 2, 2, 2, 2, 2, 2, 2, 2, 2, 2, 2, 2, 2, 2, 2, 2, 2, 2, 2, 2, 2, 2, 2, 2, 2, 2, 2, 2, 2, 2, 2, 2, 2, 2, 2, 2, 2, 2, 2, 2, 2, 2, 2, 2, 2, 2, 2, 2, 2, 2, 2, 2, 2, 2, 2, 2, 2, 2, 2, 2, 2, 2, 2, 2, 2, 2, 2, 2, 2, 2, 2, 2, 2, 2, 2, 2, 2, 2, 2, 2, 2, 2, 2, 2, 2, 2, 2, 2, 2, 2, 2, 2, 2, 2, 2, 2, 2, 2, 2, 2, 2, 2, 2, 2, 2, 2, 2, 2, 2, 2, 2, 2, 2, 2, 2, 2, 2, 2, 2, 2, 2, 2, 2, 2, 2, 2, 2, 2, 2, 2, 2, 2, 2, 2, 2, 2, 2, 2, 2, 2, 2, 2, 2, 2, 2, 2, 2, 2, 2, 2, 2, 2, 2, 2, 2, 2, 2, 2, 2, 2, 2, 2, 2, 2, 2, 2, 2, 2, 2, 2, 2, 2, 2, 2, 3 ),
 ( 0.000000000000000000, 0.5000000000000000000, 1.000000000000000000 ),
 ( 0.000000000000000000, 0.005208333333333333044, 0.01041666666666666609, 0.01562500000000000000, 0.02083333333333333218, 0.02604166666666666782, 0.03125000000000000000, 0.03645833333333333565, 0.04166666666666666435, 0.04687500000000000000, 0.05208333333333333565, 0.05729166666666666435, 0.06250000000000000000, 0.06770833333333332871, 0.07291666666666667129, 0.07812500000000000000, 0.08333333333333332871, 0.08854166666666667129, 0.09375000000000000000, 0.09895833333333332871, 0.1041666666666666713, 0.1093750000000000000, 0.1145833333333333287, 0.1197916666666666713, 0.1250000000000000000, 0.1302083333333333426, 0.1354166666666666574, 0.1406250000000000000, 0.1458333333333333426, 0.1510416666666666574, 0.1562500000000000000, 0.1614583333333333426, 0.1666666666666666574, 0.1718750000000000000, 0.1770833333333333426, 0.1822916666666666574, 0.1875000000000000000, 0.1927083333333333426, 0.1979166666666666574, 0.2031250000000000000, 0.2083333333333333426, 0.2135416666666666574, 0.2187500000000000000, 0.2239583333333333426, 0.2291666666666666574, 0.2343750000000000000, 0.2395833333333333426, 0.2447916666666666574, 0.2500000000000000000, 0.2552083333333333148, 0.2604166666666666852, 0.2656250000000000000, 0.2708333333333333148, 0.2760416666666666852, 0.2812500000000000000, 0.2864583333333333148, 0.2916666666666666852, 0.2968750000000000000, 0.3020833333333333148, 0.3072916666666666852, 0.3125000000000000000, 0.3177083333333333148, 0.3229166666666666852, 0.3281250000000000000, 0.3333333333333333148, 0.3385416666666666852, 0.3437500000000000000, 0.3489583333333333148, 0.3541666666666666852, 0.3593750000000000000, 0.3645833333333333148, 0.3697916666666666852, 0.3750000000000000000, 0.3802083333333333148, 0.3854166666666666852, 0.3906250000000000000, 0.3958333333333333148, 0.4010416666666666852, 0.4062500000000000000, 0.4114583333333333148, 0.4166666666666666852, 0.4218750000000000000, 0.4270833333333333148, 0.4322916666666666852, 0.4375000000000000000, 0.4427083333333333148, 0.4479166666666666852, 0.4531250000000000000, 0.4583333333333333148, 0.4635416666666666852, 0.4687500000000000000, 0.4739583333333333148, 0.4791666666666666852, 0.4843750000000000000, 0.4895833333333333148, 0.4947916666666666852, 0.5000000000000000000, 0.5052083333333333703, 0.5104166666666666297, 0.5156250000000000000, 0.5208333333333333703, 0.5260416666666666297, 0.5312500000000000000, 0.5364583333333333703, 0.5416666666666666297, 0.5468750000000000000, 0.5520833333333333703, 0.5572916666666666297, 0.5625000000000000000, 0.5677083333333333703, 0.5729166666666666297, 0.5781250000000000000, 0.5833333333333333703, 0.5885416666666666297, 0.5937500000000000000, 0.5989583333333333703, 0.6041666666666666297, 0.6093750000000000000, 0.6145833333333333703, 0.6197916666666666297, 0.6250000000000000000, 0.6302083333333333703, 0.6354166666666666297, 0.6406250000000000000, 0.6458333333333333703, 0.6510416666666666297, 0.6562500000000000000, 0.6614583333333333703, 0.6666666666666666297, 0.6718750000000000000, 0.6770833333333333703, 0.6822916666666666297, 0.6875000000000000000, 0.6927083333333333703, 0.6979166666666666297, 0.7031250000000000000, 0.7083333333333333703, 0.7135416666666666297, 0.7187500000000000000, 0.7239583333333333703, 0.7291666666666666297, 0.7343750000000000000, 0.7395833333333333703, 0.7447916666666666297, 0.7500000000000000000, 0.7552083333333333703, 0.7604166666666666297, 0.7656250000000000000, 0.7708333333333333703, 0.7760416666666666297, 0.7812500000000000000, 0.7864583333333333703, 0.7916666666666666297, 0.7968750000000000000, 0.8020833333333333703, 0.8072916666666666297, 0.8125000000000000000, 0.8177083333333333703, 0.8229166666666666297, 0.8281250000000000000, 0.8333333333333333703, 0.8385416666666666297, 0.8437500000000000000, 0.8489583333333333703, 0.8541666666666666297, 0.8593750000000000000, 0.8645833333333333703, 0.8697916666666666297, 0.8750000000000000000, 0.8802083333333333703, 0.8854166666666666297, 0.8906250000000000000, 0.8958333333333333703, 0.9010416666666666297, 0.9062500000000000000, 0.9114583333333333703, 0.9166666666666666297, 0.9218750000000000000, 0.9270833333333333703, 0.9322916666666666297, 0.9375000000000000000, 0.9427083333333333703, 0.9479166666666666297, 0.9531250000000000000, 0.9583333333333333703, 0.9635416666666666297, 0.9687500000000000000, 0.9739583333333333703, 0.9791666666666666297, 0.9843750000000000000, 0.9895833333333333703, 0.9947916666666666297, 1.000000000000000000 ),
 .UNSPECIFIED. ) 
 GEOMETRIC_REPRESENTATION_ITEM ( )  RATIONAL_B_SPLINE_SURFACE ( (
 ( 1.000000000000000000, 0.9659258262890683122, 1.000000000000000000, 0.9659258262890683122, 1.000000000000000000, 0.9659258262890683122, 1.000000000000000000, 0.9659258262890683122, 1.000000000000000000, 0.9659258262890683122, 1.000000000000000000, 0.9659258262890683122, 1.000000000000000000, 0.9659258262890683122, 1.000000000000000000, 0.9659258262890683122, 1.000000000000000000, 0.9659258262890683122, 1.000000000000000000, 0.9659258262890683122, 1.000000000000000000, 0.9659258262890683122, 1.000000000000000000, 0.9659258262890683122, 1.000000000000000000, 0.9659258262890683122, 1.000000000000000000, 0.9659258262890683122, 1.000000000000000000, 0.9659258262890683122, 1.000000000000000000, 0.9659258262890683122, 1.000000000000000000, 0.9659258262890683122, 1.000000000000000000, 0.9659258262890683122, 1.000000000000000000, 0.9659258262890683122, 1.000000000000000000, 0.9659258262890683122, 1.000000000000000000, 0.9659258262890683122, 1.000000000000000000, 0.9659258262890683122, 1.000000000000000000, 0.9659258262890683122, 1.000000000000000000, 0.9659258262890683122, 1.000000000000000000, 0.9659258262890683122, 1.000000000000000000, 0.9659258262890683122, 1.000000000000000000, 0.9659258262890683122, 1.000000000000000000, 0.9659258262890683122, 1.000000000000000000, 0.9659258262890683122, 1.000000000000000000, 0.9659258262890683122, 1.000000000000000000, 0.9659258262890683122, 1.000000000000000000, 0.9659258262890683122, 1.000000000000000000, 0.9659258262890683122, 1.000000000000000000, 0.9659258262890683122, 1.000000000000000000, 0.9659258262890683122, 1.000000000000000000, 0.9659258262890683122, 1.000000000000000000, 0.9659258262890683122, 1.000000000000000000, 0.9659258262890683122, 1.000000000000000000, 0.9659258262890683122, 1.000000000000000000, 0.9659258262890683122, 1.000000000000000000, 0.9659258262890683122, 1.000000000000000000, 0.9659258262890683122, 1.000000000000000000, 0.9659258262890683122, 1.000000000000000000, 0.9659258262890683122, 1.000000000000000000, 0.9659258262890683122, 1.000000000000000000, 0.9659258262890683122, 1.000000000000000000, 0.9659258262890683122, 1.000000000000000000, 0.9659258262890683122, 1.000000000000000000, 0.9659258262890683122, 1.000000000000000000, 0.9659258262890683122, 1.000000000000000000, 0.9659258262890683122, 1.000000000000000000, 0.9659258262890683122, 1.000000000000000000, 0.9659258262890683122, 1.000000000000000000, 0.9659258262890683122, 1.000000000000000000, 0.9659258262890683122, 1.000000000000000000, 0.9659258262890683122, 1.000000000000000000, 0.9659258262890683122, 1.000000000000000000, 0.9659258262890683122, 1.000000000000000000, 0.9659258262890683122, 1.000000000000000000, 0.9659258262890683122, 1.000000000000000000, 0.9659258262890683122, 1.000000000000000000, 0.9659258262890683122, 1.000000000000000000, 0.9659258262890683122, 1.000000000000000000, 0.9659258262890683122, 1.000000000000000000, 0.9659258262890683122, 1.000000000000000000, 0.9659258262890683122, 1.000000000000000000, 0.9659258262890683122, 1.000000000000000000, 0.9659258262890683122, 1.000000000000000000, 0.9659258262890683122, 1.000000000000000000, 0.9659258262890683122, 1.000000000000000000, 0.9659258262890683122, 1.000000000000000000, 0.9659258262890683122, 1.000000000000000000, 0.9659258262890683122, 1.000000000000000000, 0.9659258262890683122, 1.000000000000000000, 0.9659258262890683122, 1.000000000000000000, 0.9659258262890683122, 1.000000000000000000, 0.9659258262890683122, 1.000000000000000000, 0.9659258262890683122, 1.000000000000000000, 0.9659258262890683122, 1.000000000000000000, 0.9659258262890683122, 1.000000000000000000, 0.9659258262890683122, 1.000000000000000000, 0.9659258262890683122, 1.000000000000000000, 0.9659258262890683122, 1.000000000000000000, 0.9659258262890683122, 1.000000000000000000, 0.9659258262890683122, 1.000000000000000000, 0.9659258262890683122, 1.000000000000000000, 0.9659258262890683122, 1.000000000000000000, 0.9659258262890683122, 1.000000000000000000, 0.9659258262890683122, 1.000000000000000000, 0.9659258262890683122, 1.000000000000000000, 0.9659258262890683122, 1.000000000000000000, 0.9659258262890683122, 1.000000000000000000, 0.9659258262890683122, 1.000000000000000000, 0.9659258262890683122, 1.000000000000000000, 0.9659258262890683122, 1.000000000000000000, 0.9659258262890683122, 1.000000000000000000, 0.9659258262890683122, 1.000000000000000000, 0.9659258262890683122, 1.000000000000000000, 0.9659258262890683122, 1.000000000000000000, 0.9659258262890683122, 1.000000000000000000, 0.9659258262890683122, 1.000000000000000000, 0.9659258262890683122, 1.000000000000000000, 0.9659258262890683122, 1.000000000000000000, 0.9659258262890683122, 1.000000000000000000, 0.9659258262890683122, 1.000000000000000000, 0.9659258262890683122, 1.000000000000000000, 0.9659258262890683122, 1.000000000000000000, 0.9659258262890683122, 1.000000000000000000, 0.9659258262890683122, 1.000000000000000000, 0.9659258262890683122, 1.000000000000000000, 0.9659258262890683122, 1.000000000000000000, 0.9659258262890683122, 1.000000000000000000, 0.9659258262890683122, 1.000000000000000000, 0.9659258262890683122, 1.000000000000000000, 0.9659258262890683122, 1.000000000000000000, 0.9659258262890683122, 1.000000000000000000, 0.9659258262890683122, 1.000000000000000000, 0.9659258262890683122, 1.000000000000000000, 0.9659258262890683122, 1.000000000000000000, 0.9659258262890683122, 1.000000000000000000, 0.9659258262890683122, 1.000000000000000000, 0.9659258262890683122, 1.000000000000000000, 0.9659258262890683122, 1.000000000000000000, 0.9659258262890683122, 1.000000000000000000, 0.9659258262890683122, 1.000000000000000000, 0.9659258262890683122, 1.000000000000000000, 0.9659258262890683122, 1.000000000000000000, 0.9659258262890683122, 1.000000000000000000, 0.9659258262890683122, 1.000000000000000000, 0.9659258262890683122, 1.000000000000000000, 0.9659258262890683122, 1.000000000000000000, 0.9659258262890683122, 1.000000000000000000, 0.9659258262890683122, 1.000000000000000000, 0.9659258262890683122, 1.000000000000000000, 0.9659258262890683122, 1.000000000000000000, 0.9659258262890683122, 1.000000000000000000, 0.9659258262890683122, 1.000000000000000000, 0.9659258262890683122, 1.000000000000000000, 0.9659258262890683122, 1.000000000000000000, 0.9659258262890683122, 1.000000000000000000, 0.9659258262890683122, 1.000000000000000000, 0.9659258262890683122, 1.000000000000000000, 0.9659258262890683122, 1.000000000000000000, 0.9659258262890683122, 1.000000000000000000, 0.9659258262890683122, 1.000000000000000000, 0.9659258262890683122, 1.000000000000000000, 0.9659258262890683122, 1.000000000000000000, 0.9659258262890683122, 1.000000000000000000, 0.9659258262890683122, 1.000000000000000000, 0.9659258262890683122, 1.000000000000000000, 0.9659258262890683122, 1.000000000000000000, 0.9659258262890683122, 1.000000000000000000, 0.9659258262890683122, 1.000000000000000000, 0.9659258262890683122, 1.000000000000000000, 0.9659258262890683122, 1.000000000000000000, 0.9659258262890683122, 1.000000000000000000, 0.9659258262890683122, 1.000000000000000000, 0.9659258262890683122, 1.000000000000000000, 0.9659258262890683122, 1.000000000000000000, 0.9659258262890683122, 1.000000000000000000, 0.9659258262890683122, 1.000000000000000000, 0.9659258262890683122, 1.000000000000000000, 0.9659258262890683122, 1.000000000000000000, 0.9659258262890683122, 1.000000000000000000, 0.9659258262890683122, 1.000000000000000000, 0.9659258262890683122, 1.000000000000000000, 0.9659258262890683122, 1.000000000000000000, 0.9659258262890683122, 1.000000000000000000, 0.9659258262890683122, 1.000000000000000000, 0.9659258262890683122, 1.000000000000000000, 0.9659258262890683122, 1.000000000000000000, 0.9659258262890683122, 1.000000000000000000, 0.9659258262890683122, 1.000000000000000000, 0.9659258262890683122, 1.000000000000000000, 0.9659258262890683122, 1.000000000000000000, 0.9659258262890683122, 1.000000000000000000, 0.9659258262890683122, 1.000000000000000000, 0.9659258262890683122, 1.000000000000000000, 0.9659258262890683122, 1.000000000000000000, 0.9659258262890683122, 1.000000000000000000, 0.9659258262890683122, 1.000000000000000000, 0.9659258262890683122, 1.000000000000000000, 0.9659258262890683122, 1.000000000000000000, 0.9659258262890683122, 1.000000000000000000, 0.9659258262890683122, 1.000000000000000000, 0.9659258262890683122, 1.000000000000000000, 0.9659258262890683122, 1.000000000000000000, 0.9659258262890683122, 1.000000000000000000, 0.9659258262890683122, 1.000000000000000000, 0.9659258262890683122, 1.000000000000000000, 0.9659258262890683122, 1.000000000000000000, 0.9659258262890683122, 1.000000000000000000),
 ( 0.3333333333333333703, 0.3219752754296894559, 0.3333333333333333703, 0.3219752754296894559, 0.3333333333333333703, 0.3219752754296894559, 0.3333333333333333703, 0.3219752754296894559, 0.3333333333333333703, 0.3219752754296894559, 0.3333333333333333703, 0.3219752754296894559, 0.3333333333333333703, 0.3219752754296894559, 0.3333333333333333703, 0.3219752754296894559, 0.3333333333333333703, 0.3219752754296894559, 0.3333333333333333703, 0.3219752754296894559, 0.3333333333333333703, 0.3219752754296894559, 0.3333333333333333703, 0.3219752754296894559, 0.3333333333333333703, 0.3219752754296894559, 0.3333333333333333703, 0.3219752754296894559, 0.3333333333333333703, 0.3219752754296894559, 0.3333333333333333703, 0.3219752754296894559, 0.3333333333333333703, 0.3219752754296894559, 0.3333333333333333703, 0.3219752754296894559, 0.3333333333333333703, 0.3219752754296894559, 0.3333333333333333703, 0.3219752754296894559, 0.3333333333333333703, 0.3219752754296894559, 0.3333333333333333703, 0.3219752754296894559, 0.3333333333333333703, 0.3219752754296894559, 0.3333333333333333703, 0.3219752754296894559, 0.3333333333333333703, 0.3219752754296894559, 0.3333333333333333703, 0.3219752754296894559, 0.3333333333333333703, 0.3219752754296894559, 0.3333333333333333703, 0.3219752754296894559, 0.3333333333333333703, 0.3219752754296894559, 0.3333333333333333703, 0.3219752754296894559, 0.3333333333333333703, 0.3219752754296894559, 0.3333333333333333703, 0.3219752754296894559, 0.3333333333333333703, 0.3219752754296894559, 0.3333333333333333703, 0.3219752754296894559, 0.3333333333333333703, 0.3219752754296894559, 0.3333333333333333703, 0.3219752754296894559, 0.3333333333333333703, 0.3219752754296894559, 0.3333333333333333703, 0.3219752754296894559, 0.3333333333333333703, 0.3219752754296894559, 0.3333333333333333703, 0.3219752754296894559, 0.3333333333333333703, 0.3219752754296894559, 0.3333333333333333703, 0.3219752754296894559, 0.3333333333333333703, 0.3219752754296894559, 0.3333333333333333703, 0.3219752754296894559, 0.3333333333333333703, 0.3219752754296894559, 0.3333333333333333703, 0.3219752754296894559, 0.3333333333333333703, 0.3219752754296894559, 0.3333333333333333703, 0.3219752754296894559, 0.3333333333333333703, 0.3219752754296894559, 0.3333333333333333703, 0.3219752754296894559, 0.3333333333333333703, 0.3219752754296894559, 0.3333333333333333703, 0.3219752754296894559, 0.3333333333333333703, 0.3219752754296894559, 0.3333333333333333703, 0.3219752754296894559, 0.3333333333333333703, 0.3219752754296894559, 0.3333333333333333703, 0.3219752754296894559, 0.3333333333333333703, 0.3219752754296894559, 0.3333333333333333703, 0.3219752754296894559, 0.3333333333333333703, 0.3219752754296894559, 0.3333333333333333703, 0.3219752754296894559, 0.3333333333333333703, 0.3219752754296894559, 0.3333333333333333703, 0.3219752754296894559, 0.3333333333333333703, 0.3219752754296894559, 0.3333333333333333703, 0.3219752754296894559, 0.3333333333333333703, 0.3219752754296894559, 0.3333333333333333703, 0.3219752754296894559, 0.3333333333333333703, 0.3219752754296894559, 0.3333333333333333703, 0.3219752754296894559, 0.3333333333333333703, 0.3219752754296894559, 0.3333333333333333703, 0.3219752754296894559, 0.3333333333333333703, 0.3219752754296894559, 0.3333333333333333703, 0.3219752754296894559, 0.3333333333333333703, 0.3219752754296894559, 0.3333333333333333703, 0.3219752754296894559, 0.3333333333333333703, 0.3219752754296894559, 0.3333333333333333703, 0.3219752754296894559, 0.3333333333333333703, 0.3219752754296894559, 0.3333333333333333703, 0.3219752754296894559, 0.3333333333333333703, 0.3219752754296894559, 0.3333333333333333703, 0.3219752754296894559, 0.3333333333333333703, 0.3219752754296894559, 0.3333333333333333703, 0.3219752754296894559, 0.3333333333333333703, 0.3219752754296894559, 0.3333333333333333703, 0.3219752754296894559, 0.3333333333333333703, 0.3219752754296894559, 0.3333333333333333703, 0.3219752754296894559, 0.3333333333333333703, 0.3219752754296894559, 0.3333333333333333703, 0.3219752754296894559, 0.3333333333333333703, 0.3219752754296894559, 0.3333333333333333703, 0.3219752754296894559, 0.3333333333333333703, 0.3219752754296894559, 0.3333333333333333703, 0.3219752754296894559, 0.3333333333333333703, 0.3219752754296894559, 0.3333333333333333703, 0.3219752754296894559, 0.3333333333333333703, 0.3219752754296894559, 0.3333333333333333703, 0.3219752754296894559, 0.3333333333333333703, 0.3219752754296894559, 0.3333333333333333703, 0.3219752754296894559, 0.3333333333333333703, 0.3219752754296894559, 0.3333333333333333703, 0.3219752754296894559, 0.3333333333333333703, 0.3219752754296894559, 0.3333333333333333703, 0.3219752754296894559, 0.3333333333333333703, 0.3219752754296894559, 0.3333333333333333703, 0.3219752754296894559, 0.3333333333333333703, 0.3219752754296894559, 0.3333333333333333703, 0.3219752754296894559, 0.3333333333333333703, 0.3219752754296894559, 0.3333333333333333703, 0.3219752754296894559, 0.3333333333333333703, 0.3219752754296894559, 0.3333333333333333703, 0.3219752754296894559, 0.3333333333333333703, 0.3219752754296894559, 0.3333333333333333703, 0.3219752754296894559, 0.3333333333333333703, 0.3219752754296894559, 0.3333333333333333703, 0.3219752754296894559, 0.3333333333333333703, 0.3219752754296894559, 0.3333333333333333703, 0.3219752754296894559, 0.3333333333333333703, 0.3219752754296894559, 0.3333333333333333703, 0.3219752754296894559, 0.3333333333333333703, 0.3219752754296894559, 0.3333333333333333703, 0.3219752754296894559, 0.3333333333333333703, 0.3219752754296894559, 0.3333333333333333703, 0.3219752754296894559, 0.3333333333333333703, 0.3219752754296894559, 0.3333333333333333703, 0.3219752754296894559, 0.3333333333333333703, 0.3219752754296894559, 0.3333333333333333703, 0.3219752754296894559, 0.3333333333333333703, 0.3219752754296894559, 0.3333333333333333703, 0.3219752754296894559, 0.3333333333333333703, 0.3219752754296894559, 0.3333333333333333703, 0.3219752754296894559, 0.3333333333333333703, 0.3219752754296894559, 0.3333333333333333703, 0.3219752754296894559, 0.3333333333333333703, 0.3219752754296894559, 0.3333333333333333703, 0.3219752754296894559, 0.3333333333333333703, 0.3219752754296894559, 0.3333333333333333703, 0.3219752754296894559, 0.3333333333333333703, 0.3219752754296894559, 0.3333333333333333703, 0.3219752754296894559, 0.3333333333333333703, 0.3219752754296894559, 0.3333333333333333703, 0.3219752754296894559, 0.3333333333333333703, 0.3219752754296894559, 0.3333333333333333703, 0.3219752754296894559, 0.3333333333333333703, 0.3219752754296894559, 0.3333333333333333703, 0.3219752754296894559, 0.3333333333333333703, 0.3219752754296894559, 0.3333333333333333703, 0.3219752754296894559, 0.3333333333333333703, 0.3219752754296894559, 0.3333333333333333703, 0.3219752754296894559, 0.3333333333333333703, 0.3219752754296894559, 0.3333333333333333703, 0.3219752754296894559, 0.3333333333333333703, 0.3219752754296894559, 0.3333333333333333703, 0.3219752754296894559, 0.3333333333333333703, 0.3219752754296894559, 0.3333333333333333703, 0.3219752754296894559, 0.3333333333333333703, 0.3219752754296894559, 0.3333333333333333703, 0.3219752754296894559, 0.3333333333333333703, 0.3219752754296894559, 0.3333333333333333703, 0.3219752754296894559, 0.3333333333333333703, 0.3219752754296894559, 0.3333333333333333703, 0.3219752754296894559, 0.3333333333333333703, 0.3219752754296894559, 0.3333333333333333703, 0.3219752754296894559, 0.3333333333333333703, 0.3219752754296894559, 0.3333333333333333703, 0.3219752754296894559, 0.3333333333333333703, 0.3219752754296894559, 0.3333333333333333703, 0.3219752754296894559, 0.3333333333333333703, 0.3219752754296894559, 0.3333333333333333703, 0.3219752754296894559, 0.3333333333333333703, 0.3219752754296894559, 0.3333333333333333703, 0.3219752754296894559, 0.3333333333333333703, 0.3219752754296894559, 0.3333333333333333703, 0.3219752754296894559, 0.3333333333333333703, 0.3219752754296894559, 0.3333333333333333703, 0.3219752754296894559, 0.3333333333333333703, 0.3219752754296894559, 0.3333333333333333703, 0.3219752754296894559, 0.3333333333333333703, 0.3219752754296894559, 0.3333333333333333703, 0.3219752754296894559, 0.3333333333333333703, 0.3219752754296894559, 0.3333333333333333703, 0.3219752754296894559, 0.3333333333333333703, 0.3219752754296894559, 0.3333333333333333703, 0.3219752754296894559, 0.3333333333333333703, 0.3219752754296894559, 0.3333333333333333703, 0.3219752754296894559, 0.3333333333333333703, 0.3219752754296894559, 0.3333333333333333703, 0.3219752754296894559, 0.3333333333333333703, 0.3219752754296894559, 0.3333333333333333703, 0.3219752754296894559, 0.3333333333333333703, 0.3219752754296894559, 0.3333333333333333703, 0.3219752754296894559, 0.3333333333333333703, 0.3219752754296894559, 0.3333333333333333703, 0.3219752754296894559, 0.3333333333333333703),
 ( 0.3333333333333333703, 0.3219752754296894559, 0.3333333333333333703, 0.3219752754296894559, 0.3333333333333333703, 0.3219752754296894559, 0.3333333333333333703, 0.3219752754296894559, 0.3333333333333333703, 0.3219752754296894559, 0.3333333333333333703, 0.3219752754296894559, 0.3333333333333333703, 0.3219752754296894559, 0.3333333333333333703, 0.3219752754296894559, 0.3333333333333333703, 0.3219752754296894559, 0.3333333333333333703, 0.3219752754296894559, 0.3333333333333333703, 0.3219752754296894559, 0.3333333333333333703, 0.3219752754296894559, 0.3333333333333333703, 0.3219752754296894559, 0.3333333333333333703, 0.3219752754296894559, 0.3333333333333333703, 0.3219752754296894559, 0.3333333333333333703, 0.3219752754296894559, 0.3333333333333333703, 0.3219752754296894559, 0.3333333333333333703, 0.3219752754296894559, 0.3333333333333333703, 0.3219752754296894559, 0.3333333333333333703, 0.3219752754296894559, 0.3333333333333333703, 0.3219752754296894559, 0.3333333333333333703, 0.3219752754296894559, 0.3333333333333333703, 0.3219752754296894559, 0.3333333333333333703, 0.3219752754296894559, 0.3333333333333333703, 0.3219752754296894559, 0.3333333333333333703, 0.3219752754296894559, 0.3333333333333333703, 0.3219752754296894559, 0.3333333333333333703, 0.3219752754296894559, 0.3333333333333333703, 0.3219752754296894559, 0.3333333333333333703, 0.3219752754296894559, 0.3333333333333333703, 0.3219752754296894559, 0.3333333333333333703, 0.3219752754296894559, 0.3333333333333333703, 0.3219752754296894559, 0.3333333333333333703, 0.3219752754296894559, 0.3333333333333333703, 0.3219752754296894559, 0.3333333333333333703, 0.3219752754296894559, 0.3333333333333333703, 0.3219752754296894559, 0.3333333333333333703, 0.3219752754296894559, 0.3333333333333333703, 0.3219752754296894559, 0.3333333333333333703, 0.3219752754296894559, 0.3333333333333333703, 0.3219752754296894559, 0.3333333333333333703, 0.3219752754296894559, 0.3333333333333333703, 0.3219752754296894559, 0.3333333333333333703, 0.3219752754296894559, 0.3333333333333333703, 0.3219752754296894559, 0.3333333333333333703, 0.3219752754296894559, 0.3333333333333333703, 0.3219752754296894559, 0.3333333333333333703, 0.3219752754296894559, 0.3333333333333333703, 0.3219752754296894559, 0.3333333333333333703, 0.3219752754296894559, 0.3333333333333333703, 0.3219752754296894559, 0.3333333333333333703, 0.3219752754296894559, 0.3333333333333333703, 0.3219752754296894559, 0.3333333333333333703, 0.3219752754296894559, 0.3333333333333333703, 0.3219752754296894559, 0.3333333333333333703, 0.3219752754296894559, 0.3333333333333333703, 0.3219752754296894559, 0.3333333333333333703, 0.3219752754296894559, 0.3333333333333333703, 0.3219752754296894559, 0.3333333333333333703, 0.3219752754296894559, 0.3333333333333333703, 0.3219752754296894559, 0.3333333333333333703, 0.3219752754296894559, 0.3333333333333333703, 0.3219752754296894559, 0.3333333333333333703, 0.3219752754296894559, 0.3333333333333333703, 0.3219752754296894559, 0.3333333333333333703, 0.3219752754296894559, 0.3333333333333333703, 0.3219752754296894559, 0.3333333333333333703, 0.3219752754296894559, 0.3333333333333333703, 0.3219752754296894559, 0.3333333333333333703, 0.3219752754296894559, 0.3333333333333333703, 0.3219752754296894559, 0.3333333333333333703, 0.3219752754296894559, 0.3333333333333333703, 0.3219752754296894559, 0.3333333333333333703, 0.3219752754296894559, 0.3333333333333333703, 0.3219752754296894559, 0.3333333333333333703, 0.3219752754296894559, 0.3333333333333333703, 0.3219752754296894559, 0.3333333333333333703, 0.3219752754296894559, 0.3333333333333333703, 0.3219752754296894559, 0.3333333333333333703, 0.3219752754296894559, 0.3333333333333333703, 0.3219752754296894559, 0.3333333333333333703, 0.3219752754296894559, 0.3333333333333333703, 0.3219752754296894559, 0.3333333333333333703, 0.3219752754296894559, 0.3333333333333333703, 0.3219752754296894559, 0.3333333333333333703, 0.3219752754296894559, 0.3333333333333333703, 0.3219752754296894559, 0.3333333333333333703, 0.3219752754296894559, 0.3333333333333333703, 0.3219752754296894559, 0.3333333333333333703, 0.3219752754296894559, 0.3333333333333333703, 0.3219752754296894559, 0.3333333333333333703, 0.3219752754296894559, 0.3333333333333333703, 0.3219752754296894559, 0.3333333333333333703, 0.3219752754296894559, 0.3333333333333333703, 0.3219752754296894559, 0.3333333333333333703, 0.3219752754296894559, 0.3333333333333333703, 0.3219752754296894559, 0.3333333333333333703, 0.3219752754296894559, 0.3333333333333333703, 0.3219752754296894559, 0.3333333333333333703, 0.3219752754296894559, 0.3333333333333333703, 0.3219752754296894559, 0.3333333333333333703, 0.3219752754296894559, 0.3333333333333333703, 0.3219752754296894559, 0.3333333333333333703, 0.3219752754296894559, 0.3333333333333333703, 0.3219752754296894559, 0.3333333333333333703, 0.3219752754296894559, 0.3333333333333333703, 0.3219752754296894559, 0.3333333333333333703, 0.3219752754296894559, 0.3333333333333333703, 0.3219752754296894559, 0.3333333333333333703, 0.3219752754296894559, 0.3333333333333333703, 0.3219752754296894559, 0.3333333333333333703, 0.3219752754296894559, 0.3333333333333333703, 0.3219752754296894559, 0.3333333333333333703, 0.3219752754296894559, 0.3333333333333333703, 0.3219752754296894559, 0.3333333333333333703, 0.3219752754296894559, 0.3333333333333333703, 0.3219752754296894559, 0.3333333333333333703, 0.3219752754296894559, 0.3333333333333333703, 0.3219752754296894559, 0.3333333333333333703, 0.3219752754296894559, 0.3333333333333333703, 0.3219752754296894559, 0.3333333333333333703, 0.3219752754296894559, 0.3333333333333333703, 0.3219752754296894559, 0.3333333333333333703, 0.3219752754296894559, 0.3333333333333333703, 0.3219752754296894559, 0.3333333333333333703, 0.3219752754296894559, 0.3333333333333333703, 0.3219752754296894559, 0.3333333333333333703, 0.3219752754296894559, 0.3333333333333333703, 0.3219752754296894559, 0.3333333333333333703, 0.3219752754296894559, 0.3333333333333333703, 0.3219752754296894559, 0.3333333333333333703, 0.3219752754296894559, 0.3333333333333333703, 0.3219752754296894559, 0.3333333333333333703, 0.3219752754296894559, 0.3333333333333333703, 0.3219752754296894559, 0.3333333333333333703, 0.3219752754296894559, 0.3333333333333333703, 0.3219752754296894559, 0.3333333333333333703, 0.3219752754296894559, 0.3333333333333333703, 0.3219752754296894559, 0.3333333333333333703, 0.3219752754296894559, 0.3333333333333333703, 0.3219752754296894559, 0.3333333333333333703, 0.3219752754296894559, 0.3333333333333333703, 0.3219752754296894559, 0.3333333333333333703, 0.3219752754296894559, 0.3333333333333333703, 0.3219752754296894559, 0.3333333333333333703, 0.3219752754296894559, 0.3333333333333333703, 0.3219752754296894559, 0.3333333333333333703, 0.3219752754296894559, 0.3333333333333333703, 0.3219752754296894559, 0.3333333333333333703, 0.3219752754296894559, 0.3333333333333333703, 0.3219752754296894559, 0.3333333333333333703, 0.3219752754296894559, 0.3333333333333333703, 0.3219752754296894559, 0.3333333333333333703, 0.3219752754296894559, 0.3333333333333333703, 0.3219752754296894559, 0.3333333333333333703, 0.3219752754296894559, 0.3333333333333333703, 0.3219752754296894559, 0.3333333333333333703, 0.3219752754296894559, 0.3333333333333333703, 0.3219752754296894559, 0.3333333333333333703, 0.3219752754296894559, 0.3333333333333333703, 0.3219752754296894559, 0.3333333333333333703, 0.3219752754296894559, 0.3333333333333333703, 0.3219752754296894559, 0.3333333333333333703, 0.3219752754296894559, 0.3333333333333333703, 0.3219752754296894559, 0.3333333333333333703, 0.3219752754296894559, 0.3333333333333333703, 0.3219752754296894559, 0.3333333333333333703, 0.3219752754296894559, 0.3333333333333333703, 0.3219752754296894559, 0.3333333333333333703, 0.3219752754296894559, 0.3333333333333333703, 0.3219752754296894559, 0.3333333333333333703, 0.3219752754296894559, 0.3333333333333333703, 0.3219752754296894559, 0.3333333333333333703, 0.3219752754296894559, 0.3333333333333333703, 0.3219752754296894559, 0.3333333333333333703, 0.3219752754296894559, 0.3333333333333333703, 0.3219752754296894559, 0.3333333333333333703, 0.3219752754296894559, 0.3333333333333333703, 0.3219752754296894559, 0.3333333333333333703, 0.3219752754296894559, 0.3333333333333333703, 0.3219752754296894559, 0.3333333333333333703, 0.3219752754296894559, 0.3333333333333333703, 0.3219752754296894559, 0.3333333333333333703, 0.3219752754296894559, 0.3333333333333333703, 0.3219752754296894559, 0.3333333333333333703, 0.3219752754296894559, 0.3333333333333333703, 0.3219752754296894559, 0.3333333333333333703, 0.3219752754296894559, 0.3333333333333333703, 0.3219752754296894559, 0.3333333333333333703, 0.3219752754296894559, 0.3333333333333333703, 0.3219752754296894559, 0.3333333333333333703, 0.3219752754296894559, 0.3333333333333333703),
 ( 1.000000000000000000, 0.9659258262890683122, 1.000000000000000000, 0.9659258262890683122, 1.000000000000000000, 0.9659258262890683122, 1.000000000000000000, 0.9659258262890683122, 1.000000000000000000, 0.9659258262890683122, 1.000000000000000000, 0.9659258262890683122, 1.000000000000000000, 0.9659258262890683122, 1.000000000000000000, 0.9659258262890683122, 1.000000000000000000, 0.9659258262890683122, 1.000000000000000000, 0.9659258262890683122, 1.000000000000000000, 0.9659258262890683122, 1.000000000000000000, 0.9659258262890683122, 1.000000000000000000, 0.9659258262890683122, 1.000000000000000000, 0.9659258262890683122, 1.000000000000000000, 0.9659258262890683122, 1.000000000000000000, 0.9659258262890683122, 1.000000000000000000, 0.9659258262890683122, 1.000000000000000000, 0.9659258262890683122, 1.000000000000000000, 0.9659258262890683122, 1.000000000000000000, 0.9659258262890683122, 1.000000000000000000, 0.9659258262890683122, 1.000000000000000000, 0.9659258262890683122, 1.000000000000000000, 0.9659258262890683122, 1.000000000000000000, 0.9659258262890683122, 1.000000000000000000, 0.9659258262890683122, 1.000000000000000000, 0.9659258262890683122, 1.000000000000000000, 0.9659258262890683122, 1.000000000000000000, 0.9659258262890683122, 1.000000000000000000, 0.9659258262890683122, 1.000000000000000000, 0.9659258262890683122, 1.000000000000000000, 0.9659258262890683122, 1.000000000000000000, 0.9659258262890683122, 1.000000000000000000, 0.9659258262890683122, 1.000000000000000000, 0.9659258262890683122, 1.000000000000000000, 0.9659258262890683122, 1.000000000000000000, 0.9659258262890683122, 1.000000000000000000, 0.9659258262890683122, 1.000000000000000000, 0.9659258262890683122, 1.000000000000000000, 0.9659258262890683122, 1.000000000000000000, 0.9659258262890683122, 1.000000000000000000, 0.9659258262890683122, 1.000000000000000000, 0.9659258262890683122, 1.000000000000000000, 0.9659258262890683122, 1.000000000000000000, 0.9659258262890683122, 1.000000000000000000, 0.9659258262890683122, 1.000000000000000000, 0.9659258262890683122, 1.000000000000000000, 0.9659258262890683122, 1.000000000000000000, 0.9659258262890683122, 1.000000000000000000, 0.9659258262890683122, 1.000000000000000000, 0.9659258262890683122, 1.000000000000000000, 0.9659258262890683122, 1.000000000000000000, 0.9659258262890683122, 1.000000000000000000, 0.9659258262890683122, 1.000000000000000000, 0.9659258262890683122, 1.000000000000000000, 0.9659258262890683122, 1.000000000000000000, 0.9659258262890683122, 1.000000000000000000, 0.9659258262890683122, 1.000000000000000000, 0.9659258262890683122, 1.000000000000000000, 0.9659258262890683122, 1.000000000000000000, 0.9659258262890683122, 1.000000000000000000, 0.9659258262890683122, 1.000000000000000000, 0.9659258262890683122, 1.000000000000000000, 0.9659258262890683122, 1.000000000000000000, 0.9659258262890683122, 1.000000000000000000, 0.9659258262890683122, 1.000000000000000000, 0.9659258262890683122, 1.000000000000000000, 0.9659258262890683122, 1.000000000000000000, 0.9659258262890683122, 1.000000000000000000, 0.9659258262890683122, 1.000000000000000000, 0.9659258262890683122, 1.000000000000000000, 0.9659258262890683122, 1.000000000000000000, 0.9659258262890683122, 1.000000000000000000, 0.9659258262890683122, 1.000000000000000000, 0.9659258262890683122, 1.000000000000000000, 0.9659258262890683122, 1.000000000000000000, 0.9659258262890683122, 1.000000000000000000, 0.9659258262890683122, 1.000000000000000000, 0.9659258262890683122, 1.000000000000000000, 0.9659258262890683122, 1.000000000000000000, 0.9659258262890683122, 1.000000000000000000, 0.9659258262890683122, 1.000000000000000000, 0.9659258262890683122, 1.000000000000000000, 0.9659258262890683122, 1.000000000000000000, 0.9659258262890683122, 1.000000000000000000, 0.9659258262890683122, 1.000000000000000000, 0.9659258262890683122, 1.000000000000000000, 0.9659258262890683122, 1.000000000000000000, 0.9659258262890683122, 1.000000000000000000, 0.9659258262890683122, 1.000000000000000000, 0.9659258262890683122, 1.000000000000000000, 0.9659258262890683122, 1.000000000000000000, 0.9659258262890683122, 1.000000000000000000, 0.9659258262890683122, 1.000000000000000000, 0.9659258262890683122, 1.000000000000000000, 0.9659258262890683122, 1.000000000000000000, 0.9659258262890683122, 1.000000000000000000, 0.9659258262890683122, 1.000000000000000000, 0.9659258262890683122, 1.000000000000000000, 0.9659258262890683122, 1.000000000000000000, 0.9659258262890683122, 1.000000000000000000, 0.9659258262890683122, 1.000000000000000000, 0.9659258262890683122, 1.000000000000000000, 0.9659258262890683122, 1.000000000000000000, 0.9659258262890683122, 1.000000000000000000, 0.9659258262890683122, 1.000000000000000000, 0.9659258262890683122, 1.000000000000000000, 0.9659258262890683122, 1.000000000000000000, 0.9659258262890683122, 1.000000000000000000, 0.9659258262890683122, 1.000000000000000000, 0.9659258262890683122, 1.000000000000000000, 0.9659258262890683122, 1.000000000000000000, 0.9659258262890683122, 1.000000000000000000, 0.9659258262890683122, 1.000000000000000000, 0.9659258262890683122, 1.000000000000000000, 0.9659258262890683122, 1.000000000000000000, 0.9659258262890683122, 1.000000000000000000, 0.9659258262890683122, 1.000000000000000000, 0.9659258262890683122, 1.000000000000000000, 0.9659258262890683122, 1.000000000000000000, 0.9659258262890683122, 1.000000000000000000, 0.9659258262890683122, 1.000000000000000000, 0.9659258262890683122, 1.000000000000000000, 0.9659258262890683122, 1.000000000000000000, 0.9659258262890683122, 1.000000000000000000, 0.9659258262890683122, 1.000000000000000000, 0.9659258262890683122, 1.000000000000000000, 0.9659258262890683122, 1.000000000000000000, 0.9659258262890683122, 1.000000000000000000, 0.9659258262890683122, 1.000000000000000000, 0.9659258262890683122, 1.000000000000000000, 0.9659258262890683122, 1.000000000000000000, 0.9659258262890683122, 1.000000000000000000, 0.9659258262890683122, 1.000000000000000000, 0.9659258262890683122, 1.000000000000000000, 0.9659258262890683122, 1.000000000000000000, 0.9659258262890683122, 1.000000000000000000, 0.9659258262890683122, 1.000000000000000000, 0.9659258262890683122, 1.000000000000000000, 0.9659258262890683122, 1.000000000000000000, 0.9659258262890683122, 1.000000000000000000, 0.9659258262890683122, 1.000000000000000000, 0.9659258262890683122, 1.000000000000000000, 0.9659258262890683122, 1.000000000000000000, 0.9659258262890683122, 1.000000000000000000, 0.9659258262890683122, 1.000000000000000000, 0.9659258262890683122, 1.000000000000000000, 0.9659258262890683122, 1.000000000000000000, 0.9659258262890683122, 1.000000000000000000, 0.9659258262890683122, 1.000000000000000000, 0.9659258262890683122, 1.000000000000000000, 0.9659258262890683122, 1.000000000000000000, 0.9659258262890683122, 1.000000000000000000, 0.9659258262890683122, 1.000000000000000000, 0.9659258262890683122, 1.000000000000000000, 0.9659258262890683122, 1.000000000000000000, 0.9659258262890683122, 1.000000000000000000, 0.9659258262890683122, 1.000000000000000000, 0.9659258262890683122, 1.000000000000000000, 0.9659258262890683122, 1.000000000000000000, 0.9659258262890683122, 1.000000000000000000, 0.9659258262890683122, 1.000000000000000000, 0.9659258262890683122, 1.000000000000000000, 0.9659258262890683122, 1.000000000000000000, 0.9659258262890683122, 1.000000000000000000, 0.9659258262890683122, 1.000000000000000000, 0.9659258262890683122, 1.000000000000000000, 0.9659258262890683122, 1.000000000000000000, 0.9659258262890683122, 1.000000000000000000, 0.9659258262890683122, 1.000000000000000000, 0.9659258262890683122, 1.000000000000000000, 0.9659258262890683122, 1.000000000000000000, 0.9659258262890683122, 1.000000000000000000, 0.9659258262890683122, 1.000000000000000000, 0.9659258262890683122, 1.000000000000000000, 0.9659258262890683122, 1.000000000000000000, 0.9659258262890683122, 1.000000000000000000, 0.9659258262890683122, 1.000000000000000000, 0.9659258262890683122, 1.000000000000000000, 0.9659258262890683122, 1.000000000000000000, 0.9659258262890683122, 1.000000000000000000, 0.9659258262890683122, 1.000000000000000000, 0.9659258262890683122, 1.000000000000000000, 0.9659258262890683122, 1.000000000000000000, 0.9659258262890683122, 1.000000000000000000, 0.9659258262890683122, 1.000000000000000000, 0.9659258262890683122, 1.000000000000000000, 0.9659258262890683122, 1.000000000000000000, 0.9659258262890683122, 1.000000000000000000, 0.9659258262890683122, 1.000000000000000000, 0.9659258262890683122, 1.000000000000000000, 0.9659258262890683122, 1.000000000000000000, 0.9659258262890683122, 1.000000000000000000),
 ( 0.3333333333333333703, 0.3219752754296894559, 0.3333333333333333703, 0.3219752754296894559, 0.3333333333333333703, 0.3219752754296894559, 0.3333333333333333703, 0.3219752754296894559, 0.3333333333333333703, 0.3219752754296894559, 0.3333333333333333703, 0.3219752754296894559, 0.3333333333333333703, 0.3219752754296894559, 0.3333333333333333703, 0.3219752754296894559, 0.3333333333333333703, 0.3219752754296894559, 0.3333333333333333703, 0.3219752754296894559, 0.3333333333333333703, 0.3219752754296894559, 0.3333333333333333703, 0.3219752754296894559, 0.3333333333333333703, 0.3219752754296894559, 0.3333333333333333703, 0.3219752754296894559, 0.3333333333333333703, 0.3219752754296894559, 0.3333333333333333703, 0.3219752754296894559, 0.3333333333333333703, 0.3219752754296894559, 0.3333333333333333703, 0.3219752754296894559, 0.3333333333333333703, 0.3219752754296894559, 0.3333333333333333703, 0.3219752754296894559, 0.3333333333333333703, 0.3219752754296894559, 0.3333333333333333703, 0.3219752754296894559, 0.3333333333333333703, 0.3219752754296894559, 0.3333333333333333703, 0.3219752754296894559, 0.3333333333333333703, 0.3219752754296894559, 0.3333333333333333703, 0.3219752754296894559, 0.3333333333333333703, 0.3219752754296894559, 0.3333333333333333703, 0.3219752754296894559, 0.3333333333333333703, 0.3219752754296894559, 0.3333333333333333703, 0.3219752754296894559, 0.3333333333333333703, 0.3219752754296894559, 0.3333333333333333703, 0.3219752754296894559, 0.3333333333333333703, 0.3219752754296894559, 0.3333333333333333703, 0.3219752754296894559, 0.3333333333333333703, 0.3219752754296894559, 0.3333333333333333703, 0.3219752754296894559, 0.3333333333333333703, 0.3219752754296894559, 0.3333333333333333703, 0.3219752754296894559, 0.3333333333333333703, 0.3219752754296894559, 0.3333333333333333703, 0.3219752754296894559, 0.3333333333333333703, 0.3219752754296894559, 0.3333333333333333703, 0.3219752754296894559, 0.3333333333333333703, 0.3219752754296894559, 0.3333333333333333703, 0.3219752754296894559, 0.3333333333333333703, 0.3219752754296894559, 0.3333333333333333703, 0.3219752754296894559, 0.3333333333333333703, 0.3219752754296894559, 0.3333333333333333703, 0.3219752754296894559, 0.3333333333333333703, 0.3219752754296894559, 0.3333333333333333703, 0.3219752754296894559, 0.3333333333333333703, 0.3219752754296894559, 0.3333333333333333703, 0.3219752754296894559, 0.3333333333333333703, 0.3219752754296894559, 0.3333333333333333703, 0.3219752754296894559, 0.3333333333333333703, 0.3219752754296894559, 0.3333333333333333703, 0.3219752754296894559, 0.3333333333333333703, 0.3219752754296894559, 0.3333333333333333703, 0.3219752754296894559, 0.3333333333333333703, 0.3219752754296894559, 0.3333333333333333703, 0.3219752754296894559, 0.3333333333333333703, 0.3219752754296894559, 0.3333333333333333703, 0.3219752754296894559, 0.3333333333333333703, 0.3219752754296894559, 0.3333333333333333703, 0.3219752754296894559, 0.3333333333333333703, 0.3219752754296894559, 0.3333333333333333703, 0.3219752754296894559, 0.3333333333333333703, 0.3219752754296894559, 0.3333333333333333703, 0.3219752754296894559, 0.3333333333333333703, 0.3219752754296894559, 0.3333333333333333703, 0.3219752754296894559, 0.3333333333333333703, 0.3219752754296894559, 0.3333333333333333703, 0.3219752754296894559, 0.3333333333333333703, 0.3219752754296894559, 0.3333333333333333703, 0.3219752754296894559, 0.3333333333333333703, 0.3219752754296894559, 0.3333333333333333703, 0.3219752754296894559, 0.3333333333333333703, 0.3219752754296894559, 0.3333333333333333703, 0.3219752754296894559, 0.3333333333333333703, 0.3219752754296894559, 0.3333333333333333703, 0.3219752754296894559, 0.3333333333333333703, 0.3219752754296894559, 0.3333333333333333703, 0.3219752754296894559, 0.3333333333333333703, 0.3219752754296894559, 0.3333333333333333703, 0.3219752754296894559, 0.3333333333333333703, 0.3219752754296894559, 0.3333333333333333703, 0.3219752754296894559, 0.3333333333333333703, 0.3219752754296894559, 0.3333333333333333703, 0.3219752754296894559, 0.3333333333333333703, 0.3219752754296894559, 0.3333333333333333703, 0.3219752754296894559, 0.3333333333333333703, 0.3219752754296894559, 0.3333333333333333703, 0.3219752754296894559, 0.3333333333333333703, 0.3219752754296894559, 0.3333333333333333703, 0.3219752754296894559, 0.3333333333333333703, 0.3219752754296894559, 0.3333333333333333703, 0.3219752754296894559, 0.3333333333333333703, 0.3219752754296894559, 0.3333333333333333703, 0.3219752754296894559, 0.3333333333333333703, 0.3219752754296894559, 0.3333333333333333703, 0.3219752754296894559, 0.3333333333333333703, 0.3219752754296894559, 0.3333333333333333703, 0.3219752754296894559, 0.3333333333333333703, 0.3219752754296894559, 0.3333333333333333703, 0.3219752754296894559, 0.3333333333333333703, 0.3219752754296894559, 0.3333333333333333703, 0.3219752754296894559, 0.3333333333333333703, 0.3219752754296894559, 0.3333333333333333703, 0.3219752754296894559, 0.3333333333333333703, 0.3219752754296894559, 0.3333333333333333703, 0.3219752754296894559, 0.3333333333333333703, 0.3219752754296894559, 0.3333333333333333703, 0.3219752754296894559, 0.3333333333333333703, 0.3219752754296894559, 0.3333333333333333703, 0.3219752754296894559, 0.3333333333333333703, 0.3219752754296894559, 0.3333333333333333703, 0.3219752754296894559, 0.3333333333333333703, 0.3219752754296894559, 0.3333333333333333703, 0.3219752754296894559, 0.3333333333333333703, 0.3219752754296894559, 0.3333333333333333703, 0.3219752754296894559, 0.3333333333333333703, 0.3219752754296894559, 0.3333333333333333703, 0.3219752754296894559, 0.3333333333333333703, 0.3219752754296894559, 0.3333333333333333703, 0.3219752754296894559, 0.3333333333333333703, 0.3219752754296894559, 0.3333333333333333703, 0.3219752754296894559, 0.3333333333333333703, 0.3219752754296894559, 0.3333333333333333703, 0.3219752754296894559, 0.3333333333333333703, 0.3219752754296894559, 0.3333333333333333703, 0.3219752754296894559, 0.3333333333333333703, 0.3219752754296894559, 0.3333333333333333703, 0.3219752754296894559, 0.3333333333333333703, 0.3219752754296894559, 0.3333333333333333703, 0.3219752754296894559, 0.3333333333333333703, 0.3219752754296894559, 0.3333333333333333703, 0.3219752754296894559, 0.3333333333333333703, 0.3219752754296894559, 0.3333333333333333703, 0.3219752754296894559, 0.3333333333333333703, 0.3219752754296894559, 0.3333333333333333703, 0.3219752754296894559, 0.3333333333333333703, 0.3219752754296894559, 0.3333333333333333703, 0.3219752754296894559, 0.3333333333333333703, 0.3219752754296894559, 0.3333333333333333703, 0.3219752754296894559, 0.3333333333333333703, 0.3219752754296894559, 0.3333333333333333703, 0.3219752754296894559, 0.3333333333333333703, 0.3219752754296894559, 0.3333333333333333703, 0.3219752754296894559, 0.3333333333333333703, 0.3219752754296894559, 0.3333333333333333703, 0.3219752754296894559, 0.3333333333333333703, 0.3219752754296894559, 0.3333333333333333703, 0.3219752754296894559, 0.3333333333333333703, 0.3219752754296894559, 0.3333333333333333703, 0.3219752754296894559, 0.3333333333333333703, 0.3219752754296894559, 0.3333333333333333703, 0.3219752754296894559, 0.3333333333333333703, 0.3219752754296894559, 0.3333333333333333703, 0.3219752754296894559, 0.3333333333333333703, 0.3219752754296894559, 0.3333333333333333703, 0.3219752754296894559, 0.3333333333333333703, 0.3219752754296894559, 0.3333333333333333703, 0.3219752754296894559, 0.3333333333333333703, 0.3219752754296894559, 0.3333333333333333703, 0.3219752754296894559, 0.3333333333333333703, 0.3219752754296894559, 0.3333333333333333703, 0.3219752754296894559, 0.3333333333333333703, 0.3219752754296894559, 0.3333333333333333703, 0.3219752754296894559, 0.3333333333333333703, 0.3219752754296894559, 0.3333333333333333703, 0.3219752754296894559, 0.3333333333333333703, 0.3219752754296894559, 0.3333333333333333703, 0.3219752754296894559, 0.3333333333333333703, 0.3219752754296894559, 0.3333333333333333703, 0.3219752754296894559, 0.3333333333333333703, 0.3219752754296894559, 0.3333333333333333703, 0.3219752754296894559, 0.3333333333333333703, 0.3219752754296894559, 0.3333333333333333703, 0.3219752754296894559, 0.3333333333333333703, 0.3219752754296894559, 0.3333333333333333703, 0.3219752754296894559, 0.3333333333333333703, 0.3219752754296894559, 0.3333333333333333703, 0.3219752754296894559, 0.3333333333333333703, 0.3219752754296894559, 0.3333333333333333703, 0.3219752754296894559, 0.3333333333333333703, 0.3219752754296894559, 0.3333333333333333703, 0.3219752754296894559, 0.3333333333333333703, 0.3219752754296894559, 0.3333333333333333703, 0.3219752754296894559, 0.3333333333333333703, 0.3219752754296894559, 0.3333333333333333703, 0.3219752754296894559, 0.3333333333333333703, 0.3219752754296894559, 0.3333333333333333703, 0.3219752754296894559, 0.3333333333333333703),
 ( 0.3333333333333333703, 0.3219752754296894559, 0.3333333333333333703, 0.3219752754296894559, 0.3333333333333333703, 0.3219752754296894559, 0.3333333333333333703, 0.3219752754296894559, 0.3333333333333333703, 0.3219752754296894559, 0.3333333333333333703, 0.3219752754296894559, 0.3333333333333333703, 0.3219752754296894559, 0.3333333333333333703, 0.3219752754296894559, 0.3333333333333333703, 0.3219752754296894559, 0.3333333333333333703, 0.3219752754296894559, 0.3333333333333333703, 0.3219752754296894559, 0.3333333333333333703, 0.3219752754296894559, 0.3333333333333333703, 0.3219752754296894559, 0.3333333333333333703, 0.3219752754296894559, 0.3333333333333333703, 0.3219752754296894559, 0.3333333333333333703, 0.3219752754296894559, 0.3333333333333333703, 0.3219752754296894559, 0.3333333333333333703, 0.3219752754296894559, 0.3333333333333333703, 0.3219752754296894559, 0.3333333333333333703, 0.3219752754296894559, 0.3333333333333333703, 0.3219752754296894559, 0.3333333333333333703, 0.3219752754296894559, 0.3333333333333333703, 0.3219752754296894559, 0.3333333333333333703, 0.3219752754296894559, 0.3333333333333333703, 0.3219752754296894559, 0.3333333333333333703, 0.3219752754296894559, 0.3333333333333333703, 0.3219752754296894559, 0.3333333333333333703, 0.3219752754296894559, 0.3333333333333333703, 0.3219752754296894559, 0.3333333333333333703, 0.3219752754296894559, 0.3333333333333333703, 0.3219752754296894559, 0.3333333333333333703, 0.3219752754296894559, 0.3333333333333333703, 0.3219752754296894559, 0.3333333333333333703, 0.3219752754296894559, 0.3333333333333333703, 0.3219752754296894559, 0.3333333333333333703, 0.3219752754296894559, 0.3333333333333333703, 0.3219752754296894559, 0.3333333333333333703, 0.3219752754296894559, 0.3333333333333333703, 0.3219752754296894559, 0.3333333333333333703, 0.3219752754296894559, 0.3333333333333333703, 0.3219752754296894559, 0.3333333333333333703, 0.3219752754296894559, 0.3333333333333333703, 0.3219752754296894559, 0.3333333333333333703, 0.3219752754296894559, 0.3333333333333333703, 0.3219752754296894559, 0.3333333333333333703, 0.3219752754296894559, 0.3333333333333333703, 0.3219752754296894559, 0.3333333333333333703, 0.3219752754296894559, 0.3333333333333333703, 0.3219752754296894559, 0.3333333333333333703, 0.3219752754296894559, 0.3333333333333333703, 0.3219752754296894559, 0.3333333333333333703, 0.3219752754296894559, 0.3333333333333333703, 0.3219752754296894559, 0.3333333333333333703, 0.3219752754296894559, 0.3333333333333333703, 0.3219752754296894559, 0.3333333333333333703, 0.3219752754296894559, 0.3333333333333333703, 0.3219752754296894559, 0.3333333333333333703, 0.3219752754296894559, 0.3333333333333333703, 0.3219752754296894559, 0.3333333333333333703, 0.3219752754296894559, 0.3333333333333333703, 0.3219752754296894559, 0.3333333333333333703, 0.3219752754296894559, 0.3333333333333333703, 0.3219752754296894559, 0.3333333333333333703, 0.3219752754296894559, 0.3333333333333333703, 0.3219752754296894559, 0.3333333333333333703, 0.3219752754296894559, 0.3333333333333333703, 0.3219752754296894559, 0.3333333333333333703, 0.3219752754296894559, 0.3333333333333333703, 0.3219752754296894559, 0.3333333333333333703, 0.3219752754296894559, 0.3333333333333333703, 0.3219752754296894559, 0.3333333333333333703, 0.3219752754296894559, 0.3333333333333333703, 0.3219752754296894559, 0.3333333333333333703, 0.3219752754296894559, 0.3333333333333333703, 0.3219752754296894559, 0.3333333333333333703, 0.3219752754296894559, 0.3333333333333333703, 0.3219752754296894559, 0.3333333333333333703, 0.3219752754296894559, 0.3333333333333333703, 0.3219752754296894559, 0.3333333333333333703, 0.3219752754296894559, 0.3333333333333333703, 0.3219752754296894559, 0.3333333333333333703, 0.3219752754296894559, 0.3333333333333333703, 0.3219752754296894559, 0.3333333333333333703, 0.3219752754296894559, 0.3333333333333333703, 0.3219752754296894559, 0.3333333333333333703, 0.3219752754296894559, 0.3333333333333333703, 0.3219752754296894559, 0.3333333333333333703, 0.3219752754296894559, 0.3333333333333333703, 0.3219752754296894559, 0.3333333333333333703, 0.3219752754296894559, 0.3333333333333333703, 0.3219752754296894559, 0.3333333333333333703, 0.3219752754296894559, 0.3333333333333333703, 0.3219752754296894559, 0.3333333333333333703, 0.3219752754296894559, 0.3333333333333333703, 0.3219752754296894559, 0.3333333333333333703, 0.3219752754296894559, 0.3333333333333333703, 0.3219752754296894559, 0.3333333333333333703, 0.3219752754296894559, 0.3333333333333333703, 0.3219752754296894559, 0.3333333333333333703, 0.3219752754296894559, 0.3333333333333333703, 0.3219752754296894559, 0.3333333333333333703, 0.3219752754296894559, 0.3333333333333333703, 0.3219752754296894559, 0.3333333333333333703, 0.3219752754296894559, 0.3333333333333333703, 0.3219752754296894559, 0.3333333333333333703, 0.3219752754296894559, 0.3333333333333333703, 0.3219752754296894559, 0.3333333333333333703, 0.3219752754296894559, 0.3333333333333333703, 0.3219752754296894559, 0.3333333333333333703, 0.3219752754296894559, 0.3333333333333333703, 0.3219752754296894559, 0.3333333333333333703, 0.3219752754296894559, 0.3333333333333333703, 0.3219752754296894559, 0.3333333333333333703, 0.3219752754296894559, 0.3333333333333333703, 0.3219752754296894559, 0.3333333333333333703, 0.3219752754296894559, 0.3333333333333333703, 0.3219752754296894559, 0.3333333333333333703, 0.3219752754296894559, 0.3333333333333333703, 0.3219752754296894559, 0.3333333333333333703, 0.3219752754296894559, 0.3333333333333333703, 0.3219752754296894559, 0.3333333333333333703, 0.3219752754296894559, 0.3333333333333333703, 0.3219752754296894559, 0.3333333333333333703, 0.3219752754296894559, 0.3333333333333333703, 0.3219752754296894559, 0.3333333333333333703, 0.3219752754296894559, 0.3333333333333333703, 0.3219752754296894559, 0.3333333333333333703, 0.3219752754296894559, 0.3333333333333333703, 0.3219752754296894559, 0.3333333333333333703, 0.3219752754296894559, 0.3333333333333333703, 0.3219752754296894559, 0.3333333333333333703, 0.3219752754296894559, 0.3333333333333333703, 0.3219752754296894559, 0.3333333333333333703, 0.3219752754296894559, 0.3333333333333333703, 0.3219752754296894559, 0.3333333333333333703, 0.3219752754296894559, 0.3333333333333333703, 0.3219752754296894559, 0.3333333333333333703, 0.3219752754296894559, 0.3333333333333333703, 0.3219752754296894559, 0.3333333333333333703, 0.3219752754296894559, 0.3333333333333333703, 0.3219752754296894559, 0.3333333333333333703, 0.3219752754296894559, 0.3333333333333333703, 0.3219752754296894559, 0.3333333333333333703, 0.3219752754296894559, 0.3333333333333333703, 0.3219752754296894559, 0.3333333333333333703, 0.3219752754296894559, 0.3333333333333333703, 0.3219752754296894559, 0.3333333333333333703, 0.3219752754296894559, 0.3333333333333333703, 0.3219752754296894559, 0.3333333333333333703, 0.3219752754296894559, 0.3333333333333333703, 0.3219752754296894559, 0.3333333333333333703, 0.3219752754296894559, 0.3333333333333333703, 0.3219752754296894559, 0.3333333333333333703, 0.3219752754296894559, 0.3333333333333333703, 0.3219752754296894559, 0.3333333333333333703, 0.3219752754296894559, 0.3333333333333333703, 0.3219752754296894559, 0.3333333333333333703, 0.3219752754296894559, 0.3333333333333333703, 0.3219752754296894559, 0.3333333333333333703, 0.3219752754296894559, 0.3333333333333333703, 0.3219752754296894559, 0.3333333333333333703, 0.3219752754296894559, 0.3333333333333333703, 0.3219752754296894559, 0.3333333333333333703, 0.3219752754296894559, 0.3333333333333333703, 0.3219752754296894559, 0.3333333333333333703, 0.3219752754296894559, 0.3333333333333333703, 0.3219752754296894559, 0.3333333333333333703, 0.3219752754296894559, 0.3333333333333333703, 0.3219752754296894559, 0.3333333333333333703, 0.3219752754296894559, 0.3333333333333333703, 0.3219752754296894559, 0.3333333333333333703, 0.3219752754296894559, 0.3333333333333333703, 0.3219752754296894559, 0.3333333333333333703, 0.3219752754296894559, 0.3333333333333333703, 0.3219752754296894559, 0.3333333333333333703, 0.3219752754296894559, 0.3333333333333333703, 0.3219752754296894559, 0.3333333333333333703, 0.3219752754296894559, 0.3333333333333333703, 0.3219752754296894559, 0.3333333333333333703, 0.3219752754296894559, 0.3333333333333333703, 0.3219752754296894559, 0.3333333333333333703, 0.3219752754296894559, 0.3333333333333333703, 0.3219752754296894559, 0.3333333333333333703, 0.3219752754296894559, 0.3333333333333333703, 0.3219752754296894559, 0.3333333333333333703, 0.3219752754296894559, 0.3333333333333333703, 0.3219752754296894559, 0.3333333333333333703, 0.3219752754296894559, 0.3333333333333333703, 0.3219752754296894559, 0.3333333333333333703, 0.3219752754296894559, 0.3333333333333333703, 0.3219752754296894559, 0.3333333333333333703, 0.3219752754296894559, 0.3333333333333333703),
 ( 1.000000000000000000, 0.9659258262890683122, 1.000000000000000000, 0.9659258262890683122, 1.000000000000000000, 0.9659258262890683122, 1.000000000000000000, 0.9659258262890683122, 1.000000000000000000, 0.9659258262890683122, 1.000000000000000000, 0.9659258262890683122, 1.000000000000000000, 0.9659258262890683122, 1.000000000000000000, 0.9659258262890683122, 1.000000000000000000, 0.9659258262890683122, 1.000000000000000000, 0.9659258262890683122, 1.000000000000000000, 0.9659258262890683122, 1.000000000000000000, 0.9659258262890683122, 1.000000000000000000, 0.9659258262890683122, 1.000000000000000000, 0.9659258262890683122, 1.000000000000000000, 0.9659258262890683122, 1.000000000000000000, 0.9659258262890683122, 1.000000000000000000, 0.9659258262890683122, 1.000000000000000000, 0.9659258262890683122, 1.000000000000000000, 0.9659258262890683122, 1.000000000000000000, 0.9659258262890683122, 1.000000000000000000, 0.9659258262890683122, 1.000000000000000000, 0.9659258262890683122, 1.000000000000000000, 0.9659258262890683122, 1.000000000000000000, 0.9659258262890683122, 1.000000000000000000, 0.9659258262890683122, 1.000000000000000000, 0.9659258262890683122, 1.000000000000000000, 0.9659258262890683122, 1.000000000000000000, 0.9659258262890683122, 1.000000000000000000, 0.9659258262890683122, 1.000000000000000000, 0.9659258262890683122, 1.000000000000000000, 0.9659258262890683122, 1.000000000000000000, 0.9659258262890683122, 1.000000000000000000, 0.9659258262890683122, 1.000000000000000000, 0.9659258262890683122, 1.000000000000000000, 0.9659258262890683122, 1.000000000000000000, 0.9659258262890683122, 1.000000000000000000, 0.9659258262890683122, 1.000000000000000000, 0.9659258262890683122, 1.000000000000000000, 0.9659258262890683122, 1.000000000000000000, 0.9659258262890683122, 1.000000000000000000, 0.9659258262890683122, 1.000000000000000000, 0.9659258262890683122, 1.000000000000000000, 0.9659258262890683122, 1.000000000000000000, 0.9659258262890683122, 1.000000000000000000, 0.9659258262890683122, 1.000000000000000000, 0.9659258262890683122, 1.000000000000000000, 0.9659258262890683122, 1.000000000000000000, 0.9659258262890683122, 1.000000000000000000, 0.9659258262890683122, 1.000000000000000000, 0.9659258262890683122, 1.000000000000000000, 0.9659258262890683122, 1.000000000000000000, 0.9659258262890683122, 1.000000000000000000, 0.9659258262890683122, 1.000000000000000000, 0.9659258262890683122, 1.000000000000000000, 0.9659258262890683122, 1.000000000000000000, 0.9659258262890683122, 1.000000000000000000, 0.9659258262890683122, 1.000000000000000000, 0.9659258262890683122, 1.000000000000000000, 0.9659258262890683122, 1.000000000000000000, 0.9659258262890683122, 1.000000000000000000, 0.9659258262890683122, 1.000000000000000000, 0.9659258262890683122, 1.000000000000000000, 0.9659258262890683122, 1.000000000000000000, 0.9659258262890683122, 1.000000000000000000, 0.9659258262890683122, 1.000000000000000000, 0.9659258262890683122, 1.000000000000000000, 0.9659258262890683122, 1.000000000000000000, 0.9659258262890683122, 1.000000000000000000, 0.9659258262890683122, 1.000000000000000000, 0.9659258262890683122, 1.000000000000000000, 0.9659258262890683122, 1.000000000000000000, 0.9659258262890683122, 1.000000000000000000, 0.9659258262890683122, 1.000000000000000000, 0.9659258262890683122, 1.000000000000000000, 0.9659258262890683122, 1.000000000000000000, 0.9659258262890683122, 1.000000000000000000, 0.9659258262890683122, 1.000000000000000000, 0.9659258262890683122, 1.000000000000000000, 0.9659258262890683122, 1.000000000000000000, 0.9659258262890683122, 1.000000000000000000, 0.9659258262890683122, 1.000000000000000000, 0.9659258262890683122, 1.000000000000000000, 0.9659258262890683122, 1.000000000000000000, 0.9659258262890683122, 1.000000000000000000, 0.9659258262890683122, 1.000000000000000000, 0.9659258262890683122, 1.000000000000000000, 0.9659258262890683122, 1.000000000000000000, 0.9659258262890683122, 1.000000000000000000, 0.9659258262890683122, 1.000000000000000000, 0.9659258262890683122, 1.000000000000000000, 0.9659258262890683122, 1.000000000000000000, 0.9659258262890683122, 1.000000000000000000, 0.9659258262890683122, 1.000000000000000000, 0.9659258262890683122, 1.000000000000000000, 0.9659258262890683122, 1.000000000000000000, 0.9659258262890683122, 1.000000000000000000, 0.9659258262890683122, 1.000000000000000000, 0.9659258262890683122, 1.000000000000000000, 0.9659258262890683122, 1.000000000000000000, 0.9659258262890683122, 1.000000000000000000, 0.9659258262890683122, 1.000000000000000000, 0.9659258262890683122, 1.000000000000000000, 0.9659258262890683122, 1.000000000000000000, 0.9659258262890683122, 1.000000000000000000, 0.9659258262890683122, 1.000000000000000000, 0.9659258262890683122, 1.000000000000000000, 0.9659258262890683122, 1.000000000000000000, 0.9659258262890683122, 1.000000000000000000, 0.9659258262890683122, 1.000000000000000000, 0.9659258262890683122, 1.000000000000000000, 0.9659258262890683122, 1.000000000000000000, 0.9659258262890683122, 1.000000000000000000, 0.9659258262890683122, 1.000000000000000000, 0.9659258262890683122, 1.000000000000000000, 0.9659258262890683122, 1.000000000000000000, 0.9659258262890683122, 1.000000000000000000, 0.9659258262890683122, 1.000000000000000000, 0.9659258262890683122, 1.000000000000000000, 0.9659258262890683122, 1.000000000000000000, 0.9659258262890683122, 1.000000000000000000, 0.9659258262890683122, 1.000000000000000000, 0.9659258262890683122, 1.000000000000000000, 0.9659258262890683122, 1.000000000000000000, 0.9659258262890683122, 1.000000000000000000, 0.9659258262890683122, 1.000000000000000000, 0.9659258262890683122, 1.000000000000000000, 0.9659258262890683122, 1.000000000000000000, 0.9659258262890683122, 1.000000000000000000, 0.9659258262890683122, 1.000000000000000000, 0.9659258262890683122, 1.000000000000000000, 0.9659258262890683122, 1.000000000000000000, 0.9659258262890683122, 1.000000000000000000, 0.9659258262890683122, 1.000000000000000000, 0.9659258262890683122, 1.000000000000000000, 0.9659258262890683122, 1.000000000000000000, 0.9659258262890683122, 1.000000000000000000, 0.9659258262890683122, 1.000000000000000000, 0.9659258262890683122, 1.000000000000000000, 0.9659258262890683122, 1.000000000000000000, 0.9659258262890683122, 1.000000000000000000, 0.9659258262890683122, 1.000000000000000000, 0.9659258262890683122, 1.000000000000000000, 0.9659258262890683122, 1.000000000000000000, 0.9659258262890683122, 1.000000000000000000, 0.9659258262890683122, 1.000000000000000000, 0.9659258262890683122, 1.000000000000000000, 0.9659258262890683122, 1.000000000000000000, 0.9659258262890683122, 1.000000000000000000, 0.9659258262890683122, 1.000000000000000000, 0.9659258262890683122, 1.000000000000000000, 0.9659258262890683122, 1.000000000000000000, 0.9659258262890683122, 1.000000000000000000, 0.9659258262890683122, 1.000000000000000000, 0.9659258262890683122, 1.000000000000000000, 0.9659258262890683122, 1.000000000000000000, 0.9659258262890683122, 1.000000000000000000, 0.9659258262890683122, 1.000000000000000000, 0.9659258262890683122, 1.000000000000000000, 0.9659258262890683122, 1.000000000000000000, 0.9659258262890683122, 1.000000000000000000, 0.9659258262890683122, 1.000000000000000000, 0.9659258262890683122, 1.000000000000000000, 0.9659258262890683122, 1.000000000000000000, 0.9659258262890683122, 1.000000000000000000, 0.9659258262890683122, 1.000000000000000000, 0.9659258262890683122, 1.000000000000000000, 0.9659258262890683122, 1.000000000000000000, 0.9659258262890683122, 1.000000000000000000, 0.9659258262890683122, 1.000000000000000000, 0.9659258262890683122, 1.000000000000000000, 0.9659258262890683122, 1.000000000000000000, 0.9659258262890683122, 1.000000000000000000, 0.9659258262890683122, 1.000000000000000000, 0.9659258262890683122, 1.000000000000000000, 0.9659258262890683122, 1.000000000000000000, 0.9659258262890683122, 1.000000000000000000, 0.9659258262890683122, 1.000000000000000000, 0.9659258262890683122, 1.000000000000000000, 0.9659258262890683122, 1.000000000000000000, 0.9659258262890683122, 1.000000000000000000, 0.9659258262890683122, 1.000000000000000000, 0.9659258262890683122, 1.000000000000000000, 0.9659258262890683122, 1.000000000000000000, 0.9659258262890683122, 1.000000000000000000, 0.9659258262890683122, 1.000000000000000000, 0.9659258262890683122, 1.000000000000000000, 0.9659258262890683122, 1.000000000000000000, 0.9659258262890683122, 1.000000000000000000, 0.9659258262890683122, 1.000000000000000000, 0.9659258262890683122, 1.000000000000000000, 0.9659258262890683122, 1.000000000000000000, 0.9659258262890683122, 1.000000000000000000) ) ) 
 REPRESENTATION_ITEM ( '' )  SURFACE ( )  );
#6404=CARTESIAN_POINT ( 'NONE',  ( 15.04653450569339945, 67.42409749907601224, 25.98046417659831775 ) ) ;
#6414=CARTESIAN_POINT ( 'NONE',  ( 19.09188309203661049, 40.35937499999999289, -19.09188309203694445 ) ) ;
#6420=CARTESIAN_POINT ( 'NONE',  ( 25.98046417659858420, 15.01340250092397888, 15.04653450569292872 ) ) ;
#6422=CARTESIAN_POINT ( 'NONE',  ( 20.50609665441005092, 54.96875000000000000, 20.50609665440969209 ) ) ;
#6433=CARTESIAN_POINT ( 'NONE',  ( -0.04044903254992426173, 22.46131916759064850, 27.95245687107223276 ) ) ;
#6439=CARTESIAN_POINT ( 'NONE',  ( -15.01150461594595775, 48.80989583333332860, 26.00068869287368756 ) ) ;
#6443=CARTESIAN_POINT ( 'NONE',  ( 15.01150461594596308, 29.90364583333332504, -26.00068869287367335 ) ) ;
#6448=CARTESIAN_POINT ( 'NONE',  ( 25.98046417659831775, 42.50222249907603356, -15.04653450569338879 ) ) ;
#6450=CARTESIAN_POINT ( 'NONE',  ( -2.584737979205442066E-13, 57.11718750000000711, -30.02300923189239867 ) ) ;
#6454=CARTESIAN_POINT ( 'NONE',  ( 7.025853678916867295, 67.56732666574268364, 26.06988505166722803 ) ) ;
#6460=CARTESIAN_POINT ( 'NONE',  ( -24.20753774853730889, 35.34635416666666430, 13.97622843553634020 ) ) ;
#6466=CARTESIAN_POINT ( 'NONE',  ( -25.98046417659831420, 23.59597249907602290, 15.04653450569339945 ) ) ;
#6469=CARTESIAN_POINT ( 'NONE',  ( 6.950374756619257965, 38.63503499907601224, -26.09010956794244507 ) ) ;
#6474=CARTESIAN_POINT ( 'NONE',  ( -2.428612866367529427E-13, 50.24218750000000711, -27.95245687107222921 ) ) ;
#6479=CARTESIAN_POINT ( 'NONE',  ( 30.02300923189239512, 20.16406249999999645, -2.619432448724977703E-13 ) ) ;
#6480=CARTESIAN_POINT ( 'NONE',  ( 20.53372385742072481, 24.60975666759063785, -20.47846945139902175 ) ) ;
#6488=CARTESIAN_POINT ( 'NONE',  ( -20.47846945139902175, 54.68788166759063785, -20.53372385742072481 ) ) ;
#6491=CARTESIAN_POINT ( 'NONE',  ( -28.01184896238290278, 32.05208333333332860, 7.505752307973363457 ) ) ;
#6495=CARTESIAN_POINT ( 'NONE',  ( -24.18731323226221974, 47.65847249907603356, 14.01125832528330406 ) ) ;
#6501=CARTESIAN_POINT ( 'NONE',  ( 19.06425588902592239, 35.78163166759063074, 19.11951029504763611 ) ) ;
#6509=CARTESIAN_POINT ( 'NONE',  ( 25.98046417659831775, 52.81472249907603356, -15.04653450569338879 ) ) ;
#6514=CARTESIAN_POINT ( 'NONE',  ( -13.97622843553632421, 29.33072916666665719, -24.20753774853731599 ) ) ;
#6517=CARTESIAN_POINT ( 'NONE',  ( 15.01150461594643204, 31.04947916666666075, 26.00068869287340334 ) ) ;
#6520=CARTESIAN_POINT ( 'NONE',  ( 26.02091320914851025, 45.37798583425732346, -14.97647472619946463 ) ) ;
#6522=CARTESIAN_POINT ( 'NONE',  ( 20.50609665440969565, 64.42187499999998579, -20.50609665441004736 ) ) ;
#6541=CARTESIAN_POINT ( 'NONE',  ( -26.06988505166735237, 13.15142333425730925, -7.025853678916388567 ) ) ;
#6542=CARTESIAN_POINT ( 'NONE',  ( -19.09188309203694445, 67.00000000000000000, -19.09188309203661049 ) ) ;
#6546=CARTESIAN_POINT ( 'NONE',  ( 26.07999730980477437, 50.95833333333332860, -6.988114217768290004 ) ) ;
#6547=CARTESIAN_POINT ( 'NONE',  ( -28.02196122052045268, 36.92746500092395934, 7.468012846824790607 ) ) ;
#6548=CARTESIAN_POINT ( 'NONE',  ( 14.97647472619900455, 31.90326416574268364, -26.02091320914876960 ) ) ;
#6551=CARTESIAN_POINT ( 'NONE',  ( -26.09010956794245217, 51.52565999907602645, -6.950374756619243755 ) ) ;
#6558=CARTESIAN_POINT ( 'NONE',  ( 20.50609665441005092, 34.34374999999999289, 20.50609665440969209 ) ) ;
#6563=CARTESIAN_POINT ( 'NONE',  ( 7.505752307972854531, 60.69791666666667140, -28.01184896238303423 ) ) ;
#6571=CARTESIAN_POINT ( 'NONE',  ( 14.01125832528330051, 19.29909749907602290, 24.18731323226221974 ) ) ;
#6579=CARTESIAN_POINT ( 'NONE',  ( 6.988114217767829928, 43.51041666666666430, -26.07999730980489872 ) ) ;
#6584=CARTESIAN_POINT ( 'NONE',  ( 26.02091320914851025, 11.00298583425731103, -14.97647472619946463 ) ) ;
#6585=CARTESIAN_POINT ( 'NONE',  ( -20.50609665440969209, 55.82812499999999289, 20.50609665441005092 ) ) ;
#6595=CARTESIAN_POINT ( 'NONE',  ( 6.950374756619721595, 36.06809000092397355, 26.09010956794232428 ) ) ;
#6601=CARTESIAN_POINT ( 'NONE',  ( 26.00068869287340334, 61.12760416666665719, -15.01150461594642316 ) ) ;
#6605=CARTESIAN_POINT ( 'NONE',  ( -2.584737979205441561E-13, 26.17968750000000000, -30.02300923189239512 ) ) ;
#6610=CARTESIAN_POINT ( 'NONE',  ( 30.02300923189239867, 46.22618083240936215, -0.04044903255044467877 ) ) ;
#6612=CARTESIAN_POINT ( 'NONE',  ( 20.50609665441005092, 61.84374999999998579, 20.50609665440969209 ) ) ;
#6616=CARTESIAN_POINT ( 'NONE',  ( 19.09188309203661049, 12.85937500000000000, -19.09188309203694445 ) ) ;
#6622=CARTESIAN_POINT ( 'NONE',  ( -13.97622843553588901, 28.18489583333333215, 24.20753774853756823 ) ) ;
#6627=CARTESIAN_POINT ( 'NONE',  ( -20.53372385742107653, 20.87461833240935505, -20.47846945139867003 ) ) ;
#6629=CARTESIAN_POINT ( 'NONE',  ( 24.22776226481265383, 36.20013916574269075, 13.94119854578893580 ) ) ;
#6633=CARTESIAN_POINT ( 'NONE',  ( -26.07999730980477437, 59.55208333333332149, 6.988114217768305103 ) ) ;
#6638=CARTESIAN_POINT ( 'NONE',  ( -20.50609665440969209, 21.45312499999999645, 20.50609665441005092 ) ) ;
#6639=CARTESIAN_POINT ( 'NONE',  ( 26.02091320914851025, 28.19048583425731636, -14.97647472619946463 ) ) ;
#6649=CARTESIAN_POINT ( 'NONE',  ( 30.02300923189239867, 52.53944416759064495, 0.04044903254992252006 ) ) ;
#6652=CARTESIAN_POINT ( 'NONE',  ( 7.505752307972854531, 33.19791666666665719, -28.01184896238303423 ) ) ;
#6657=CARTESIAN_POINT ( 'NONE',  ( 6.950374756619257965, 42.07253499907601935, -26.09010956794244507 ) ) ;
#6664=CARTESIAN_POINT ( 'NONE',  ( -24.22776226481240514, 47.09673583425730214, 13.94119854578937812 ) ) ;
#6671=CARTESIAN_POINT ( 'NONE',  ( 14.97647472619900455, 62.84076416574269786, -26.02091320914876960 ) ) ;
#6675=CARTESIAN_POINT ( 'NONE',  ( -2.428612866367529427E-13, 36.49218750000000000, -27.95245687107222921 ) ) ;
#6678=CARTESIAN_POINT ( 'NONE',  ( -7.505752307973343918, 39.78645833333332860, -28.01184896238290989 ) ) ;
#6681=CARTESIAN_POINT ( 'NONE',  ( 14.97647472619947351, 46.23736083425730925, 26.02091320914850314 ) ) ;
#6683=CARTESIAN_POINT ( 'NONE',  ( 26.00068869287367335, 65.13802083333334281, 15.01150461594596308 ) ) ;
#6703=CARTESIAN_POINT ( 'NONE',  ( 14.01125832528286352, 21.02902750092397710, -24.18731323226246843 ) ) ;
#6709=CARTESIAN_POINT ( 'NONE',  ( 13.97622843553633842, 55.11197916666665719, 24.20753774853730889 ) ) ;
#6710=CARTESIAN_POINT ( 'NONE',  ( 20.47846945139902530, 42.65663166759063785, 20.53372385742071771 ) ) ;
#6712=CARTESIAN_POINT ( 'NONE',  ( -7.468012846824272799, 33.47878499907601935, 28.02196122052058413 ) ) ;
#6715=CARTESIAN_POINT ( 'NONE',  ( -19.06425588902558133, 54.39024333240934794, 19.11951029504797006 ) ) ;
#6721=ORIENTED_EDGE ( 'NONE', *, *, #1024, .T. ) ;
#6722=CARTESIAN_POINT ( 'NONE',  ( 15.01150461594596308, 33.34114583333332860, -26.00068869287367335 ) ) ;
#6726=CARTESIAN_POINT ( 'NONE',  ( 26.00068869287367335, 61.70052083333331439, 15.01150461594596308 ) ) ;
#6736=CARTESIAN_POINT ( 'NONE',  ( 24.22776226481265383, 22.45013916574269075, 13.94119854578893580 ) ) ;
#6745=CARTESIAN_POINT ( 'NONE',  ( 27.95245687107222921, 44.22656249999997868, -2.463307335887066074E-13 ) ) ;
#6750=CARTESIAN_POINT ( 'NONE',  ( -0.04044903254990864921, 12.14881916759064140, 30.02300923189239867 ) ) ;
#6751=CARTESIAN_POINT ( 'NONE',  ( -15.01150461594595775, 52.24739583333332860, 26.00068869287368756 ) ) ;
#6763=CARTESIAN_POINT ( 'NONE',  ( -26.06988505166735237, 33.77642333425730214, -7.025853678916388567 ) ) ;
#6767=CARTESIAN_POINT ( 'NONE',  ( 15.01150461594596308, 60.84114583333332860, -26.00068869287367335 ) ) ;
#6771=CARTESIAN_POINT ( 'NONE',  ( -28.01184896238304134, 32.33854166666666430, -7.505752307972844761 ) ) ;
#6776=CARTESIAN_POINT ( 'NONE',  ( -20.53372385742107653, 44.93711833240935505, -20.47846945139867003 ) ) ;
#6779=CARTESIAN_POINT ( 'NONE',  ( -20.50609665440969209, 59.26562500000000000, 20.50609665441005092 ) ) ;
#6784=CARTESIAN_POINT ( 'NONE',  ( -24.20753774853756823, 15.29427083333332504, -13.97622843553588723 ) ) ;
#6794=CARTESIAN_POINT ( 'NONE',  ( 28.02196122052058413, 22.30690999907601579, 7.468012846824272799 ) ) ;
#6796=CARTESIAN_POINT ( 'NONE',  ( -24.22776226481266448, 37.91888916574269075, -13.94119854578892514 ) ) ;
#6800=CARTESIAN_POINT ( 'NONE',  ( -2.428612866367529427E-13, 63.99218749999997868, -27.95245687107222921 ) ) ;
#6805=CARTESIAN_POINT ( 'NONE',  ( 15.01150461594643204, 37.92447916666666430, 26.00068869287340334 ) ) ;
#6806=CARTESIAN_POINT ( 'NONE',  ( -28.00173670424549499, 30.33892333425730925, -7.543491769121417612 ) ) ;
#6815=CARTESIAN_POINT ( 'NONE',  ( 26.02091320914851025, 52.25298583425730925, -14.97647472619946463 ) ) ;
#6818=CARTESIAN_POINT ( 'NONE',  ( -28.01184896238304134, 32.33854166666666430, -7.505752307972844761 ) ) ;
#6822=CARTESIAN_POINT ( 'NONE',  ( -26.06988505166722803, 44.36420166574269075, 7.025853678916877953 ) ) ;
#6829=CARTESIAN_POINT ( 'NONE',  ( -19.11951029504763611, 46.95350666759064495, 19.06425588902592239 ) ) ;
#6838=CARTESIAN_POINT ( 'NONE',  ( -14.01125832528328985, 14.14284749907602290, -24.18731323226223040 ) ) ;
#6843=CARTESIAN_POINT ( 'NONE',  ( -26.07999730980477437, 32.05208333333332860, 6.988114217768305103 ) ) ;
#6847=CARTESIAN_POINT ( 'NONE',  ( -28.01184896238304134, 42.65104166666666430, -7.505752307972844761 ) ) ;
#6851=CARTESIAN_POINT ( 'NONE',  ( -7.543491769121417612, 60.41704833425730214, 28.00173670424549499 ) ) ;
#6852=CARTESIAN_POINT ( 'NONE',  ( -19.11951029504763611, 57.26600666759063785, 19.06425588902592239 ) ) ;
#6854=CARTESIAN_POINT ( 'NONE',  ( 26.00068869287367335, 61.70052083333331439, 15.01150461594596308 ) ) ;
#6872=CARTESIAN_POINT ( 'NONE',  ( 13.94119854578937812, 22.17486083425730925, 24.22776226481240514 ) ) ;
#6877=CARTESIAN_POINT ( 'NONE',  ( -25.98046417659859486, 47.66965250092398065, -15.04653450569291628 ) ) ;
#6878=CARTESIAN_POINT ( 'NONE',  ( -28.00173670424535644, 37.48920166574269075, 7.543491769121936308 ) ) ;
#6882=CARTESIAN_POINT ( 'NONE',  ( 0.04044903255044120238, 64.27305583240934084, 27.95245687107223276 ) ) ;
#6885=CARTESIAN_POINT ( 'NONE',  ( -28.01184896238304134, 15.15104166666666252, -7.505752307972844761 ) ) ;
#6892=CARTESIAN_POINT ( 'NONE',  ( 15.01150461594596308, 36.77864583333332860, -26.00068869287367335 ) ) ;
#6907=CARTESIAN_POINT ( 'NONE',  ( 14.01125832528330051, 29.61159749907602290, 24.18731323226221974 ) ) ;
#6914=CARTESIAN_POINT ( 'NONE',  ( 19.09188309203694800, 51.53124999999999289, 19.09188309203660694 ) ) ;
#6919=CARTESIAN_POINT ( 'NONE',  ( 25.98046417659858420, 21.88840250092397710, 15.04653450569292872 ) ) ;
#6920=CARTESIAN_POINT ( 'NONE',  ( -7.505752307973343918, 63.84895833333332860, -28.01184896238290989 ) ) ;
#6932=CARTESIAN_POINT ( 'NONE',  ( -24.22776226481240514, 36.78423583425730214, 13.94119854578937812 ) ) ;
#6938=CARTESIAN_POINT ( 'NONE',  ( 26.00068869287367335, 58.26302083333332149, 15.01150461594596308 ) ) ;
#6941=CARTESIAN_POINT ( 'NONE',  ( 2.740863092043355209E-13, 41.64843750000000000, 30.02300923189239512 ) ) ;
#6946=CARTESIAN_POINT ( 'NONE',  ( -28.02196122052058413, 54.96315999907602645, -7.468012846824272799 ) ) ;
#6948=CARTESIAN_POINT ( 'NONE',  ( 2.740863092043355209E-13, 58.83593750000000711, 30.02300923189239867 ) ) ;
#6952=CARTESIAN_POINT ( 'NONE',  ( 2.584737979205441561E-13, 21.02343749999999645, 27.95245687107222921 ) ) ;
#6963=CARTESIAN_POINT ( 'NONE',  ( -7.543491769121917656, 28.03607666574268364, -28.00173670424536354 ) ) ;
#6966=CARTESIAN_POINT ( 'NONE',  ( 14.01125832528330051, 33.04909749907601935, 24.18731323226221974 ) ) ;
#6970=CARTESIAN_POINT ( 'NONE',  ( -27.95245687107222921, 66.57031250000000000, 2.498001805406602216E-13 ) ) ;
#6975=EDGE_CURVE ( 'NONE', #16033, #32341, #14157, .T. ) ;
#6977=CARTESIAN_POINT ( 'NONE',  ( -20.50609665441004736, 29.18749999999999645, -20.50609665440969565 ) ) ;
#6978=CARTESIAN_POINT ( 'NONE',  ( -30.02300923189239867, 33.63319416759063785, -0.04044903254991731589 ) ) ;
#6987=CARTESIAN_POINT ( 'NONE',  ( -15.04653450569291984, 63.99777750092396644, 25.98046417659859486 ) ) ;
#6990=CARTESIAN_POINT ( 'NONE',  ( -30.02300923189239867, 28.75781249999999645, 2.654126918244514854E-13 ) ) ;
#6995=CARTESIAN_POINT ( 'NONE',  ( 14.01125832528330051, 39.92409749907602645, 24.18731323226221974 ) ) ;
#7002=CARTESIAN_POINT ( 'NONE',  ( 14.01125832528286352, 45.09152750092398065, -24.18731323226246843 ) ) ;
#7008=CARTESIAN_POINT ( 'NONE',  ( 15.04653450569339945, 63.98659749907601935, 25.98046417659831775 ) ) ;
#7012=CARTESIAN_POINT ( 'NONE',  ( -19.09188309203660694, 38.64062500000000000, 19.09188309203694800 ) ) ;
#7015=CARTESIAN_POINT ( 'NONE',  ( 7.505752307973351023, 38.06770833333332860, 28.01184896238290278 ) ) ;
#7019=CARTESIAN_POINT ( 'NONE',  ( 30.02300923189239867, 55.97694416759064495, 0.04044903254992252006 ) ) ;
#7020=CARTESIAN_POINT ( 'NONE',  ( -7.025853678916393008, 60.41704833425730214, 26.06988505166735592 ) ) ;
#7022=CARTESIAN_POINT ( 'NONE',  ( 7.468012846824281681, 18.01003499907601935, -28.02196122052058058 ) ) ;
#7042=CARTESIAN_POINT ( 'NONE',  ( -13.94119854578936923, 17.01861083425731280, -24.22776226481241224 ) ) ;
#7047=CARTESIAN_POINT ( 'NONE',  ( 28.00173670424549499, 45.80767333425730925, 7.543491769121417612 ) ) ;
#7049=CARTESIAN_POINT ( 'NONE',  ( -26.02091320914878025, 37.91888916574269075, -14.97647472619899389 ) ) ;
#7052=CARTESIAN_POINT ( 'NONE',  ( 7.025853678916867295, 64.12982666574268364, 26.06988505166722803 ) ) ;
#7063=CARTESIAN_POINT ( 'NONE',  ( 26.00068869287340334, 47.37760416666666430, -15.01150461594642316 ) ) ;
#7076=CARTESIAN_POINT ( 'NONE',  ( 6.950374756619257965, 28.32253499907601579, -26.09010956794244507 ) ) ;
#7084=CARTESIAN_POINT ( 'NONE',  ( 24.20753774853731244, 54.25260416666666430, -13.97622843553632599 ) ) ;
#7089=CARTESIAN_POINT ( 'NONE',  ( 7.468012846824777284, 18.88059000092397355, 28.02196122052045268 ) ) ;
#7090=CARTESIAN_POINT ( 'NONE',  ( -20.50609665441004736, 67.00000000000000000, -20.50609665440969565 ) ) ;
#7102=CARTESIAN_POINT ( 'NONE',  ( 19.06425588902592239, 35.78163166759063074, 19.11951029504763611 ) ) ;
#7109=CARTESIAN_POINT ( 'NONE',  ( -26.00068869287340334, 42.22135416666666430, 15.01150461594643382 ) ) ;
#7114=CARTESIAN_POINT ( 'NONE',  ( 25.98046417659831775, 52.81472249907603356, -15.04653450569338879 ) ) ;
#7116=CARTESIAN_POINT ( 'NONE',  ( -7.505752307973343918, 60.41145833333332149, -28.01184896238290989 ) ) ;
#7121=CARTESIAN_POINT ( 'NONE',  ( 19.09188309203694800, 20.59374999999999645, 19.09188309203660694 ) ) ;
#7135=CARTESIAN_POINT ( 'NONE',  ( -26.09010956794245217, 41.21315999907602645, -6.950374756619243755 ) ) ;
#7139=CARTESIAN_POINT ( 'NONE',  ( -19.09188309203694445, 67.00000000000000000, -19.09188309203661049 ) ) ;
#7144=CARTESIAN_POINT ( 'NONE',  ( 7.505752307972854531, 29.76041666666666430, -28.01184896238303423 ) ) ;
#7145=CARTESIAN_POINT ( 'NONE',  ( 30.02300923189239867, 31.91444416759064495, 0.04044903254992252006 ) ) ;
#7155=CARTESIAN_POINT ( 'NONE',  ( 28.02196122052045268, 62.70871500092398065, -7.468012846824774620 ) ) ;
#7158=CARTESIAN_POINT ( 'NONE',  ( 28.01184896238304134, 27.18229166666666430, 7.505752307972846538 ) ) ;
#7164=CARTESIAN_POINT ( 'NONE',  ( 27.95245687107223276, 53.10118083240936215, -0.04044903255042905932 ) ) ;
#7171=CARTESIAN_POINT ( 'NONE',  ( -6.950374756619716266, 44.66184000092397355, -26.09010956794232428 ) ) ;
#7178=CARTESIAN_POINT ( 'NONE',  ( -14.97647472619899389, 64.55951416574268364, 26.02091320914878025 ) ) ;
#7183=CARTESIAN_POINT ( 'NONE',  ( -13.97622843553632421, 32.76822916666666430, -24.20753774853731599 ) ) ;
#7186=CARTESIAN_POINT ( 'NONE',  ( 2.740863092043355209E-13, 41.64843750000000000, 30.02300923189239512 ) ) ;
#7189=CARTESIAN_POINT ( 'NONE',  ( 20.53372385742072481, 55.54725666759064495, -20.47846945139902175 ) ) ;
#7190=CARTESIAN_POINT ( 'NONE',  ( 26.06988505166735592, 62.99517333425730214, 7.025853678916393896 ) ) ;
#7192=CARTESIAN_POINT ( 'NONE',  ( -7.468012846824272799, 19.72878499907601935, 28.02196122052058413 ) ) ;
#7213=CARTESIAN_POINT ( 'NONE',  ( 27.95245687107223986, 18.16444416759064140, 0.04044903254993640479 ) ) ;
#7218=CARTESIAN_POINT ( 'NONE',  ( -7.468012846824771955, 48.09934000092398065, -28.02196122052045624 ) ) ;
#7219=CARTESIAN_POINT ( 'NONE',  ( 0.04044903255045854962, 40.21055583240935505, 30.02300923189239867 ) ) ;
#7222=CARTESIAN_POINT ( 'NONE',  ( -0.04044903255042732459, 62.55430583240935505, -27.95245687107223986 ) ) ;
#7225=CARTESIAN_POINT ( 'NONE',  ( 7.505752307972854531, 16.01041666666666075, -28.01184896238303423 ) ) ;
#7231=CARTESIAN_POINT ( 'NONE',  ( 28.01184896238304134, 47.80729166666666430, 7.505752307972846538 ) ) ;
#7244=CARTESIAN_POINT ( 'NONE',  ( -27.95245687107223986, 23.88243083240935505, 0.04044903255043252877 ) ) ;
#7252=CARTESIAN_POINT ( 'NONE',  ( 6.988114217768294445, 48.38020833333332860, 26.07999730980477437 ) ) ;
#7256=CARTESIAN_POINT ( 'NONE',  ( 6.988114217768294445, 27.75520833333332860, 26.07999730980477437 ) ) ;
#7257=CARTESIAN_POINT ( 'NONE',  ( -28.02196122052045268, 16.30246500092397355, 7.468012846824790607 ) ) ;
#7259=CARTESIAN_POINT ( 'NONE',  ( 20.50609665440969565, 64.42187499999998579, -20.50609665441004736 ) ) ;
#7268=CARTESIAN_POINT ( 'NONE',  ( 6.988114217768294445, 65.56770833333332860, 26.07999730980477437 ) ) ;
#7273=CARTESIAN_POINT ( 'NONE',  ( -6.950374756619716266, 44.66184000092397355, -26.09010956794232428 ) ) ;
#7277=CARTESIAN_POINT ( 'NONE',  ( 28.01184896238290278, 13.14583333333332860, -7.505752307973347470 ) ) ;
#7281=CARTESIAN_POINT ( 'NONE',  ( 15.01150461594596308, 43.65364583333332860, -26.00068869287367335 ) ) ;
#7286=CARTESIAN_POINT ( 'NONE',  ( 20.53372385742108008, 50.09336833240935505, 20.47846945139866648 ) ) ;
#7293=CARTESIAN_POINT ( 'NONE',  ( -13.97622843553588901, 21.30989583333331794, 24.20753774853756823 ) ) ;
#7306=CARTESIAN_POINT ( 'NONE',  ( 13.94119854578893580, 45.65326416574269786, -24.22776226481265383 ) ) ;
#7310=CARTESIAN_POINT ( 'NONE',  ( -24.20753774853756823, 63.41927083333333570, -13.97622843553588723 ) ) ;
#7315=CARTESIAN_POINT ( 'NONE',  ( -2.584737979205441561E-13, 36.49218750000000000, -30.02300923189239512 ) ) ;
#7316=CARTESIAN_POINT ( 'NONE',  ( 20.53372385742072481, 34.92225666759063074, -20.47846945139902175 ) ) ;
#7328=CARTESIAN_POINT ( 'NONE',  ( -2.584737979205441561E-13, 15.86718749999999645, -30.02300923189239512 ) ) ;
#7331=CARTESIAN_POINT ( 'NONE',  ( -30.02300923189239867, 42.50781249999998579, 2.654126918244514854E-13 ) ) ;
#7336=CARTESIAN_POINT ( 'NONE',  ( -24.18731323226221974, 54.53347249907601935, 14.01125832528330406 ) ) ;
#7350=CARTESIAN_POINT ( 'NONE',  ( -28.02196122052058413, 68.71315999907601224, -7.468012846824272799 ) ) ;
#7354=CARTESIAN_POINT ( 'NONE',  ( 24.20753774853756113, 34.20052083333332860, 13.97622843553589789 ) ) ;
#7357=CARTESIAN_POINT ( 'NONE',  ( -30.02300923189239512, 42.50781249999997868, 2.654126918244515359E-13 ) ) ;
#7361=CARTESIAN_POINT ( 'NONE',  ( 15.04653450569292872, 62.27902750092396644, -25.98046417659857710 ) ) ;
#7362=CARTESIAN_POINT ( 'NONE',  ( 13.94119854578937812, 63.42486083425730925, 24.22776226481240514 ) ) ;
#7367=CARTESIAN_POINT ( 'NONE',  ( -15.04653450569338524, 14.14284749907602290, -25.98046417659831775 ) ) ;
#7388=CARTESIAN_POINT ( 'NONE',  ( -6.950374756619716266, 20.59934000092397355, -26.09010956794232428 ) ) ;
#7392=CARTESIAN_POINT ( 'NONE',  ( 14.97647472619947351, 49.67486083425730925, 26.02091320914850314 ) ) ;
#7394=CARTESIAN_POINT ( 'NONE',  ( 15.04653450569339945, 33.04909749907601935, 25.98046417659831775 ) ) ;
#7399=CARTESIAN_POINT ( 'NONE',  ( 24.22776226481265383, 67.13763916574266943, 13.94119854578893580 ) ) ;
#7408=CARTESIAN_POINT ( 'NONE',  ( -20.50609665441004736, 42.93750000000000000, -20.50609665440969565 ) ) ;
#7423=CARTESIAN_POINT ( 'NONE',  ( -24.18731323226221974, 23.59597249907602290, 14.01125832528330406 ) ) ;
#7431=CARTESIAN_POINT ( 'NONE',  ( 24.20753774853731244, 47.37760416666666430, -13.97622843553632599 ) ) ;
#7437=CARTESIAN_POINT ( 'NONE',  ( 19.09188309203694800, 27.46875000000000000, 19.09188309203660694 ) ) ;
#7440=CARTESIAN_POINT ( 'NONE',  ( -14.97647472619946285, 17.01861083425731280, -26.02091320914851025 ) ) ;
#7441=CARTESIAN_POINT ( 'NONE',  ( 26.00068869287340334, 61.12760416666665719, -15.01150461594642316 ) ) ;
#7451=CARTESIAN_POINT ( 'NONE',  ( -26.09010956794232428, 40.36496500092396644, 6.950374756619732253 ) ) ;
#7456=CARTESIAN_POINT ( 'NONE',  ( 28.01184896238290278, 20.02083333333332860, -7.505752307973347470 ) ) ;
#7461=CARTESIAN_POINT ( 'NONE',  ( -26.00068869287368756, 39.35677083333331439, -15.01150461594595775 ) ) ;
#7467=CARTESIAN_POINT ( 'NONE',  ( -7.543491769121917656, 55.53607666574269075, -28.00173670424536354 ) ) ;
#7475=CARTESIAN_POINT ( 'NONE',  ( -13.97622843553632421, 22.45572916666666430, -24.20753774853731599 ) ) ;
#7492=CARTESIAN_POINT ( 'NONE',  ( 19.11951029504763611, 17.73475666759064140, -19.06425588902591173 ) ) ;
#7496=CARTESIAN_POINT ( 'NONE',  ( -26.00068869287368756, 32.48177083333332860, -15.01150461594595775 ) ) ;
#7506=CARTESIAN_POINT ( 'NONE',  ( 30.02300923189239512, 13.28906249999999289, -2.619432448724977703E-13 ) ) ;
#7509=CARTESIAN_POINT ( 'NONE',  ( -28.01184896238290278, 35.48958333333332860, 7.505752307973363457 ) ) ;
#7514=CARTESIAN_POINT ( 'NONE',  ( -13.94119854578892514, 54.24701416574269075, 24.22776226481266448 ) ) ;
#7520=CARTESIAN_POINT ( 'NONE',  ( -26.07999730980490583, 15.15104166666666252, -6.988114217767815717 ) ) ;
#7528=CARTESIAN_POINT ( 'NONE',  ( -24.22776226481266448, 20.73138916574268720, -13.94119854578892514 ) ) ;
#7532=CARTESIAN_POINT ( 'NONE',  ( 27.95245687107222921, 47.66406249999998579, -2.463307335887066074E-13 ) ) ;
#7535=CARTESIAN_POINT ( 'NONE',  ( -28.01184896238304134, 46.08854166666666430, -7.505752307972844761 ) ) ;
#7537=CARTESIAN_POINT ( 'NONE',  ( 20.47846945139902530, 56.40663166759065206, 20.53372385742071771 ) ) ;
#7538=CARTESIAN_POINT ( 'NONE',  ( 24.18731323226247554, 56.26340250092398065, 14.01125832528285997 ) ) ;
#7540=CARTESIAN_POINT ( 'NONE',  ( -28.00173670424535644, 16.86420166574268720, 7.543491769121936308 ) ) ;
#7545=CARTESIAN_POINT ( 'NONE',  ( -26.00068869287340334, 66.28385416666662877, 15.01150461594643382 ) ) ;
#7559=CARTESIAN_POINT ( 'NONE',  ( -14.01125832528285109, 33.06027750092398776, 24.18731323226248264 ) ) ;
#7567=CARTESIAN_POINT ( 'NONE',  ( 20.53372385742108008, 46.65586833240934794, 20.47846945139866648 ) ) ;
#7571=CARTESIAN_POINT ( 'NONE',  ( -13.94119854578892514, 64.55951416574268364, 24.22776226481266448 ) ) ;
#7575=CARTESIAN_POINT ( 'NONE',  ( -20.50609665441004736, 22.31250000000000000, -20.50609665440969565 ) ) ;
#7583=CARTESIAN_POINT ( 'NONE',  ( -30.02300923189239512, 45.94531249999997868, 2.654126918244515359E-13 ) ) ;
#7584=CARTESIAN_POINT ( 'NONE',  ( 2.740863092043355209E-13, 58.83593750000000000, 30.02300923189239512 ) ) ;
#7597=CARTESIAN_POINT ( 'NONE',  ( -13.94119854578892514, 30.18451416574268720, 24.22776226481266448 ) ) ;
#7604=CARTESIAN_POINT ( 'NONE',  ( -6.988114217767819270, 48.66666666666666430, 26.07999730980490583 ) ) ;
#7608=CARTESIAN_POINT ( 'NONE',  ( 27.95245687107223276, 33.91406249999998579, -2.463307335887066074E-13 ) ) ;
#7609=CARTESIAN_POINT ( 'NONE',  ( 26.02091320914851025, 24.75298583425730925, -14.97647472619946463 ) ) ;
#7610=CARTESIAN_POINT ( 'NONE',  ( -26.00068869287340334, 66.28385416666662877, 15.01150461594643382 ) ) ;
#7620=CARTESIAN_POINT ( 'NONE',  ( -19.06425588902591173, 44.37538166759063785, -19.11951029504763611 ) ) ;
#7624=CARTESIAN_POINT ( 'NONE',  ( -2.584737979205441561E-13, 15.86718749999999645, -30.02300923189239512 ) ) ;
#7628=CARTESIAN_POINT ( 'NONE',  ( -20.50609665441004736, 42.93750000000000000, -20.50609665440969565 ) ) ;
#7633=CARTESIAN_POINT ( 'NONE',  ( 0.04044903255045854962, 57.39805583240935505, 30.02300923189239867 ) ) ;
#7635=CARTESIAN_POINT ( 'NONE',  ( -28.01184896238304134, 63.27604166666667140, -7.505752307972844761 ) ) ;
#7638=CARTESIAN_POINT ( 'NONE',  ( -6.988114217768288228, 63.84895833333332860, -26.07999730980477437 ) ) ;
#7641=CARTESIAN_POINT ( 'NONE',  ( 19.09188309203661049, 23.17187499999999289, -19.09188309203694445 ) ) ;
#7657=CARTESIAN_POINT ( 'NONE',  ( -7.025853678916393008, 19.16704833425730570, 26.06988505166735592 ) ) ;
#7661=CARTESIAN_POINT ( 'NONE',  ( -26.00068869287368756, 39.35677083333331439, -15.01150461594595775 ) ) ;
#7673=CARTESIAN_POINT ( 'NONE',  ( -7.543491769121417612, 63.85454833425732346, 28.00173670424549499 ) ) ;
#7675=CARTESIAN_POINT ( 'NONE',  ( -2.584737979205442066E-13, 43.36718749999999289, -30.02300923189239867 ) ) ;
#7681=CARTESIAN_POINT ( 'NONE',  ( -6.950374756619247307, 50.66628499907601935, 26.09010956794245217 ) ) ;
#7686=CARTESIAN_POINT ( 'NONE',  ( -2.428612866367529427E-13, 12.42968749999999822, -27.95245687107223276 ) ) ;
#7695=CARTESIAN_POINT ( 'NONE',  ( 19.11951029504797006, 22.59336833240935505, 19.06425588902558133 ) ) ;
#7699=CARTESIAN_POINT ( 'NONE',  ( -24.20753774853730889, 42.22135416666666430, 13.97622843553633842 ) ) ;
#7703=CARTESIAN_POINT ( 'NONE',  ( -7.505752307973343918, 46.66145833333332860, -28.01184896238290989 ) ) ;
#7705=CARTESIAN_POINT ( 'NONE',  ( 30.02300923189239512, 16.72656249999999645, -2.619432448724977703E-13 ) ) ;
#7706=CARTESIAN_POINT ( 'NONE',  ( 26.02091320914851025, 11.00298583425731103, -14.97647472619946463 ) ) ;
#7713=CARTESIAN_POINT ( 'NONE',  ( -28.01184896238304134, 66.71354166666665719, -7.505752307972844761 ) ) ;
#7727=CARTESIAN_POINT ( 'NONE',  ( 0.04044903254993986036, 27.61756916759064140, -27.95245687107223986 ) ) ;
#7733=CARTESIAN_POINT ( 'NONE',  ( -15.04653450569338524, 48.51784749907601935, -25.98046417659831775 ) ) ;
#7737=CARTESIAN_POINT ( 'NONE',  ( -26.07999730980490583, 18.58854166666666430, -6.988114217767815717 ) ) ;
#7740=CARTESIAN_POINT ( 'NONE',  ( -28.01184896238304134, 25.46354166666666430, -7.505752307972844761 ) ) ;
#7744=CARTESIAN_POINT ( 'NONE',  ( 7.468012846824777284, 42.94309000092397355, 28.02196122052045268 ) ) ;
#7746=CARTESIAN_POINT ( 'NONE',  ( -7.505752307973343918, 43.22395833333332860, -28.01184896238290989 ) ) ;
#7747=CARTESIAN_POINT ( 'NONE',  ( -20.50609665441004736, 63.56249999999999289, -20.50609665440969565 ) ) ;
#7759=CARTESIAN_POINT ( 'NONE',  ( -28.01184896238304134, 15.15104166666666252, -7.505752307972844761 ) ) ;
#7764=CARTESIAN_POINT ( 'NONE',  ( -14.01125832528328985, 31.33034749907602290, -24.18731323226223040 ) ) ;
#7771=CARTESIAN_POINT ( 'NONE',  ( -6.988114217768288228, 56.97395833333333570, -26.07999730980477437 ) ) ;
#7775=CARTESIAN_POINT ( 'NONE',  ( 13.97622843553633842, 37.92447916666666430, 24.20753774853730889 ) ) ;
#7776=CARTESIAN_POINT ( 'NONE',  ( 7.468012846824777284, 29.19309000092397000, 28.02196122052045268 ) ) ;
#7777=CARTESIAN_POINT ( 'NONE',  ( 28.02196122052058413, 22.30690999907601579, 7.468012846824272799 ) ) ;
#7786=CARTESIAN_POINT ( 'NONE',  ( 19.11951029504763611, 38.35975666759064495, -19.06425588902591173 ) ) ;
#7790=CARTESIAN_POINT ( 'NONE',  ( 7.505752307972854531, 19.44791666666666075, -28.01184896238303423 ) ) ;
#7795=CARTESIAN_POINT ( 'NONE',  ( 20.50609665441005092, 51.53124999999999289, 20.50609665440969209 ) ) ;
#7797=PLANE ( 'NONE',  #8634 ) ;
#7801=CARTESIAN_POINT ( 'NONE',  ( -25.98046417659831420, 57.97097249907601935, 15.04653450569339945 ) ) ;
#7803=CARTESIAN_POINT ( 'NONE',  ( -30.02300923189239867, 66.57031250000000000, 2.654126918244514854E-13 ) ) ;
#7806=CARTESIAN_POINT ( 'NONE',  ( 6.988114217767829928, 57.26041666666666430, -26.07999730980489872 ) ) ;
#7809=CARTESIAN_POINT ( 'NONE',  ( 2.584737979205441561E-13, 31.33593749999999289, 27.95245687107222921 ) ) ;
#7815=CARTESIAN_POINT ( 'NONE',  ( -27.95245687107223986, 50.82069416759063785, -0.04044903254993292840 ) ) ;
#7827=CARTESIAN_POINT ( 'NONE',  ( -24.18731323226248264, 16.73215250092398065, -14.01125832528284931 ) ) ;
#7831=CARTESIAN_POINT ( 'NONE',  ( -20.50609665440969209, 38.64062500000000000, 20.50609665441005092 ) ) ;
#7835=CARTESIAN_POINT ( 'NONE',  ( 7.505752307973351023, 24.31770833333332504, 28.01184896238290278 ) ) ;
#7842=CARTESIAN_POINT ( 'NONE',  ( -26.02091320914878025, 31.04388916574268364, -14.97647472619899389 ) ) ;
#7844=CARTESIAN_POINT ( 'NONE',  ( 7.505752307972854531, 40.07291666666666430, -28.01184896238303423 ) ) ;
#7850=CARTESIAN_POINT ( 'NONE',  ( 26.06988505166722803, 52.95795166574269075, -7.025853678916862854 ) ) ;
#7855=CARTESIAN_POINT ( 'NONE',  ( 13.97622843553589966, 16.15364583333333215, -24.20753774853756113 ) ) ;
#7862=CARTESIAN_POINT ( 'NONE',  ( 26.06988505166722803, 22.02045166574269075, -7.025853678916862854 ) ) ;
#7866=CARTESIAN_POINT ( 'NONE',  ( 26.07999730980490227, 44.36979166666666430, 6.988114217767821046 ) ) ;
#7869=CARTESIAN_POINT ( 'NONE',  ( 20.50609665441005092, 44.65624999999999289, 20.50609665440969209 ) ) ;
#7872=CARTESIAN_POINT ( 'NONE',  ( 28.01184896238290278, 16.58333333333333215, -7.505752307973347470 ) ) ;
#7873=CARTESIAN_POINT ( 'NONE',  ( 25.98046417659858420, 15.01340250092397888, 15.04653450569292872 ) ) ;
#7880=CARTESIAN_POINT ( 'NONE',  ( 2.740863092043355209E-13, 65.71093749999997158, 30.02300923189239512 ) ) ;
#7898=CARTESIAN_POINT ( 'NONE',  ( 19.11951029504763611, 28.04725666759063429, -19.06425588902591173 ) ) ;
#7905=CARTESIAN_POINT ( 'NONE',  ( 28.02196122052058413, 49.80690999907602645, 7.468012846824272799 ) ) ;
#7908=PRESENTATION_STYLE_ASSIGNMENT (( #24042 ) ) ;
#7909=CARTESIAN_POINT ( 'NONE',  ( -13.97622843553588901, 21.30989583333331794, 24.20753774853756823 ) ) ;
#7912=CARTESIAN_POINT ( 'NONE',  ( 2.740863092043355209E-13, 24.46093749999999645, 30.02300923189239512 ) ) ;
#7916=CARTESIAN_POINT ( 'NONE',  ( -28.02196122052045268, 36.92746500092395934, 7.468012846824790607 ) ) ;
#7918=CARTESIAN_POINT ( 'NONE',  ( 2.740863092043355209E-13, 55.39843749999999289, 30.02300923189239512 ) ) ;
#7928=CARTESIAN_POINT ( 'NONE',  ( -20.50609665440969209, 24.89062500000000000, 20.50609665441005092 ) ) ;
#7933=CARTESIAN_POINT ( 'NONE',  ( -26.06988505166722803, 30.61420166574267654, 7.025853678916877953 ) ) ;
#7941=CARTESIAN_POINT ( 'NONE',  ( -26.07999730980477437, 62.98958333333332149, 6.988114217768305103 ) ) ;
#7945=CARTESIAN_POINT ( 'NONE',  ( -13.97622843553632777, 39.64322916666667140, -24.20753774853731599 ) ) ;
#7946=CARTESIAN_POINT ( 'NONE',  ( -28.02196122052045268, 26.61496500092397355, 7.468012846824790607 ) ) ;
#7947=CARTESIAN_POINT ( 'NONE',  ( -26.02091320914878025, 20.73138916574268720, -14.97647472619899389 ) ) ;
#7952=CARTESIAN_POINT ( 'NONE',  ( 24.22776226481265383, 46.51263916574269786, 13.94119854578893580 ) ) ;
#7958=CARTESIAN_POINT ( 'NONE',  ( 27.95245687107223986, 42.22694416759065206, 0.04044903254993640479 ) ) ;
#7962=CARTESIAN_POINT ( 'NONE',  ( -20.50609665440969209, 18.01562499999999645, 20.50609665441005092 ) ) ;
#7967=CARTESIAN_POINT ( 'NONE',  ( 26.00068869287367335, 51.38802083333332149, 15.01150461594596308 ) ) ;
#7971=CARTESIAN_POINT ( 'NONE',  ( -0.04044903255044120238, 59.11680583240937636, -30.02300923189239867 ) ) ;
#7976=CARTESIAN_POINT ( 'NONE',  ( -24.20753774853756823, 59.98177083333332860, -13.97622843553588723 ) ) ;
#7979=CARTESIAN_POINT ( 'NONE',  ( -2.428612866367529427E-13, 36.49218750000000000, -27.95245687107222921 ) ) ;
#7985=CARTESIAN_POINT ( 'NONE',  ( 7.025853678916403666, 58.69829833425730925, -26.06988505166735237 ) ) ;
#8000=CARTESIAN_POINT ( 'NONE',  ( -6.950374756619716266, 17.16184000092397000, -26.09010956794232428 ) ) ;
#8005=CARTESIAN_POINT ( 'NONE',  ( -15.01150461594642138, 43.08072916666666430, -26.00068869287340334 ) ) ;
#8009=CARTESIAN_POINT ( 'NONE',  ( -15.01150461594595775, 21.30989583333331794, 26.00068869287368756 ) ) ;
#8015=CARTESIAN_POINT ( 'NONE',  ( -7.543491769121917656, 34.91107666574267654, -28.00173670424536354 ) ) ;
#8017=CARTESIAN_POINT ( 'NONE',  ( -28.01184896238290278, 42.36458333333332860, 7.505752307973363457 ) ) ;
#8022=CARTESIAN_POINT ( 'NONE',  ( 0.04044903255044120238, 64.27305583240934084, 27.95245687107223276 ) ) ;
#8034=CARTESIAN_POINT ( 'NONE',  ( -13.94119854578892514, 16.43451416574268720, 24.22776226481266448 ) ) ;
#8039=CARTESIAN_POINT ( 'NONE',  ( 19.09188309203661049, 47.23437499999999289, -19.09188309203694445 ) ) ;
#8043=CARTESIAN_POINT ( 'NONE',  ( 20.50609665440969565, 12.85937500000000000, -20.50609665441004736 ) ) ;
#8044=CARTESIAN_POINT ( 'NONE',  ( -28.02196122052045268, 16.30246500092397355, 7.468012846824790607 ) ) ;
#8065=CARTESIAN_POINT ( 'NONE',  ( 6.950374756619721595, 32.63059000092395934, 26.09010956794232428 ) ) ;
#8072=CARTESIAN_POINT ( 'NONE',  ( 14.97647472619900455, 45.65326416574269786, -26.02091320914876960 ) ) ;
#8075=SHAPE_REPRESENTATION ( 'Linear Compliance Spring & Shaft', ( #1376 ), #13943 ) ;
#8077=CARTESIAN_POINT ( 'NONE',  ( 26.07999730980477437, 16.58333333333333215, -6.988114217768290004 ) ) ;
#8081=CARTESIAN_POINT ( 'NONE',  ( -2.584737979205441561E-13, 19.30468749999999645, -30.02300923189239512 ) ) ;
#8085=CARTESIAN_POINT ( 'NONE',  ( -20.47846945139902175, 40.93788166759063785, -20.53372385742072481 ) ) ;
#8087=CARTESIAN_POINT ( 'NONE',  ( 26.00068869287367335, 51.38802083333332149, 15.01150461594596308 ) ) ;
#8097=CARTESIAN_POINT ( 'NONE',  ( 15.01150461594596486, 23.02864583333332504, -26.00068869287367690 ) ) ;
#8102=CARTESIAN_POINT ( 'NONE',  ( 14.01125832528330051, 33.04909749907601935, 24.18731323226221974 ) ) ;
#8109=CARTESIAN_POINT ( 'NONE',  ( 24.20753774853731244, 57.69010416666667140, -13.97622843553632599 ) ) ;
#8113=CARTESIAN_POINT ( 'NONE',  ( 2.584737979205442066E-13, 45.08593750000000000, 27.95245687107223276 ) ) ;
#8114=CARTESIAN_POINT ( 'NONE',  ( -20.47846945139902175, 27.18788166759063785, -20.53372385742072481 ) ) ;
#8115=CARTESIAN_POINT ( 'NONE',  ( 20.53372385742108008, 19.15586833240934794, 20.47846945139866648 ) ) ;
#8120=CARTESIAN_POINT ( 'NONE',  ( 14.01125832528330051, 46.79909749907603356, 24.18731323226221974 ) ) ;
#8126=CARTESIAN_POINT ( 'NONE',  ( -26.06988505166735237, 47.52642333425731636, -7.025853678916388567 ) ) ;
#8130=CARTESIAN_POINT ( 'NONE',  ( -26.00068869287368756, 29.04427083333332504, -15.01150461594595775 ) ) ;
#8135=CARTESIAN_POINT ( 'NONE',  ( 20.50609665440969565, 47.23437499999999289, -20.50609665441004736 ) ) ;
#8141=CARTESIAN_POINT ( 'NONE',  ( -7.468012846824272799, 64.41628499907602645, 28.02196122052058413 ) ) ;
#8146=CARTESIAN_POINT ( 'NONE',  ( -27.95245687107223276, 59.69531250000000711, 2.498001805406602216E-13 ) ) ;
#8149=CARTESIAN_POINT ( 'NONE',  ( -24.20753774853730889, 28.47135416666666075, 13.97622843553633842 ) ) ;
#8154=CARTESIAN_POINT ( 'NONE',  ( -13.94119854578936923, 61.70611083425731636, -24.22776226481241224 ) ) ;
#8164=CARTESIAN_POINT ( 'NONE',  ( 26.09010956794232428, 14.58371500092397710, -6.950374756619718042 ) ) ;
#8169=CARTESIAN_POINT ( 'NONE',  ( 30.02300923189239512, 40.78906249999998579, -2.619432448724977703E-13 ) ) ;
#8172=CARTESIAN_POINT ( 'NONE',  ( -30.02300923189239512, 18.44531249999999645, 2.654126918244515359E-13 ) ) ;
#8179=CARTESIAN_POINT ( 'NONE',  ( 14.97647472619900455, 35.34076416574268364, -26.02091320914876960 ) ) ;
#8181=CARTESIAN_POINT ( 'NONE',  ( -7.505752307973343918, 53.53645833333332860, -28.01184896238290989 ) ) ;
#8187=CARTESIAN_POINT ( 'NONE',  ( 26.09010956794244507, 60.11940999907602645, 6.950374756619249084 ) ) ;
#8193=CARTESIAN_POINT ( 'NONE',  ( -13.97622843553632777, 22.45572916666666430, -24.20753774853731599 ) ) ;
#8200=CARTESIAN_POINT ( 'NONE',  ( -13.94119854578892514, 23.30951416574269075, 24.22776226481266448 ) ) ;
#8204=CARTESIAN_POINT ( 'NONE',  ( 6.988114217768294445, 44.94270833333332860, 26.07999730980477437 ) ) ;
#8208=CARTESIAN_POINT ( 'NONE',  ( -20.50609665440969209, 18.01562499999999645, 20.50609665441005092 ) ) ;
#8209=CARTESIAN_POINT ( 'NONE',  ( 25.98046417659858420, 18.45090250092397355, 15.04653450569292872 ) ) ;
#8228=CARTESIAN_POINT ( 'NONE',  ( -24.18731323226248264, 33.91965250092398065, -14.01125832528284931 ) ) ;
#8235=CARTESIAN_POINT ( 'NONE',  ( -20.47846945139866648, 44.07774333240935505, 20.53372385742108008 ) ) ;
#8239=CARTESIAN_POINT ( 'NONE',  ( -19.09188309203694445, 18.87499999999999645, -19.09188309203661049 ) ) ;
#8241=CARTESIAN_POINT ( 'NONE',  ( -15.01150461594642138, 22.45572916666666430, -26.00068869287340334 ) ) ;
#8245=CARTESIAN_POINT ( 'NONE',  ( -14.97647472619946285, 37.64361083425730925, -26.02091320914851025 ) ) ;
#8247=CARTESIAN_POINT ( 'NONE',  ( -7.505752307972844761, 55.54166666666667140, 28.01184896238304134 ) ) ;
#8248=CARTESIAN_POINT ( 'NONE',  ( 7.505752307973351023, 65.56770833333332860, 28.01184896238290278 ) ) ;
#8258=CARTESIAN_POINT ( 'NONE',  ( 28.01184896238304134, 20.30729166666666430, 7.505752307972846538 ) ) ;
#8269=CARTESIAN_POINT ( 'NONE',  ( -13.97622843553632421, 60.26822916666665009, -24.20753774853731599 ) ) ;
#8273=CARTESIAN_POINT ( 'NONE',  ( 19.09188309203661049, 43.79687500000000000, -19.09188309203694445 ) ) ;
#8274=CARTESIAN_POINT ( 'NONE',  ( 28.00173670424549499, 32.05767333425730214, 7.543491769121417612 ) ) ;
#8275=CARTESIAN_POINT ( 'NONE',  ( -25.98046417659831420, 23.59597249907602290, 15.04653450569339945 ) ) ;
#8279=CARTESIAN_POINT ( 'NONE',  ( 27.95245687107223276, 42.78868083240935505, -0.04044903255042905932 ) ) ;
#8287=CARTESIAN_POINT ( 'NONE',  ( -19.06425588902591173, 51.25038166759065206, -19.11951029504763611 ) ) ;
#8291=CARTESIAN_POINT ( 'NONE',  ( 20.50609665441005092, 27.46875000000000000, 20.50609665440969209 ) ) ;
#8295=CARTESIAN_POINT ( 'NONE',  ( 2.740863092043355209E-13, 48.52343750000000000, 30.02300923189239512 ) ) ;
#8301=CARTESIAN_POINT ( 'NONE',  ( -14.97647472619899389, 57.68451416574269075, 26.02091320914878025 ) ) ;
#8304=ADVANCED_FACE ( 'NONE', ( #5221 ), #22909, .T. ) ;
#8306=CARTESIAN_POINT ( 'NONE',  ( 24.20753774853756113, 61.70052083333332860, 13.97622843553589789 ) ) ;
#8309=CARTESIAN_POINT ( 'NONE',  ( 2.584737979205441561E-13, 27.89843750000000000, 27.95245687107222921 ) ) ;
#8315=CARTESIAN_POINT ( 'NONE',  ( -19.06425588902591173, 58.12538166759063785, -19.11951029504763611 ) ) ;
#8329=CARTESIAN_POINT ( 'NONE',  ( 26.09010956794232428, 24.89621500092397710, -6.950374756619718042 ) ) ;
#8334=CARTESIAN_POINT ( 'NONE',  ( 28.01184896238304134, 54.68229166666665719, 7.505752307972846538 ) ) ;
#8338=CARTESIAN_POINT ( 'NONE',  ( -20.50609665440969209, 18.01562499999999645, 20.50609665441005092 ) ) ;
#8344=CARTESIAN_POINT ( 'NONE',  ( -7.468012846824272799, 33.47878499907601935, 28.02196122052058413 ) ) ;
#8346=CARTESIAN_POINT ( 'NONE',  ( -7.505752307973343918, 46.66145833333332860, -28.01184896238290989 ) ) ;
#8349=CARTESIAN_POINT ( 'NONE',  ( 14.01125832528330051, 60.54909749907603356, 24.18731323226221974 ) ) ;
#8357=CARTESIAN_POINT ( 'NONE',  ( -13.97622843553632777, 19.01822916666666430, -24.20753774853731599 ) ) ;
#8364=CARTESIAN_POINT ( 'NONE',  ( -24.18731323226221974, 30.47097249907602290, 14.01125832528330406 ) ) ;
#8369=CARTESIAN_POINT ( 'NONE',  ( -24.20753774853756823, 53.10677083333331439, -13.97622843553588723 ) ) ;
#8373=CARTESIAN_POINT ( 'NONE',  ( 2.740863092043355209E-13, 17.58593749999999645, 30.02300923189239512 ) ) ;
#8374=CARTESIAN_POINT ( 'NONE',  ( 30.02300923189239867, 11.28944416759064140, 0.04044903254992252006 ) ) ;
#8395=CARTESIAN_POINT ( 'NONE',  ( -19.06425588902591173, 40.93788166759063785, -19.11951029504763611 ) ) ;
#8403=CARTESIAN_POINT ( 'NONE',  ( -20.47846945139866648, 57.82774333240935505, 20.53372385742108008 ) ) ;
#8407=CARTESIAN_POINT ( 'NONE',  ( -19.09188309203660694, 14.57812499999999645, 19.09188309203694800 ) ) ;
#8410=CARTESIAN_POINT ( 'NONE',  ( -20.50609665440969209, 28.32812499999999645, 20.50609665441005092 ) ) ;
#8413=CARTESIAN_POINT ( 'NONE',  ( -20.53372385742071771, 40.07850666759064495, 20.47846945139902530 ) ) ;
#8415=CARTESIAN_POINT ( 'NONE',  ( -26.00068869287340334, 55.97135416666665719, 15.01150461594643382 ) ) ;
#8426=CARTESIAN_POINT ( 'NONE',  ( -20.50609665440969209, 18.01562499999999645, 20.50609665441005092 ) ) ;
#8437=CARTESIAN_POINT ( 'NONE',  ( 26.07999730980477437, 61.27083333333332860, -6.988114217768290004 ) ) ;
#8442=CARTESIAN_POINT ( 'NONE',  ( -19.09188309203660694, 52.39062499999999289, 19.09188309203694800 ) ) ;
#8443=CARTESIAN_POINT ( 'NONE',  ( -26.02091320914849959, 33.34673583425730214, 14.97647472619947528 ) ) ;
#8444=CARTESIAN_POINT ( 'NONE',  ( -7.468012846824272799, 23.16628499907601579, 28.02196122052058413 ) ) ;
#8449=CARTESIAN_POINT ( 'NONE',  ( 14.01125832528330051, 50.23659749907603356, 24.18731323226221974 ) ) ;
#8457=CARTESIAN_POINT ( 'NONE',  ( 7.025853678916403666, 55.26079833425730214, -26.06988505166735237 ) ) ;
#8461=CARTESIAN_POINT ( 'NONE',  ( -28.01184896238290278, 21.73958333333332860, 7.505752307973363457 ) ) ;
#8465=CARTESIAN_POINT ( 'NONE',  ( -26.00068869287340334, 49.09635416666665719, 15.01150461594643382 ) ) ;
#8474=CARTESIAN_POINT ( 'NONE',  ( -19.06425588902558133, 20.01524333240935505, 19.11951029504797006 ) ) ;
#8481=CARTESIAN_POINT ( 'NONE',  ( -24.20753774853756823, 32.48177083333332860, -13.97622843553588723 ) ) ;
#8486=CARTESIAN_POINT ( 'NONE',  ( -24.22776226481240514, 53.97173583425732346, 13.94119854578937812 ) ) ;
#8498=CARTESIAN_POINT ( 'NONE',  ( 14.01125832528286352, 27.90402750092397355, -24.18731323226246843 ) ) ;
#8503=CARTESIAN_POINT ( 'NONE',  ( -7.505752307973343918, 50.09895833333332860, -28.01184896238290989 ) ) ;
#8507=CARTESIAN_POINT ( 'NONE',  ( -28.01184896238290278, 25.17708333333332860, 7.505752307973363457 ) ) ;
#8515=CARTESIAN_POINT ( 'NONE',  ( -20.53372385742107653, 38.06211833240934084, -20.47846945139867003 ) ) ;
#8517=CARTESIAN_POINT ( 'NONE',  ( 28.01184896238290278, 47.52083333333332860, -7.505752307973347470 ) ) ;
#8522=CARTESIAN_POINT ( 'NONE',  ( 19.06425588902558133, 59.54649333240936215, -19.11951029504797006 ) ) ;
#8528=CARTESIAN_POINT ( 'NONE',  ( 6.988114217768294445, 20.88020833333333215, 26.07999730980477437 ) ) ;
#8537=CARTESIAN_POINT ( 'NONE',  ( -6.950374756619247307, 26.60378499907601579, 26.09010956794245217 ) ) ;
#8539=PRODUCT_DEFINITION_SHAPE ( 'NONE', 'NONE',  #12245 ) ;
#8541=CARTESIAN_POINT ( 'NONE',  ( -24.20753774853730889, 49.09635416666665719, 13.97622843553633842 ) ) ;
#8545=CARTESIAN_POINT ( 'NONE',  ( -20.50609665440969209, 28.32812499999999645, 20.50609665441005092 ) ) ;
#8546=CARTESIAN_POINT ( 'NONE',  ( 28.02196122052045268, 21.45871500092397355, -7.468012846824774620 ) ) ;
#8567=CARTESIAN_POINT ( 'NONE',  ( 26.06988505166735592, 42.37017333425730925, 7.025853678916393896 ) ) ;
#8575=CARTESIAN_POINT ( 'NONE',  ( 7.468012846824281681, 59.26003499907601935, -28.02196122052058058 ) ) ;
#8579=CARTESIAN_POINT ( 'NONE',  ( -13.97622843553632421, 22.45572916666666430, -24.20753774853731599 ) ) ;
#8581=CARTESIAN_POINT ( 'NONE',  ( -28.01184896238304134, 32.33854166666666430, -7.505752307972844761 ) ) ;
#8584=CARTESIAN_POINT ( 'NONE',  ( -25.98046417659859486, 47.66965250092398065, -15.04653450569291628 ) ) ;
#8586=CARTESIAN_POINT ( 'NONE',  ( -20.50609665441004736, 49.81249999999999289, -20.50609665440969565 ) ) ;
#8587=CARTESIAN_POINT ( 'NONE',  ( -28.01184896238290278, 66.42708333333332860, 7.505752307973363457 ) ) ;
#8608=CARTESIAN_POINT ( 'NONE',  ( 19.09188309203661049, 64.42187499999998579, -19.09188309203694445 ) ) ;
#8613=CARTESIAN_POINT ( 'NONE',  ( -24.20753774853730889, 45.65885416666666430, 13.97622843553634020 ) ) ;
#8614=CARTESIAN_POINT ( 'NONE',  ( 20.47846945139902530, 35.78163166759063074, 20.53372385742071771 ) ) ;
#8616=CARTESIAN_POINT ( 'NONE',  ( 26.02091320914876960, 32.76263916574268364, 14.97647472619900455 ) ) ;
#8619=CARTESIAN_POINT ( 'NONE',  ( -7.025853678916861966, 55.53607666574269075, -26.06988505166722803 ) ) ;
#8625=CARTESIAN_POINT ( 'NONE',  ( -0.04044903254992426173, 53.39881916759064495, 27.95245687107223276 ) ) ;
#8629=CARTESIAN_POINT ( 'NONE',  ( 20.50609665441005092, 24.03124999999999645, 20.50609665440969209 ) ) ;
#8633=CARTESIAN_POINT ( 'NONE',  ( 2.740863092043355209E-13, 58.83593750000000000, 30.02300923189239512 ) ) ;
#8634=AXIS2_PLACEMENT_3D ( 'NONE', #33719, #26332, #26166 ) ;
#8639=CARTESIAN_POINT ( 'NONE',  ( -27.95245687107223986, 20.44493083240935150, 0.04044903255043252877 ) ) ;
#8646=CARTESIAN_POINT ( 'NONE',  ( -26.07999730980477437, 38.92708333333333570, 6.988114217768305103 ) ) ;
#8652=CARTESIAN_POINT ( 'NONE',  ( -13.94119854578936923, 58.26861083425732346, -24.22776226481241224 ) ) ;
#8654=CARTESIAN_POINT ( 'NONE',  ( 28.01184896238290278, 50.95833333333332860, -7.505752307973347470 ) ) ;
#8666=CARTESIAN_POINT ( 'NONE',  ( 19.06425588902592239, 25.46913166759064140, 19.11951029504763611 ) ) ;
#8673=CARTESIAN_POINT ( 'NONE',  ( 20.50609665441005092, 51.53124999999999289, 20.50609665440969209 ) ) ;
#8677=CARTESIAN_POINT ( 'NONE',  ( -15.01150461594595775, 31.62239583333332860, 26.00068869287368756 ) ) ;
#8683=CARTESIAN_POINT ( 'NONE',  ( -20.53372385742107653, 41.49961833240934794, -20.47846945139867003 ) ) ;
#8685=CARTESIAN_POINT ( 'NONE',  ( -2.584737979205442066E-13, 50.24218750000000711, -30.02300923189239867 ) ) ;
#8688=CARTESIAN_POINT ( 'NONE',  ( -7.025853678916861966, 65.84857666574268364, -26.06988505166722803 ) ) ;
#8694=CARTESIAN_POINT ( 'NONE',  ( 2.584737979205442066E-13, 24.46093749999999645, 27.95245687107223276 ) ) ;
#8701=CARTESIAN_POINT ( 'NONE',  ( -26.09010956794245217, 24.02565999907602290, -6.950374756619243755 ) ) ;
#8705=CARTESIAN_POINT ( 'NONE',  ( 13.97622843553633665, 51.67447916666665719, 24.20753774853730889 ) ) ;
#8709=CARTESIAN_POINT ( 'NONE',  ( 7.505752307973351023, 20.88020833333333215, 28.01184896238290278 ) ) ;
#8710=CARTESIAN_POINT ( 'NONE',  ( 14.97647472619947351, 25.61236083425731636, 26.02091320914850314 ) ) ;
#8718=CARTESIAN_POINT ( 'NONE',  ( 28.00173670424549499, 59.55767333425731636, 7.543491769121417612 ) ) ;
#8725=CARTESIAN_POINT ( 'NONE',  ( 6.950374756619257965, 38.63503499907601224, -26.09010956794244507 ) ) ;
#8732=CARTESIAN_POINT ( 'NONE',  ( 19.11951029504763611, 38.35975666759064495, -19.06425588902591173 ) ) ;
#8740=CARTESIAN_POINT ( 'NONE',  ( 26.02091320914876960, 56.82513916574268364, 14.97647472619900455 ) ) ;
#8744=CARTESIAN_POINT ( 'NONE',  ( 27.95245687107222921, 30.47656250000000355, -2.463307335887066074E-13 ) ) ;
#8746=CARTESIAN_POINT ( 'NONE',  ( 28.01184896238304134, 34.05729166666666430, 7.505752307972846538 ) ) ;
#8749=CARTESIAN_POINT ( 'NONE',  ( 25.98046417659858420, 45.95090250092398065, 15.04653450569292872 ) ) ;
#8751=CARTESIAN_POINT ( 'NONE',  ( -28.01184896238304134, 59.83854166666666430, -7.505752307972844761 ) ) ;
#8770=CARTESIAN_POINT ( 'NONE',  ( -19.11951029504763611, 12.57850666759064140, 19.06425588902592239 ) ) ;
#8775=CARTESIAN_POINT ( 'NONE',  ( 24.20753774853731244, 54.25260416666666430, -13.97622843553633132 ) ) ;
#8776=CARTESIAN_POINT ( 'NONE',  ( 30.02300923189239867, 35.35194416759064495, 0.04044903254992252006 ) ) ;
#8777=CARTESIAN_POINT ( 'NONE',  ( -30.02300923189239867, 23.88243083240935505, 0.04044903255044988294 ) ) ;
#8780=CARTESIAN_POINT ( 'NONE',  ( -19.11951029504797006, 58.68711833240935505, -19.06425588902558133 ) ) ;
#8787=CARTESIAN_POINT ( 'NONE',  ( -26.06988505166735237, 50.96392333425730925, -7.025853678916388567 ) ) ;
#8791=CARTESIAN_POINT ( 'NONE',  ( 20.50609665441005092, 20.59374999999999645, 20.50609665440969209 ) ) ;
#8796=CARTESIAN_POINT ( 'NONE',  ( -7.505752307973343918, 60.41145833333332149, -28.01184896238290989 ) ) ;
#8803=CARTESIAN_POINT ( 'NONE',  ( 6.950374756619257965, 18.01003499907601935, -26.09010956794244507 ) ) ;
#8810=CARTESIAN_POINT ( 'NONE',  ( 6.988114217767829928, 40.07291666666666430, -26.07999730980489872 ) ) ;
#8816=CARTESIAN_POINT ( 'NONE',  ( -7.468012846824771955, 13.72434000092397532, -28.02196122052045624 ) ) ;
#8817=CARTESIAN_POINT ( 'NONE',  ( 20.50609665440969565, 57.54687500000000000, -20.50609665441004736 ) ) ;
#8830=CARTESIAN_POINT ( 'NONE',  ( -19.11951029504763611, 26.32850666759063785, 19.06425588902592239 ) ) ;
#8836=CARTESIAN_POINT ( 'NONE',  ( 26.00068869287367335, 54.82552083333331439, 15.01150461594596308 ) ) ;
#8840=CARTESIAN_POINT ( 'NONE',  ( -15.01150461594642138, 25.89322916666666430, -26.00068869287340334 ) ) ;
#8846=CARTESIAN_POINT ( 'NONE',  ( -26.02091320914878025, 41.35638916574269075, -14.97647472619899389 ) ) ;
#8849=CARTESIAN_POINT ( 'NONE',  ( 7.505752307973351023, 48.38020833333332860, 28.01184896238290278 ) ) ;
#8852=CARTESIAN_POINT ( 'NONE',  ( 6.988114217767829928, 12.57291666666666252, -26.07999730980489872 ) ) ;
#8858=CARTESIAN_POINT ( 'NONE',  ( 27.95245687107223276, 20.16406249999999645, -2.463307335887066074E-13 ) ) ;
#8864=CARTESIAN_POINT ( 'NONE',  ( 28.00173670424535644, 28.89545166574268009, -7.543491769121920321 ) ) ;
#8867=CARTESIAN_POINT ( 'NONE',  ( 26.09010956794244507, 25.74440999907601935, 6.950374756619249084 ) ) ;
#8871=CARTESIAN_POINT ( 'NONE',  ( 13.97622843553589966, 50.52864583333333570, -24.20753774853756113 ) ) ;
#8876=CARTESIAN_POINT ( 'NONE',  ( -26.00068869287368756, 22.16927083333332504, -15.01150461594595775 ) ) ;
#8877=CARTESIAN_POINT ( 'NONE',  ( -30.02300923189239867, 19.88319416759064495, -0.04044903254991731589 ) ) ;
#8886=CARTESIAN_POINT ( 'NONE',  ( -0.04044903254990864921, 60.27381916759065206, 30.02300923189239867 ) ) ;
#8892=CARTESIAN_POINT ( 'NONE',  ( -7.025853678916861966, 41.78607666574268364, -26.06988505166722803 ) ) ;
#8898=CARTESIAN_POINT ( 'NONE',  ( -0.04044903254992426173, 36.21131916759064495, 27.95245687107223276 ) ) ;
#8905=CARTESIAN_POINT ( 'NONE',  ( 28.02196122052058413, 53.24440999907603356, 7.468012846824272799 ) ) ;
#8909=CARTESIAN_POINT ( 'NONE',  ( -24.20753774853730889, 28.47135416666666075, 13.97622843553633842 ) ) ;
#8913=CARTESIAN_POINT ( 'NONE',  ( -28.01184896238304134, 28.90104166666666785, -7.505752307972844761 ) ) ;
#8916=CARTESIAN_POINT ( 'NONE',  ( 28.00173670424549499, 45.80767333425730925, 7.543491769121417612 ) ) ;
#8919=CARTESIAN_POINT ( 'NONE',  ( 28.01184896238290278, 57.83333333333333570, -7.505752307973347470 ) ) ;
#8943=CARTESIAN_POINT ( 'NONE',  ( -24.20753774853730889, 66.28385416666662877, 13.97622843553633842 ) ) ;
#8948=CARTESIAN_POINT ( 'NONE',  ( 24.20753774853731244, 47.37760416666666430, -13.97622843553633132 ) ) ;
#8949=CARTESIAN_POINT ( 'NONE',  ( 7.468012846824777284, 36.06809000092397355, 28.02196122052045268 ) ) ;
#8950=CARTESIAN_POINT ( 'NONE',  ( -15.04653450569338524, 24.45534749907602290, -25.98046417659831775 ) ) ;
#8953=CARTESIAN_POINT ( 'NONE',  ( 7.025853678916867295, 57.25482666574269075, 26.06988505166722803 ) ) ;
#8961=CARTESIAN_POINT ( 'NONE',  ( 30.02300923189239512, 33.91406249999997158, -2.619432448724977703E-13 ) ) ;
#8966=CARTESIAN_POINT ( 'NONE',  ( 20.50609665441005092, 58.40625000000000711, 20.50609665440969209 ) ) ;
#8973=CARTESIAN_POINT ( 'NONE',  ( -20.53372385742107653, 68.99961833240934084, -20.47846945139867003 ) ) ;
#8981=CARTESIAN_POINT ( 'NONE',  ( -24.20753774853756823, 39.35677083333331439, -13.97622843553588723 ) ) ;
#8988=CARTESIAN_POINT ( 'NONE',  ( 15.04653450569292872, 14.15402750092397532, -25.98046417659857710 ) ) ;
#8989=CARTESIAN_POINT ( 'NONE',  ( -30.02300923189239512, 56.25781249999997868, 2.654126918244515359E-13 ) ) ;
#9000=CARTESIAN_POINT ( 'NONE',  ( -14.01125832528285109, 22.74777750092397355, 24.18731323226248264 ) ) ;
#9004=STYLED_ITEM ( 'NONE', ( #20945 ), #18554 ) ;
#9006=CARTESIAN_POINT ( 'NONE',  ( 28.01184896238304134, 47.80729166666666430, 7.505752307972846538 ) ) ;
#9010=CARTESIAN_POINT ( 'NONE',  ( -2.584737979205441561E-13, 29.61718749999999645, -30.02300923189239512 ) ) ;
#9014=CARTESIAN_POINT ( 'NONE',  ( 30.02300923189239867, 39.35118083240935505, -0.04044903255044467877 ) ) ;
#9016=CARTESIAN_POINT ( 'NONE',  ( 15.01150461594643382, 58.54947916666666430, 26.00068869287340334 ) ) ;
#9020=CARTESIAN_POINT ( 'NONE',  ( -27.95245687107222921, 18.44531249999999645, 2.498001805406602216E-13 ) ) ;
#9028=CARTESIAN_POINT ( 'NONE',  ( 13.97622843553633842, 31.04947916666666430, 24.20753774853730889 ) ) ;
#9034=CARTESIAN_POINT ( 'NONE',  ( 30.02300923189239867, 25.60118083240935860, -0.04044903255044467877 ) ) ;
#9036=CARTESIAN_POINT ( 'NONE',  ( -26.09010956794245217, 30.90065999907601579, -6.950374756619243755 ) ) ;
#9040=CARTESIAN_POINT ( 'NONE',  ( 26.07999730980477437, 54.39583333333332860, -6.988114217768290004 ) ) ;
#9045=CARTESIAN_POINT ( 'NONE',  ( 26.00068869287367335, 23.88802083333331794, 15.01150461594596308 ) ) ;
#9046=CARTESIAN_POINT ( 'NONE',  ( 0.04044903254992426173, 27.61756916759064140, -30.02300923189239867 ) ) ;
#9055=CARTESIAN_POINT ( 'NONE',  ( -20.47846945139902175, 58.12538166759063785, -20.53372385742072481 ) ) ;
#9058=CARTESIAN_POINT ( 'NONE',  ( 26.00068869287367690, 34.20052083333332149, 15.01150461594596486 ) ) ;
#9062=CARTESIAN_POINT ( 'NONE',  ( 27.95245687107223276, 46.22618083240936215, -0.04044903255042905932 ) ) ;
#9069=CARTESIAN_POINT ( 'NONE',  ( 13.94119854578937812, 35.92486083425730214, 24.22776226481240514 ) ) ;
#9076=CARTESIAN_POINT ( 'NONE',  ( -7.543491769121917656, 52.09857666574269075, -28.00173670424536354 ) ) ;
#9079=CARTESIAN_POINT ( 'NONE',  ( -24.20753774853730889, 21.59635416666666785, 13.97622843553633842 ) ) ;
#9082=CARTESIAN_POINT ( 'NONE',  ( 2.740863092043355209E-13, 31.33593749999999289, 30.02300923189239512 ) ) ;
#9085=CARTESIAN_POINT ( 'NONE',  ( -20.53372385742071771, 53.82850666759064495, 20.47846945139902530 ) ) ;
#9088=CARTESIAN_POINT ( 'NONE',  ( -26.00068869287340334, 62.84635416666667851, 15.01150461594643382 ) ) ;
#9107=CARTESIAN_POINT ( 'NONE',  ( -26.09010956794232428, 12.86496500092397710, 6.950374756619732253 ) ) ;
#9112=CARTESIAN_POINT ( 'NONE',  ( -26.07999730980490583, 49.52604166666666430, -6.988114217767815717 ) ) ;
#9113=CARTESIAN_POINT ( 'NONE',  ( -28.00173670424549499, 37.21392333425730214, -7.543491769121417612 ) ) ;
#9114=CARTESIAN_POINT ( 'NONE',  ( -15.04653450569338524, 31.33034749907602290, -25.98046417659831775 ) ) ;
#9117=CARTESIAN_POINT ( 'NONE',  ( -24.18731323226221974, 54.53347249907601935, 14.01125832528330406 ) ) ;
#9125=CARTESIAN_POINT ( 'NONE',  ( -7.505752307972844761, 38.35416666666666430, 28.01184896238304134 ) ) ;
#9130=CARTESIAN_POINT ( 'NONE',  ( 26.00068869287367335, 58.26302083333332149, 15.01150461594596308 ) ) ;
#9138=CARTESIAN_POINT ( 'NONE',  ( 19.06425588902558133, 18.29649333240935150, -19.11951029504797006 ) ) ;
#9145=CARTESIAN_POINT ( 'NONE',  ( 6.988114217768294445, 38.06770833333332860, 26.07999730980477437 ) ) ;
#9151=CARTESIAN_POINT ( 'NONE',  ( 26.09010956794232428, 62.70871500092398065, -6.950374756619718042 ) ) ;
#9152=CARTESIAN_POINT ( 'NONE',  ( 15.01150461594643204, 51.67447916666665719, 26.00068869287340334 ) ) ;
#9163=CARTESIAN_POINT ( 'NONE',  ( -27.95245687107223986, 30.19569416759064140, -0.04044903254993292840 ) ) ;
#9168=CARTESIAN_POINT ( 'NONE',  ( -2.584737979205441561E-13, 60.55468749999999289, -30.02300923189239512 ) ) ;
#9172=CARTESIAN_POINT ( 'NONE',  ( 26.00068869287367335, 34.20052083333332860, 15.01150461594596308 ) ) ;
#9177=CARTESIAN_POINT ( 'NONE',  ( 7.468012846824281681, 45.51003499907601935, -28.02196122052058058 ) ) ;
#9179=CARTESIAN_POINT ( 'NONE',  ( 15.01150461594596486, 53.96614583333333570, -26.00068869287367690 ) ) ;
#9183=CARTESIAN_POINT ( 'NONE',  ( -6.950374756619247307, 67.85378499907602645, 26.09010956794245217 ) ) ;
#9189=CARTESIAN_POINT ( 'NONE',  ( 24.20753774853756113, 34.20052083333332149, 13.97622843553589789 ) ) ;
#9193=CARTESIAN_POINT ( 'NONE',  ( -14.97647472619899389, 26.74701416574268720, 26.02091320914878025 ) ) ;
#9195=CARTESIAN_POINT ( 'NONE',  ( -24.18731323226221974, 37.34597249907603356, 14.01125832528330406 ) ) ;
#9199=CARTESIAN_POINT ( 'NONE',  ( 13.97622843553633665, 61.98697916666665009, 24.20753774853730889 ) ) ;
#9205=CARTESIAN_POINT ( 'NONE',  ( 28.01184896238290278, 23.45833333333333215, -7.505752307973347470 ) ) ;
#9206=CARTESIAN_POINT ( 'NONE',  ( 7.543491769121427382, 27.76079833425730925, -28.00173670424548433 ) ) ;
#9216=CARTESIAN_POINT ( 'NONE',  ( 14.97647472619947351, 56.54986083425731636, 26.02091320914850314 ) ) ;
#9219=CARTESIAN_POINT ( 'NONE',  ( -26.00068869287340334, 28.47135416666666430, 15.01150461594643559 ) ) ;
#9223=CARTESIAN_POINT ( 'NONE',  ( 26.09010956794244507, 39.49440999907601224, 6.950374756619249084 ) ) ;
#9229=CARTESIAN_POINT ( 'NONE',  ( -24.18731323226248264, 47.66965250092398065, -14.01125832528284931 ) ) ;
#9236=CARTESIAN_POINT ( 'NONE',  ( -0.04044903255044120238, 65.99180583240935505, -30.02300923189239867 ) ) ;
#9240=CARTESIAN_POINT ( 'NONE',  ( -19.09188309203660694, 24.89062500000000000, 19.09188309203694800 ) ) ;
#9243=CARTESIAN_POINT ( 'NONE',  ( -26.00068869287340334, 42.22135416666666430, 15.01150461594643382 ) ) ;
#9246=ORIENTED_EDGE ( 'NONE', *, *, #28799, .F. ) ;
#9247=CARTESIAN_POINT ( 'NONE',  ( 30.02300923189239867, 49.10194416759064495, 0.04044903254992252006 ) ) ;
#9250=CARTESIAN_POINT ( 'NONE',  ( 30.02300923189239512, 57.97656249999997868, -2.619432448724977703E-13 ) ) ;
#9269=CARTESIAN_POINT ( 'NONE',  ( -14.01125832528285109, 12.43527750092397532, 24.18731323226248264 ) ) ;
#9274=CARTESIAN_POINT ( 'NONE',  ( 19.09188309203694800, 54.96875000000000000, 19.09188309203660694 ) ) ;
#9275=CARTESIAN_POINT ( 'NONE',  ( 26.02091320914851025, 41.94048583425730925, -14.97647472619946463 ) ) ;
#9276=CARTESIAN_POINT ( 'NONE',  ( -28.00173670424535644, 27.17670166574268009, 7.543491769121936308 ) ) ;
#9279=CARTESIAN_POINT ( 'NONE',  ( 26.06988505166722803, 52.95795166574269075, -7.025853678916862854 ) ) ;
#9287=CARTESIAN_POINT ( 'NONE',  ( -7.505752307973343918, 32.91145833333332860, -28.01184896238290989 ) ) ;
#9291=CARTESIAN_POINT ( 'NONE',  ( 28.01184896238304134, 54.68229166666665719, 7.505752307972846538 ) ) ;
#9299=CARTESIAN_POINT ( 'NONE',  ( 26.09010956794244507, 29.18190999907601579, 6.950374756619249084 ) ) ;
#9307=CARTESIAN_POINT ( 'NONE',  ( 2.584737979205441561E-13, 45.08593750000000711, 27.95245687107222921 ) ) ;
#9312=CARTESIAN_POINT ( 'NONE',  ( 20.53372385742072481, 14.29725666759064318, -20.47846945139902175 ) ) ;
#9313=CARTESIAN_POINT ( 'NONE',  ( 26.00068869287367335, 51.38802083333332149, 15.01150461594596308 ) ) ;
#9323=CARTESIAN_POINT ( 'NONE',  ( -7.025853678916393008, 36.35454833425730925, 26.06988505166735592 ) ) ;
#9329=CARTESIAN_POINT ( 'NONE',  ( -7.505752307972844761, 58.97916666666666430, 28.01184896238304134 ) ) ;
#9333=CARTESIAN_POINT ( 'NONE',  ( 7.505752307972854531, 33.19791666666665719, -28.01184896238303423 ) ) ;
#9339=CARTESIAN_POINT ( 'NONE',  ( -28.00173670424535644, 44.36420166574269075, 7.543491769121936308 ) ) ;
#9341=CARTESIAN_POINT ( 'NONE',  ( -15.01150461594595775, 55.68489583333332860, 26.00068869287368756 ) ) ;
#9347=CARTESIAN_POINT ( 'NONE',  ( 27.95245687107222921, 16.72656249999999645, -2.463307335887066074E-13 ) ) ;
#9359=CARTESIAN_POINT ( 'NONE',  ( 15.04653450569339945, 22.73659749907601935, 25.98046417659831775 ) ) ;
#9361=CARTESIAN_POINT ( 'NONE',  ( 13.94119854578893580, 35.34076416574268364, -24.22776226481265383 ) ) ;
#9365=CARTESIAN_POINT ( 'NONE',  ( -27.95245687107222921, 59.69531250000000711, 2.498001805406602216E-13 ) ) ;
#9370=CARTESIAN_POINT ( 'NONE',  ( 28.01184896238304134, 37.49479166666666430, 7.505752307972846538 ) ) ;
#9371=CARTESIAN_POINT ( 'NONE',  ( 28.00173670424549499, 32.05767333425730214, 7.543491769121417612 ) ) ;
#9382=CARTESIAN_POINT ( 'NONE',  ( 20.53372385742072481, 58.98475666759065206, -20.47846945139902175 ) ) ;
#9385=CARTESIAN_POINT ( 'NONE',  ( -7.505752307972844761, 31.47916666666666075, 28.01184896238304134 ) ) ;
#9389=CARTESIAN_POINT ( 'NONE',  ( -26.09010956794245217, 44.65065999907601935, -6.950374756619243755 ) ) ;
#9393=CARTESIAN_POINT ( 'NONE',  ( -19.79898987322349768, 11.99999999999999645, -19.79898987322315307 ) ) ;
#9395=CARTESIAN_POINT ( 'NONE',  ( 6.950374756619721595, 46.38059000092397355, 26.09010956794232428 ) ) ;
#9404=CARTESIAN_POINT ( 'NONE',  ( 14.97647472619900455, 66.27826416574268364, -26.02091320914876960 ) ) ;
#9409=CARTESIAN_POINT ( 'NONE',  ( 13.97622843553589966, 36.77864583333332860, -24.20753774853756113 ) ) ;
#9412=CARTESIAN_POINT ( 'NONE',  ( -26.00068869287368756, 39.35677083333331439, -15.01150461594595775 ) ) ;
#9415=CARTESIAN_POINT ( 'NONE',  ( -15.04653450569291984, 57.12277750092398065, 25.98046417659859486 ) ) ;
#9416=CARTESIAN_POINT ( 'NONE',  ( -26.06988505166735237, 61.27642333425730925, -7.025853678916388567 ) ) ;
#9418=CARTESIAN_POINT ( 'NONE',  ( -15.01150461594595775, 65.99739583333334281, 26.00068869287368756 ) ) ;
#9438=CARTESIAN_POINT ( 'NONE',  ( 24.22776226481241224, 17.87798583425730570, -13.94119854578936923 ) ) ;
#9446=CARTESIAN_POINT ( 'NONE',  ( -15.04653450569291984, 46.81027750092398776, 25.98046417659859486 ) ) ;
#9449=CARTESIAN_POINT ( 'NONE',  ( 30.02300923189239867, 35.91368083240935505, -0.04044903255044467877 ) ) ;
#9452=CARTESIAN_POINT ( 'NONE',  ( -24.22776226481266448, 68.85638916574269786, -13.94119854578892514 ) ) ;
#9455=CARTESIAN_POINT ( 'NONE',  ( 15.01150461594643204, 13.86197916666666430, 26.00068869287340334 ) ) ;
#9462=CARTESIAN_POINT ( 'NONE',  ( -15.01150461594642138, 36.20572916666666430, -26.00068869287340334 ) ) ;
#9478=CARTESIAN_POINT ( 'NONE',  ( -26.06988505166722803, 27.17670166574268009, 7.025853678916877953 ) ) ;
#9486=CARTESIAN_POINT ( 'NONE',  ( 26.07999730980490227, 47.80729166666666430, 6.988114217767821046 ) ) ;
#9491=CARTESIAN_POINT ( 'NONE',  ( -15.04653450569291984, 15.87277750092397710, 25.98046417659859486 ) ) ;
#9493=CARTESIAN_POINT ( 'NONE',  ( -15.01150461594595775, 62.55989583333332860, 26.00068869287368756 ) ) ;
#9505=CARTESIAN_POINT ( 'NONE',  ( 13.94119854578937812, 29.04986083425730570, 24.22776226481240514 ) ) ;
#9510=CARTESIAN_POINT ( 'NONE',  ( 15.01150461594596308, 64.27864583333332860, -26.00068869287367335 ) ) ;
#9514=CARTESIAN_POINT ( 'NONE',  ( -20.50609665440969209, 35.20312500000000000, 20.50609665441005092 ) ) ;
#9519=CARTESIAN_POINT ( 'NONE',  ( 7.543491769121922985, 53.81732666574268364, 28.00173670424535644 ) ) ;
#9522=CARTESIAN_POINT ( 'NONE',  ( 7.505752307972854531, 57.26041666666666430, -28.01184896238303423 ) ) ;
#9527=CARTESIAN_POINT ( 'NONE',  ( -13.97622843553632421, 19.01822916666666785, -24.20753774853731599 ) ) ;
#9537=CARTESIAN_POINT ( 'NONE',  ( -25.98046417659831420, 27.03347249907602290, 15.04653450569339945 ) ) ;
#9539=CARTESIAN_POINT ( 'NONE',  ( -19.06425588902558133, 33.76524333240934084, 19.11951029504797006 ) ) ;
#9544=CARTESIAN_POINT ( 'NONE',  ( 26.07999730980490227, 61.55729166666666430, 6.988114217767821046 ) ) ;
#9550=CARTESIAN_POINT ( 'NONE',  ( -30.02300923189239512, 32.19531250000000000, 2.654126918244515359E-13 ) ) ;
#9551=CARTESIAN_POINT ( 'NONE',  ( 28.00173670424549499, 28.62017333425730925, 7.543491769121417612 ) ) ;
#9563=CARTESIAN_POINT ( 'NONE',  ( -7.505752307973343918, 15.72395833333332860, -28.01184896238290989 ) ) ;
#9565=CARTESIAN_POINT ( 'NONE',  ( -2.584737979205442066E-13, 29.61718749999999645, -30.02300923189239867 ) ) ;
#9571=CARTESIAN_POINT ( 'NONE',  ( 27.95245687107223276, 39.35118083240935505, -0.04044903255042905932 ) ) ;
#9579=CARTESIAN_POINT ( 'NONE',  ( 26.06988505166735592, 49.24517333425730925, 7.025853678916393896 ) ) ;
#9585=CARTESIAN_POINT ( 'NONE',  ( 20.53372385742108008, 63.84336833240935505, 20.47846945139866648 ) ) ;
#9589=CARTESIAN_POINT ( 'NONE',  ( -13.97622843553632421, 36.20572916666666430, -24.20753774853731599 ) ) ;
#9592=CARTESIAN_POINT ( 'NONE',  ( 15.01150461594643204, 37.92447916666666430, 26.00068869287340334 ) ) ;
#9596=CARTESIAN_POINT ( 'NONE',  ( -28.00173670424549499, 57.83892333425730214, -7.543491769121417612 ) ) ;
#9597=CARTESIAN_POINT ( 'NONE',  ( 19.06425588902592239, 63.28163166759064495, 19.11951029504763611 ) ) ;
#9599=CARTESIAN_POINT ( 'NONE',  ( 15.04653450569339945, 15.86159749907602112, 25.98046417659831775 ) ) ;
#9619=CARTESIAN_POINT ( 'NONE',  ( 26.06988505166735592, 25.18267333425730214, 7.025853678916393896 ) ) ;
#9624=CARTESIAN_POINT ( 'NONE',  ( 28.02196122052045268, 48.95871500092396644, -7.468012846824774620 ) ) ;
#9625=CARTESIAN_POINT ( 'NONE',  ( 0.04044903255045854962, 33.33555583240935505, 30.02300923189239867 ) ) ;
#9629=CARTESIAN_POINT ( 'NONE',  ( -13.97622843553632421, 12.14322916666666430, -24.20753774853731599 ) ) ;
#9639=CARTESIAN_POINT ( 'NONE',  ( -15.01150461594595775, 35.05989583333332860, 26.00068869287368756 ) ) ;
#9647=APPLICATION_CONTEXT ( 'automotive_design' ) ;
#9655=CARTESIAN_POINT ( 'NONE',  ( 24.18731323226221974, 25.31472249907601579, -14.01125832528328985 ) ) ;
#9663=CARTESIAN_POINT ( 'NONE',  ( -19.09188309203694445, 53.25000000000000000, -19.09188309203661049 ) ) ;
#9668=CARTESIAN_POINT ( 'NONE',  ( 14.97647472619947351, 22.17486083425730925, 26.02091320914850314 ) ) ;
#9669=CARTESIAN_POINT ( 'NONE',  ( -20.50609665440969209, 62.70312500000000000, 20.50609665441005092 ) ) ;
#9680=CARTESIAN_POINT ( 'NONE',  ( -6.950374756619716266, 34.34934000092397355, -26.09010956794232428 ) ) ;
#9689=CARTESIAN_POINT ( 'NONE',  ( 26.00068869287340334, 37.06510416666666430, -15.01150461594642316 ) ) ;
#9694=CARTESIAN_POINT ( 'NONE',  ( 28.00173670424535644, 56.39545166574268364, -7.543491769121920321 ) ) ;
#9696=CARTESIAN_POINT ( 'NONE',  ( -20.50609665440969209, 55.82812499999999289, 20.50609665441005092 ) ) ;
#9701=CARTESIAN_POINT ( 'NONE',  ( -2.428612866367529427E-13, 19.30468749999999645, -27.95245687107222921 ) ) ;
#9713=CARTESIAN_POINT ( 'NONE',  ( -14.01125832528328985, 38.20534749907601935, -24.18731323226223040 ) ) ;
#9716=CARTESIAN_POINT ( 'NONE',  ( 13.97622843553633665, 65.42447916666667140, 24.20753774853730889 ) ) ;
#9721=CARTESIAN_POINT ( 'NONE',  ( -28.01184896238304134, 32.33854166666666430, -7.505752307972844761 ) ) ;
#9722=CARTESIAN_POINT ( 'NONE',  ( -25.98046417659859486, 33.91965250092398065, -15.04653450569291628 ) ) ;
#9732=CARTESIAN_POINT ( 'NONE',  ( 26.02091320914851025, 62.56548583425730925, -14.97647472619946463 ) ) ;
#9735=CARTESIAN_POINT ( 'NONE',  ( -20.50609665441004736, 29.18749999999999645, -20.50609665440969565 ) ) ;
#9740=CARTESIAN_POINT ( 'NONE',  ( 19.06425588902558133, 56.10899333240935505, -19.11951029504797006 ) ) ;
#9747=CARTESIAN_POINT ( 'NONE',  ( 14.01125832528286352, 48.52902750092398065, -24.18731323226246843 ) ) ;
#9754=CARTESIAN_POINT ( 'NONE',  ( -26.02091320914878025, 61.98138916574268364, -14.97647472619899389 ) ) ;
#9759=CARTESIAN_POINT ( 'NONE',  ( -24.20753774853730889, 31.90885416666666430, 13.97622843553633842 ) ) ;
#9762=CARTESIAN_POINT ( 'NONE',  ( 7.505752307973351023, 41.50520833333333570, 28.01184896238290278 ) ) ;
#9766=CARTESIAN_POINT ( 'NONE',  ( -30.02300923189239867, 61.13319416759063785, -0.04044903254991731589 ) ) ;
#9767=CARTESIAN_POINT ( 'NONE',  ( -27.95245687107223986, 57.69569416759065206, -0.04044903254993292840 ) ) ;
#9770=CARTESIAN_POINT ( 'NONE',  ( 20.53372385742108008, 15.71836833240935327, 20.47846945139866648 ) ) ;
#9795=CARTESIAN_POINT ( 'NONE',  ( -26.06988505166735237, 20.02642333425731280, -7.025853678916388567 ) ) ;
#9800=CARTESIAN_POINT ( 'NONE',  ( -14.97647472619946285, 51.39361083425730925, -26.02091320914851025 ) ) ;
#9802=CARTESIAN_POINT ( 'NONE',  ( -28.02196122052058413, 37.77565999907600514, -7.468012846824272799 ) ) ;
#9805=CARTESIAN_POINT ( 'NONE',  ( 19.06425588902558133, 62.98399333240935505, -19.11951029504797006 ) ) ;
#9814=CARTESIAN_POINT ( 'NONE',  ( 30.02300923189239512, 47.66406249999998579, -2.619432448724977703E-13 ) ) ;
#9827=CARTESIAN_POINT ( 'NONE',  ( 6.950374756619257965, 24.88503499907601935, -26.09010956794244507 ) ) ;
#9835=CARTESIAN_POINT ( 'NONE',  ( -19.09188309203694445, 46.37500000000000000, -19.09188309203661049 ) ) ;
#9839=CARTESIAN_POINT ( 'NONE',  ( 19.09188309203661049, 30.04687500000000000, -19.09188309203694445 ) ) ;
#9841=CARTESIAN_POINT ( 'NONE',  ( -28.00173670424549499, 20.02642333425731280, -7.543491769121417612 ) ) ;
#9842=CARTESIAN_POINT ( 'NONE',  ( -20.50609665440969209, 59.26562500000000000, 20.50609665441005092 ) ) ;
#9853=CARTESIAN_POINT ( 'NONE',  ( -24.18731323226248264, 33.91965250092398065, -14.01125832528284931 ) ) ;
#9857=CARTESIAN_POINT ( 'NONE',  ( 15.01150461594596308, 16.15364583333333215, -26.00068869287367335 ) ) ;
#9861=CARTESIAN_POINT ( 'NONE',  ( -28.01184896238290278, 42.36458333333332860, 7.505752307973363457 ) ) ;
#9866=CARTESIAN_POINT ( 'NONE',  ( -7.543491769121917656, 48.66107666574268364, -28.00173670424536354 ) ) ;
#9868=CARTESIAN_POINT ( 'NONE',  ( 30.02300923189239867, 64.85156249999997158, -2.619432448724978208E-13 ) ) ;
#9872=CARTESIAN_POINT ( 'NONE',  ( 19.09188309203661049, 19.73437500000000000, -19.09188309203694445 ) ) ;
#9888=CARTESIAN_POINT ( 'NONE',  ( 19.11951029504797006, 39.78086833240934794, 19.06425588902558133 ) ) ;
#9892=CARTESIAN_POINT ( 'NONE',  ( -6.988114217768288228, 63.84895833333332860, -26.07999730980477437 ) ) ;
#9897=CARTESIAN_POINT ( 'NONE',  ( 26.00068869287367335, 34.20052083333332860, 15.01150461594596308 ) ) ;
#9898=CARTESIAN_POINT ( 'NONE',  ( 15.04653450569292872, 31.34152750092398421, -25.98046417659857710 ) ) ;
#9908=CARTESIAN_POINT ( 'NONE',  ( -28.01184896238304134, 15.15104166666666252, -7.505752307972844761 ) ) ;
#9911=CARTESIAN_POINT ( 'NONE',  ( -30.02300923189239867, 35.63281249999999289, 2.654126918244514854E-13 ) ) ;
#9917=CARTESIAN_POINT ( 'NONE',  ( 26.09010956794244507, 53.24440999907603356, 6.950374756619249084 ) ) ;
#9922=CARTESIAN_POINT ( 'NONE',  ( 2.584737979205442066E-13, 14.14843749999999467, 27.95245687107223276 ) ) ;
#9930=CARTESIAN_POINT ( 'NONE',  ( 28.00173670424535644, 66.70795166574268364, -7.543491769121920321 ) ) ;
#9936=CARTESIAN_POINT ( 'NONE',  ( -13.97622843553588901, 31.62239583333332860, 24.20753774853756823 ) ) ;
#9939=CARTESIAN_POINT ( 'NONE',  ( 28.01184896238290278, 40.64583333333332860, -7.505752307973347470 ) ) ;
#9942=CARTESIAN_POINT ( 'NONE',  ( 7.543491769121427382, 62.13579833425730925, -28.00173670424548433 ) ) ;
#9943=CARTESIAN_POINT ( 'NONE',  ( 13.94119854578937812, 56.54986083425731636, 24.22776226481240514 ) ) ;
#9946=CARTESIAN_POINT ( 'NONE',  ( -26.02091320914878025, 20.73138916574268720, -14.97647472619899389 ) ) ;
#9967=CARTESIAN_POINT ( 'NONE',  ( 14.01125832528286352, 24.46652750092397355, -24.18731323226246843 ) ) ;
#9972=CARTESIAN_POINT ( 'NONE',  ( 30.02300923189239867, 45.66444416759065916, 0.04044903254992252006 ) ) ;
#9974=CARTESIAN_POINT ( 'NONE',  ( 20.47846945139867003, 35.48399333240935505, -20.53372385742107653 ) ) ;
#9978=CARTESIAN_POINT ( 'NONE',  ( 24.18731323226221974, 66.56472249907604066, -14.01125832528328985 ) ) ;
#9983=CARTESIAN_POINT ( 'NONE',  ( -2.584737979205441561E-13, 12.42968749999999289, -30.02300923189239512 ) ) ;
#9991=CARTESIAN_POINT ( 'NONE',  ( 28.01184896238290278, 44.08333333333332860, -7.505752307973347470 ) ) ;
#10001=CARTESIAN_POINT ( 'NONE',  ( -26.00068869287340334, 14.72135416666666607, 15.01150461594643559 ) ) ;
#10007=CARTESIAN_POINT ( 'NONE',  ( -24.22776226481266448, 27.60638916574269075, -13.94119854578892514 ) ) ;
#10016=CARTESIAN_POINT ( 'NONE',  ( -13.97622843553632421, 53.39322916666665009, -24.20753774853731599 ) ) ;
#10020=CARTESIAN_POINT ( 'NONE',  ( 13.97622843553633842, 27.61197916666666430, 24.20753774853730889 ) ) ;
#10021=CARTESIAN_POINT ( 'NONE',  ( 25.98046417659858420, 18.45090250092397355, 15.04653450569292872 ) ) ;
#10022=CARTESIAN_POINT ( 'NONE',  ( -20.53372385742107653, 13.99961833240935327, -20.47846945139867003 ) ) ;
#10033=CARTESIAN_POINT ( 'NONE',  ( 26.09010956794232428, 45.52121500092397355, -6.950374756619718042 ) ) ;
#10038=CARTESIAN_POINT ( 'NONE',  ( -15.01150461594642138, 15.58072916666666607, -26.00068869287340334 ) ) ;
#10041=CARTESIAN_POINT ( 'NONE',  ( -28.01184896238304134, 35.77604166666666430, -7.505752307972844761 ) ) ;
#10045=CARTESIAN_POINT ( 'NONE',  ( -20.47846945139866648, 50.95274333240935505, 20.53372385742108008 ) ) ;
#10051=CARTESIAN_POINT ( 'NONE',  ( -6.988114217767819270, 21.16666666666666430, 26.07999730980490583 ) ) ;
#10067=CARTESIAN_POINT ( 'NONE',  ( 19.11951029504763611, 14.29725666759064318, -19.06425588902591173 ) ) ;
#10071=CARTESIAN_POINT ( 'NONE',  ( 26.00068869287367335, 30.76302083333332504, 15.01150461594596308 ) ) ;
#10085=CARTESIAN_POINT ( 'NONE',  ( -0.04044903254990864921, 63.71131916759064495, 30.02300923189239867 ) ) ;
#10088=CARTESIAN_POINT ( 'NONE',  ( -7.505752307972844761, 38.35416666666666430, 28.01184896238304134 ) ) ;
#10094=CARTESIAN_POINT ( 'NONE',  ( 26.09010956794244507, 49.80690999907602645, 6.950374756619249084 ) ) ;
#10107=CARTESIAN_POINT ( 'NONE',  ( -26.09010956794245217, 20.58815999907601935, -6.950374756619243755 ) ) ;
#10112=CARTESIAN_POINT ( 'NONE',  ( -24.20753774853730889, 35.34635416666666430, 13.97622843553633842 ) ) ;
#10115=CARTESIAN_POINT ( 'NONE',  ( -30.02300923189239512, 49.38281249999997868, 2.654126918244515359E-13 ) ) ;
#10118=CARTESIAN_POINT ( 'NONE',  ( 7.468012846824777284, 56.69309000092396644, 28.02196122052045268 ) ) ;
#10119=CARTESIAN_POINT ( 'NONE',  ( -24.22776226481240514, 64.28423583425730214, 13.94119854578937812 ) ) ;
#10121=CARTESIAN_POINT ( 'NONE',  ( -28.02196122052058413, 17.15065999907602290, -7.468012846824272799 ) ) ;
#10126=CARTESIAN_POINT ( 'NONE',  ( 26.00068869287367335, 65.13802083333334281, 15.01150461594596308 ) ) ;
#10141=CARTESIAN_POINT ( 'NONE',  ( -6.950374756619716266, 34.34934000092397355, -26.09010956794232428 ) ) ;
#10147=CARTESIAN_POINT ( 'NONE',  ( 7.543491769121922985, 46.94232666574269075, 28.00173670424535644 ) ) ;
#10152=CARTESIAN_POINT ( 'NONE',  ( -27.95245687107223986, 68.56993083240934084, 0.04044903255043252877 ) ) ;
#10155=CARTESIAN_POINT ( 'NONE',  ( 26.00068869287340334, 16.44010416666666430, -15.01150461594642316 ) ) ;
#10161=CARTESIAN_POINT ( 'NONE',  ( 26.00068869287367335, 44.51302083333331439, 15.01150461594596308 ) ) ;
#10162=CARTESIAN_POINT ( 'NONE',  ( 26.00068869287340334, 64.56510416666667140, -15.01150461594642316 ) ) ;
#10173=CARTESIAN_POINT ( 'NONE',  ( 15.01150461594643382, 13.86197916666666252, 26.00068869287340334 ) ) ;
#10179=CARTESIAN_POINT ( 'NONE',  ( -6.950374756619247307, 30.04128499907601224, 26.09010956794245217 ) ) ;
#10187=CARTESIAN_POINT ( 'NONE',  ( 19.09188309203694800, 48.09375000000000000, 19.09188309203660694 ) ) ;
#10192=CARTESIAN_POINT ( 'NONE',  ( -6.988114217768288228, 29.47395833333332860, -26.07999730980477437 ) ) ;
#10196=CARTESIAN_POINT ( 'NONE',  ( -7.468012846824771955, 24.03684000092397000, -28.02196122052045624 ) ) ;
#10197=CARTESIAN_POINT ( 'NONE',  ( 7.505752307973351023, 65.56770833333332860, 28.01184896238290278 ) ) ;
#10206=CARTESIAN_POINT ( 'NONE',  ( 6.950374756619721595, 46.38059000092397355, 26.09010956794232428 ) ) ;
#10210=CARTESIAN_POINT ( 'NONE',  ( 20.50609665440969565, 12.85937500000000000, -20.50609665441004736 ) ) ;
#10215=CARTESIAN_POINT ( 'NONE',  ( 15.01150461594596308, 40.21614583333332860, -26.00068869287367335 ) ) ;
#10221=CARTESIAN_POINT ( 'NONE',  ( 20.53372385742108008, 56.96836833240936215, 20.47846945139866648 ) ) ;
#10223=CARTESIAN_POINT ( 'NONE',  ( -20.50609665440969209, 66.14062500000000000, 20.50609665441005092 ) ) ;
#10228=CARTESIAN_POINT ( 'NONE',  ( 13.97622843553589966, 19.59114583333332149, -24.20753774853756113 ) ) ;
#10244=CARTESIAN_POINT ( 'NONE',  ( 7.025853678916403666, 10.57329833425730747, -26.06988505166735237 ) ) ;
#10248=CARTESIAN_POINT ( 'NONE',  ( 2.740863092043355209E-13, 41.64843750000000000, 30.02300923189239512 ) ) ;
#10258=CARTESIAN_POINT ( 'NONE',  ( -2.584737979205441561E-13, 12.42968749999999289, -30.02300923189239512 ) ) ;
#10260=CARTESIAN_POINT ( 'NONE',  ( 30.02300923189239867, 37.35156249999999289, -2.619432448724978208E-13 ) ) ;
#10266=CARTESIAN_POINT ( 'NONE',  ( 7.025853678916867295, 53.81732666574268364, 26.06988505166722803 ) ) ;
#10272=DIRECTION ( 'NONE',  ( -0.7071067811865526798, 0.000000000000000000, -0.7071067811865423547 ) ) ;
#10280=CARTESIAN_POINT ( 'NONE',  ( -0.04044903255042732459, 17.86680583240935860, -27.95245687107223986 ) ) ;
#10285=CARTESIAN_POINT ( 'NONE',  ( -19.09188309203660694, 42.07812499999999289, 19.09188309203694800 ) ) ;
#10289=CARTESIAN_POINT ( 'NONE',  ( -7.505752307972844761, 48.66666666666666430, 28.01184896238304134 ) ) ;
#10292=CARTESIAN_POINT ( 'NONE',  ( -2.584737979205441561E-13, 15.86718749999999645, -30.02300923189239512 ) ) ;
#10293=CARTESIAN_POINT ( 'NONE',  ( -26.02091320914849959, 16.15923583425731636, 14.97647472619947528 ) ) ;
#10312=CARTESIAN_POINT ( 'NONE',  ( -6.950374756619716266, 27.47434000092397000, -26.09010956794232428 ) ) ;
#10318=CARTESIAN_POINT ( 'NONE',  ( 7.543491769121922985, 50.37982666574269075, 28.00173670424535644 ) ) ;
#10324=CARTESIAN_POINT ( 'NONE',  ( 26.07999730980477437, 13.14583333333332860, -6.988114217768290004 ) ) ;
#10328=CARTESIAN_POINT ( 'NONE',  ( -28.01184896238290278, 21.73958333333332860, 7.505752307973363457 ) ) ;
#10334=CARTESIAN_POINT ( 'NONE',  ( -7.505752307973343918, 39.78645833333332860, -28.01184896238290989 ) ) ;
#10335=CARTESIAN_POINT ( 'NONE',  ( 7.505752307973351023, 58.69270833333332860, 28.01184896238290278 ) ) ;
#10344=CARTESIAN_POINT ( 'NONE',  ( -30.02300923189239867, 15.00781249999999645, 2.654126918244514854E-13 ) ) ;
#10348=CARTESIAN_POINT ( 'NONE',  ( 24.22776226481265383, 32.76263916574268364, 13.94119854578893580 ) ) ;
#10355=CARTESIAN_POINT ( 'NONE',  ( -19.09188309203694445, 60.12500000000000000, -19.09188309203661049 ) ) ;
#10359=CARTESIAN_POINT ( 'NONE',  ( -26.07999730980490583, 42.65104166666666430, -6.988114217767815717 ) ) ;
#10360=CARTESIAN_POINT ( 'NONE',  ( 20.53372385742072481, 24.60975666759063785, -20.47846945139902175 ) ) ;
#10361=CARTESIAN_POINT ( 'NONE',  ( 15.04653450569339945, 19.29909749907602290, 25.98046417659831775 ) ) ;
#10370=CARTESIAN_POINT ( 'NONE',  ( 13.94119854578937812, 39.36236083425731636, 24.22776226481240514 ) ) ;
#10374=CARTESIAN_POINT ( 'NONE',  ( 28.01184896238304134, 13.43229166666666607, 7.505752307972846538 ) ) ;
#10378=CARTESIAN_POINT ( 'NONE',  ( -15.01150461594642138, 46.51822916666666430, -26.00068869287340334 ) ) ;
#10383=CARTESIAN_POINT ( 'NONE',  ( 20.53372385742108008, 63.84336833240935505, 20.47846945139866648 ) ) ;
#10385=CARTESIAN_POINT ( 'NONE',  ( 28.01184896238290278, 64.70833333333334281, -7.505752307973347470 ) ) ;
#10388=CARTESIAN_POINT ( 'NONE',  ( 19.09188309203661049, 64.42187499999998579, -19.09188309203694445 ) ) ;
#10391=CARTESIAN_POINT ( 'NONE',  ( -13.97622843553588901, 31.62239583333332860, 24.20753774853756823 ) ) ;
#10397=CARTESIAN_POINT ( 'NONE',  ( -26.06988505166735237, 47.52642333425731636, -7.025853678916388567 ) ) ;
#10407=CARTESIAN_POINT ( 'NONE',  ( 0.04044903254993986036, 10.43006916759064495, -27.95245687107223986 ) ) ;
#10412=CARTESIAN_POINT ( 'NONE',  ( 2.740863092043355209E-13, 45.08593750000000711, 30.02300923189239512 ) ) ;
#10423=CARTESIAN_POINT ( 'NONE',  ( -20.47846945139866648, 37.20274333240935505, 20.53372385742108008 ) ) ;
#10425=CARTESIAN_POINT ( 'NONE',  ( -28.01184896238304134, 35.77604166666666430, -7.505752307972844761 ) ) ;
#10432=CARTESIAN_POINT ( 'NONE',  ( 24.22776226481265383, 49.95013916574269786, 13.94119854578893580 ) ) ;
#10437=CARTESIAN_POINT ( 'NONE',  ( -13.97622843553632777, 15.58072916666666430, -24.20753774853731599 ) ) ;
#10445=CARTESIAN_POINT ( 'NONE',  ( 26.06988505166722803, 18.58295166574268364, -7.025853678916862854 ) ) ;
#10450=CARTESIAN_POINT ( 'NONE',  ( 6.988114217767829928, 40.07291666666666430, -26.07999730980489872 ) ) ;
#10453=CARTESIAN_POINT ( 'NONE',  ( 28.01184896238304134, 47.80729166666666430, 7.505752307972846538 ) ) ;
#10455=CARTESIAN_POINT ( 'NONE',  ( 26.00068869287367335, 13.57552083333332682, 15.01150461594596308 ) ) ;
#10456=CARTESIAN_POINT ( 'NONE',  ( -25.98046417659859486, 16.73215250092398065, -15.04653450569291628 ) ) ;
#10463=CARTESIAN_POINT ( 'NONE',  ( -26.00068869287368756, 66.85677083333334281, -15.01150461594595775 ) ) ;
#10477=CARTESIAN_POINT ( 'NONE',  ( 0.04044903254993986036, 34.49256916759064495, -27.95245687107223986 ) ) ;
#10484=CARTESIAN_POINT ( 'NONE',  ( -20.53372385742107653, 44.93711833240935505, -20.47846945139867003 ) ) ;
#10487=SURFACE_SIDE_STYLE ('',( #5678 ) ) ;
#10488=CARTESIAN_POINT ( 'NONE',  ( 2.584737979205441561E-13, 21.02343749999999645, 27.95245687107222921 ) ) ;
#10491=CARTESIAN_POINT ( 'NONE',  ( -20.50609665441004736, 18.87499999999999645, -20.50609665440969565 ) ) ;
#10495=CARTESIAN_POINT ( 'NONE',  ( -28.00173670424549499, 44.08892333425729504, -7.543491769121417612 ) ) ;
#10497=CARTESIAN_POINT ( 'NONE',  ( 15.01150461594596308, 47.09114583333332860, -26.00068869287367335 ) ) ;
#10508=CARTESIAN_POINT ( 'NONE',  ( 2.740863092043355209E-13, 24.46093749999999645, 30.02300923189239867 ) ) ;
#10514=CARTESIAN_POINT ( 'NONE',  ( 27.95245687107223276, 32.47618083240936215, -0.04044903255042905932 ) ) ;
#10522=CARTESIAN_POINT ( 'NONE',  ( -27.95245687107222921, 59.69531250000000711, 2.498001805406602216E-13 ) ) ;
#10526=CARTESIAN_POINT ( 'NONE',  ( -6.988114217768288228, 36.34895833333333570, -26.07999730980477437 ) ) ;
#10527=CARTESIAN_POINT ( 'NONE',  ( 20.53372385742072481, 28.04725666759063429, -20.47846945139902175 ) ) ;
#10528=CARTESIAN_POINT ( 'NONE',  ( -25.98046417659831420, 20.15847249907602290, 15.04653450569339945 ) ) ;
#10532=CARTESIAN_POINT ( 'NONE',  ( 6.950374756619257965, 48.94753499907601935, -26.09010956794244507 ) ) ;
#10538=CARTESIAN_POINT ( 'NONE',  ( -14.01125832528285109, 39.93527750092397355, 24.18731323226248264 ) ) ;
#10542=CARTESIAN_POINT ( 'NONE',  ( 20.50609665440969565, 19.73437500000000000, -20.50609665441004736 ) ) ;
#10546=CARTESIAN_POINT ( 'NONE',  ( 26.00068869287367335, 47.95052083333331439, 15.01150461594596308 ) ) ;
#10550=CARTESIAN_POINT ( 'NONE',  ( 0.04044903255045854962, 64.27305583240934084, 30.02300923189239867 ) ) ;
#10555=CARTESIAN_POINT ( 'NONE',  ( -13.97622843553588901, 62.55989583333332149, 24.20753774853756823 ) ) ;
#10560=CARTESIAN_POINT ( 'NONE',  ( 2.584737979205441561E-13, 34.77343750000000000, 27.95245687107222921 ) ) ;
#10567=CARTESIAN_POINT ( 'NONE',  ( 6.950374756619721595, 56.69309000092396644, 26.09010956794232428 ) ) ;
#10579=CARTESIAN_POINT ( 'NONE',  ( -19.11951029504763611, 16.01600666759064140, 19.06425588902592239 ) ) ;
#10584=CARTESIAN_POINT ( 'NONE',  ( 26.00068869287367335, 41.07552083333331439, 15.01150461594596308 ) ) ;
#10588=CARTESIAN_POINT ( 'NONE',  ( -15.01150461594595775, 17.87239583333332149, 26.00068869287368756 ) ) ;
#10595=CARTESIAN_POINT ( 'NONE',  ( -20.53372385742107653, 34.62461833240934794, -20.47846945139867003 ) ) ;
#10597=CARTESIAN_POINT ( 'NONE',  ( -15.01150461594642316, 39.64322916666667140, -26.00068869287341045 ) ) ;
#10602=CARTESIAN_POINT ( 'NONE',  ( -26.09010956794245217, 65.27565999907601224, -6.950374756619243755 ) ) ;
#10616=CARTESIAN_POINT ( 'NONE',  ( 7.025853678916867295, 22.87982666574268720, 26.06988505166722803 ) ) ;
#10620=CARTESIAN_POINT ( 'NONE',  ( -24.20753774853756823, 46.23177083333331439, -13.97622843553588723 ) ) ;
#10626=CARTESIAN_POINT ( 'NONE',  ( -20.53372385742071771, 64.14100666759063074, 20.47846945139902530 ) ) ;
#10627=CARTESIAN_POINT ( 'NONE',  ( 28.00173670424549499, 14.87017333425730747, 7.543491769121417612 ) ) ;
#10633=CARTESIAN_POINT ( 'NONE',  ( -7.505752307972844761, 65.85416666666665719, 28.01184896238304134 ) ) ;
#10647=CARTESIAN_POINT ( 'NONE',  ( 26.09010956794232428, 31.77121500092397000, -6.950374756619718042 ) ) ;
#10654=CARTESIAN_POINT ( 'NONE',  ( -25.98046417659831420, 44.22097249907603356, 15.04653450569339945 ) ) ;
#10658=CARTESIAN_POINT ( 'NONE',  ( 13.97622843553633665, 17.29947916666666430, 24.20753774853730889 ) ) ;
#10661=CARTESIAN_POINT ( 'NONE',  ( 15.01150461594643204, 20.73697916666666075, 26.00068869287340334 ) ) ;
#10665=CARTESIAN_POINT ( 'NONE',  ( 15.04653450569292872, 45.09152750092398065, -25.98046417659857710 ) ) ;
#10667=CARTESIAN_POINT ( 'NONE',  ( 26.00068869287367335, 54.82552083333331439, 15.01150461594596308 ) ) ;
#10676=CARTESIAN_POINT ( 'NONE',  ( -20.50609665440969209, 21.45312499999999645, 20.50609665441005092 ) ) ;
#10681=CARTESIAN_POINT ( 'NONE',  ( 0.04044903255044120238, 36.77305583240936215, 27.95245687107223276 ) ) ;
#10688=CARTESIAN_POINT ( 'NONE',  ( -6.988114217767819270, 58.97916666666666430, 26.07999730980490583 ) ) ;
#10693=CARTESIAN_POINT ( 'NONE',  ( 24.20753774853731244, 43.94010416666665719, -13.97622843553633132 ) ) ;
#10694=CARTESIAN_POINT ( 'NONE',  ( -20.53372385742071771, 26.32850666759063785, 20.47846945139902530 ) ) ;
#10695=CARTESIAN_POINT ( 'NONE',  ( -28.00173670424535644, 20.30170166574269075, 7.543491769121936308 ) ) ;
#10699=CARTESIAN_POINT ( 'NONE',  ( -19.06425588902558133, 50.95274333240935505, 19.11951029504797006 ) ) ;
#10705=CARTESIAN_POINT ( 'NONE',  ( -13.94119854578936923, 44.51861083425730214, -24.22776226481241224 ) ) ;
#10710=CARTESIAN_POINT ( 'NONE',  ( -15.01150461594642138, 22.45572916666666430, -26.00068869287340334 ) ) ;
#10715=CARTESIAN_POINT ( 'NONE',  ( -28.01184896238304134, 52.96354166666666430, -7.505752307972844761 ) ) ;
#10721=CARTESIAN_POINT ( 'NONE',  ( -20.47846945139866648, 57.82774333240935505, 20.53372385742108008 ) ) ;
#10727=CARTESIAN_POINT ( 'NONE',  ( 26.07999730980490227, 58.11979166666665719, 6.988114217767821046 ) ) ;
#10730=CARTESIAN_POINT ( 'NONE',  ( 24.20753774853731244, 33.62760416666665719, -13.97622843553632599 ) ) ;
#10736=CARTESIAN_POINT ( 'NONE',  ( 14.01125832528286352, 55.40402750092397355, -24.18731323226246843 ) ) ;
#10749=CARTESIAN_POINT ( 'NONE',  ( -26.09010956794232428, 12.86496500092397710, 6.950374756619732253 ) ) ;
#10754=CARTESIAN_POINT ( 'NONE',  ( 26.00068869287367335, 44.51302083333331439, 15.01150461594596308 ) ) ;
#10758=CARTESIAN_POINT ( 'NONE',  ( -15.01150461594642138, 22.45572916666666430, -26.00068869287340334 ) ) ;
#10764=CARTESIAN_POINT ( 'NONE',  ( 7.468012846824281681, 35.19753499907601935, -28.02196122052058058 ) ) ;
#10767=CARTESIAN_POINT ( 'NONE',  ( -15.01150461594642316, 46.51822916666666430, -26.00068869287341045 ) ) ;
#10773=CARTESIAN_POINT ( 'NONE',  ( 19.11951029504797006, 63.84336833240935505, 19.06425588902558133 ) ) ;
#10779=CARTESIAN_POINT ( 'NONE',  ( -19.09188309203694445, 25.74999999999999645, -19.09188309203661049 ) ) ;
#10786=CARTESIAN_POINT ( 'NONE',  ( 19.11951029504797006, 15.71836833240935327, 19.06425588902558133 ) ) ;
#10791=CARTESIAN_POINT ( 'NONE',  ( -6.988114217768288228, 43.22395833333332860, -26.07999730980477437 ) ) ;
#10795=CARTESIAN_POINT ( 'NONE',  ( -26.00068869287368756, 15.29427083333332504, -15.01150461594595775 ) ) ;
#10796=CARTESIAN_POINT ( 'NONE',  ( -14.97647472619946285, 13.58111083425730925, -26.02091320914851025 ) ) ;
#10817=CARTESIAN_POINT ( 'NONE',  ( -24.22776226481240514, 26.47173583425730925, 13.94119854578937812 ) ) ;
#10824=CARTESIAN_POINT ( 'NONE',  ( 15.04653450569339945, 43.36159749907602645, 25.98046417659831775 ) ) ;
#10827=CARTESIAN_POINT ( 'NONE',  ( -26.07999730980477437, 14.86458333333333037, 6.988114217768305103 ) ) ;
#10830=CARTESIAN_POINT ( 'NONE',  ( -26.00068869287340334, 21.59635416666666785, 15.01150461594643382 ) ) ;
#10834=CARTESIAN_POINT ( 'NONE',  ( 20.47846945139902530, 39.21913166759063785, 20.53372385742071771 ) ) ;
#10837=CARTESIAN_POINT ( 'NONE',  ( -20.50609665441004736, 53.25000000000000000, -20.50609665440969565 ) ) ;
#10849=CARTESIAN_POINT ( 'NONE',  ( 26.00068869287341045, 23.31510416666666430, -15.01150461594642493 ) ) ;
#10854=CARTESIAN_POINT ( 'NONE',  ( 24.18731323226221974, 32.18972249907602645, -14.01125832528328985 ) ) ;
#10862=CARTESIAN_POINT ( 'NONE',  ( -24.20753774853756823, 63.41927083333333570, -13.97622843553588723 ) ) ;
#10866=CARTESIAN_POINT ( 'NONE',  ( 6.988114217767829928, 43.51041666666666430, -26.07999730980489872 ) ) ;
#10867=CARTESIAN_POINT ( 'NONE',  ( 15.04653450569292872, 31.34152750092398421, -25.98046417659857710 ) ) ;
#10868=CARTESIAN_POINT ( 'NONE',  ( -30.02300923189239867, 17.00743083240935860, 0.04044903255044988294 ) ) ;
#10872=CARTESIAN_POINT ( 'NONE',  ( 19.11951029504797006, 46.65586833240934794, 19.06425588902558133 ) ) ;
#10878=CARTESIAN_POINT ( 'NONE',  ( -19.11951029504763611, 46.95350666759064495, 19.06425588902592239 ) ) ;
#10882=CARTESIAN_POINT ( 'NONE',  ( -26.00068869287340334, 25.03385416666666785, 15.01150461594643382 ) ) ;
#10886=CARTESIAN_POINT ( 'NONE',  ( 7.505752307973351023, 44.94270833333332860, 28.01184896238290278 ) ) ;
#10893=CARTESIAN_POINT ( 'NONE',  ( -20.53372385742107653, 62.12461833240934794, -20.47846945139867003 ) ) ;
#10898=CARTESIAN_POINT ( 'NONE',  ( -6.988114217767819270, 58.97916666666666430, 26.07999730980490583 ) ) ;
#10901=CARTESIAN_POINT ( 'NONE',  ( -2.428612866367529427E-13, 33.05468750000000000, -27.95245687107222921 ) ) ;
#10907=CARTESIAN_POINT ( 'NONE',  ( -7.025853678916393008, 56.97954833425730925, 26.06988505166735592 ) ) ;
#10918=CARTESIAN_POINT ( 'NONE',  ( 26.09010956794232428, 21.45871500092397355, -6.950374756619718042 ) ) ;
#10923=CARTESIAN_POINT ( 'NONE',  ( -26.00068869287368756, 46.23177083333331439, -15.01150461594595775 ) ) ;
#10925=CARTESIAN_POINT ( 'NONE',  ( 20.50609665440969565, 19.73437500000000000, -20.50609665441004736 ) ) ;
#10931=CARTESIAN_POINT ( 'NONE',  ( -15.04653450569338524, 38.20534749907601935, -25.98046417659831775 ) ) ;
#10933=CARTESIAN_POINT ( 'NONE',  ( -30.02300923189239867, 49.38281249999999289, 2.654126918244514854E-13 ) ) ;
#10939=CARTESIAN_POINT ( 'NONE',  ( -24.22776226481266448, 58.54388916574269075, -13.94119854578892514 ) ) ;
#10946=CARTESIAN_POINT ( 'NONE',  ( -2.428612866367529427E-13, 26.17968750000000000, -27.95245687107223276 ) ) ;
#10953=CARTESIAN_POINT ( 'NONE',  ( 24.22776226481265383, 25.88763916574269075, 13.94119854578893580 ) ) ;
#10956=CARTESIAN_POINT ( 'NONE',  ( 19.09188309203694800, 44.65624999999999289, 19.09188309203660694 ) ) ;
#10960=CARTESIAN_POINT ( 'NONE',  ( 20.50609665441005092, 17.15624999999999645, 20.50609665440969209 ) ) ;
#10961=CARTESIAN_POINT ( 'NONE',  ( -14.97647472619946285, 10.14361083425730925, -26.02091320914851025 ) ) ;
#10972=FILL_AREA_STYLE ('',( #16135 ) ) ;
#10984=CARTESIAN_POINT ( 'NONE',  ( -0.04044903254992426173, 43.08631916759065916, 27.95245687107223276 ) ) ;
#10988=UNCERTAINTY_MEASURE_WITH_UNIT (LENGTH_MEASURE( 1.000000000000000082E-05 ), #15818, 'distance_accuracy_value', 'NONE');
#10993=CARTESIAN_POINT ( 'NONE',  ( 0.04044903255045854962, 53.96055583240936926, 30.02300923189239867 ) ) ;
#10998=CARTESIAN_POINT ( 'NONE',  ( 24.20753774853756113, 13.57552083333332682, 13.97622843553589789 ) ) ;
#11000=CARTESIAN_POINT ( 'NONE',  ( -26.00068869287368756, 18.73177083333332149, -15.01150461594595775 ) ) ;
#11003=VERTEX_POINT ( 'NONE', #21823 ) ;
#11004=CARTESIAN_POINT ( 'NONE',  ( 14.97647472619947351, 42.79986083425731636, 26.02091320914850314 ) ) ;
#11006=CARTESIAN_POINT ( 'NONE',  ( 26.00068869287367335, 47.95052083333331439, 15.01150461594596308 ) ) ;
#11016=CARTESIAN_POINT ( 'NONE',  ( 30.02300923189239867, 23.60156250000000000, -2.619432448724978208E-13 ) ) ;
#11028=CARTESIAN_POINT ( 'NONE',  ( 6.988114217767829928, 60.69791666666667140, -26.07999730980489872 ) ) ;
#11032=CARTESIAN_POINT ( 'NONE',  ( -26.07999730980477437, 42.36458333333332860, 6.988114217768305103 ) ) ;
#11033=CARTESIAN_POINT ( 'NONE',  ( 7.468012846824777284, 25.75559000092397710, 28.02196122052045268 ) ) ;
#11034=CARTESIAN_POINT ( 'NONE',  ( 30.02300923189239867, 18.72618083240936215, -0.04044903255044467877 ) ) ;
#11039=CARTESIAN_POINT ( 'NONE',  ( -6.950374756619247307, 47.22878499907602645, 26.09010956794245217 ) ) ;
#11049=CARTESIAN_POINT ( 'NONE',  ( 0.04044903254993986036, 55.11756916759064495, -27.95245687107223986 ) ) ;
#11054=CARTESIAN_POINT ( 'NONE',  ( -7.505752307972844761, 24.60416666666666430, 28.01184896238304134 ) ) ;
#11058=CARTESIAN_POINT ( 'NONE',  ( -20.50609665441004736, 46.37500000000000000, -20.50609665440969565 ) ) ;
#11064=CARTESIAN_POINT ( 'NONE',  ( -7.468012846824272799, 60.97878499907603356, 28.02196122052058413 ) ) ;
#11067=CARTESIAN_POINT ( 'NONE',  ( -26.07999730980477437, 59.55208333333332149, 6.988114217768305103 ) ) ;
#11070=CARTESIAN_POINT ( 'NONE',  ( 6.988114217768294445, 31.19270833333333215, 26.07999730980477437 ) ) ;
#11076=CARTESIAN_POINT ( 'NONE',  ( -19.11951029504763611, 60.70350666759063785, 19.06425588902592239 ) ) ;
#11087=CARTESIAN_POINT ( 'NONE',  ( -0.04044903254992426173, 25.89881916759064140, 27.95245687107223276 ) ) ;
#11094=CARTESIAN_POINT ( 'NONE',  ( -26.00068869287368756, 49.66927083333330728, -15.01150461594595775 ) ) ;
#11098=CARTESIAN_POINT ( 'NONE',  ( -15.01150461594595775, 24.74739583333332504, 26.00068869287368756 ) ) ;
#11104=CARTESIAN_POINT ( 'NONE',  ( 14.97647472619900455, 38.77826416574269075, -26.02091320914876960 ) ) ;
#11106=CARTESIAN_POINT ( 'NONE',  ( -2.584737979205442066E-13, 46.80468750000000000, -30.02300923189239867 ) ) ;
#11109=CARTESIAN_POINT ( 'NONE',  ( 7.025853678916867295, 64.12982666574268364, 26.06988505166722803 ) ) ;
#11117=CARTESIAN_POINT ( 'NONE',  ( -24.20753774853756823, 22.16927083333332860, -13.97622843553588723 ) ) ;
#11124=CARTESIAN_POINT ( 'NONE',  ( -19.06425588902558133, 30.32774333240935150, 19.11951029504797006 ) ) ;
#11127=CARTESIAN_POINT ( 'NONE',  ( 24.20753774853756113, 54.82552083333331439, 13.97622843553589789 ) ) ;
#11132=CARTESIAN_POINT ( 'NONE',  ( -2.584737979205441561E-13, 26.17968750000000000, -30.02300923189239512 ) ) ;
#11133=CARTESIAN_POINT ( 'NONE',  ( -7.468012846824771955, 24.03684000092397000, -28.02196122052045624 ) ) ;
#11153=CARTESIAN_POINT ( 'NONE',  ( -19.11951029504763611, 43.51600666759065206, 19.06425588902592239 ) ) ;
#11161=CARTESIAN_POINT ( 'NONE',  ( -20.53372385742107653, 55.24961833240936926, -20.47846945139867003 ) ) ;
#11165=CARTESIAN_POINT ( 'NONE',  ( -13.97622843553632421, 25.89322916666666430, -24.20753774853731599 ) ) ;
#11168=CARTESIAN_POINT ( 'NONE',  ( -28.01184896238290278, 28.61458333333333215, 7.505752307973363457 ) ) ;
#11171=CARTESIAN_POINT ( 'NONE',  ( -14.97647472619946285, 41.08111083425730214, -26.02091320914851025 ) ) ;
#11173=CARTESIAN_POINT ( 'NONE',  ( -28.01184896238304134, 49.52604166666666430, -7.505752307972844761 ) ) ;
#11174=CARTESIAN_POINT ( 'NONE',  ( -30.02300923189239512, 66.57031250000000000, 2.654126918244515359E-13 ) ) ;
#11193=CARTESIAN_POINT ( 'NONE',  ( 0.04044903254993986036, 13.86756916759064318, -27.95245687107223986 ) ) ;
#11198=CARTESIAN_POINT ( 'NONE',  ( -6.988114217768288228, 53.53645833333332860, -26.07999730980477437 ) ) ;
#11199=CARTESIAN_POINT ( 'NONE',  ( -0.04044903254990864921, 36.21131916759064495, 30.02300923189239867 ) ) ;
#11200=CARTESIAN_POINT ( 'NONE',  ( 25.98046417659831775, 32.18972249907602645, -15.04653450569338879 ) ) ;
#11204=CARTESIAN_POINT ( 'NONE',  ( 27.95245687107223276, 56.53868083240936215, -0.04044903255042905932 ) ) ;
#11210=CARTESIAN_POINT ( 'NONE',  ( 24.22776226481241224, 52.25298583425730925, -13.94119854578936923 ) ) ;
#11214=CARTESIAN_POINT ( 'NONE',  ( -15.01150461594642138, 25.89322916666666430, -26.00068869287340334 ) ) ;
#11218=CARTESIAN_POINT ( 'NONE',  ( -28.01184896238304134, 56.40104166666666430, -7.505752307972844761 ) ) ;
#11224=CARTESIAN_POINT ( 'NONE',  ( -24.22776226481266448, 17.29388916574268720, -13.94119854578892514 ) ) ;
#11231=CARTESIAN_POINT ( 'NONE',  ( 2.584737979205441561E-13, 41.64843750000000000, 27.95245687107222921 ) ) ;
#11237=CARTESIAN_POINT ( 'NONE',  ( -24.18731323226248264, 61.41965250092398776, -14.01125832528284931 ) ) ;
#11239=CARTESIAN_POINT ( 'NONE',  ( 15.01150461594596308, 53.96614583333333570, -26.00068869287367335 ) ) ;
#11251=CARTESIAN_POINT ( 'NONE',  ( -14.01125832528285109, 26.18527750092397710, 24.18731323226248264 ) ) ;
#11257=CARTESIAN_POINT ( 'NONE',  ( 26.00068869287340334, 54.25260416666666430, -15.01150461594642316 ) ) ;
#11261=CARTESIAN_POINT ( 'NONE',  ( -20.50609665441004736, 25.74999999999999645, -20.50609665440969565 ) ) ;
#11267=CARTESIAN_POINT ( 'NONE',  ( 20.53372385742108008, 43.21836833240935505, 20.47846945139866648 ) ) ;
#11269=CARTESIAN_POINT ( 'NONE',  ( 7.505752307972854531, 46.94791666666666430, -28.01184896238303423 ) ) ;
#11273=CARTESIAN_POINT ( 'NONE',  ( -24.22776226481266448, 61.98138916574268364, -13.94119854578892514 ) ) ;
#11279=CARTESIAN_POINT ( 'NONE',  ( 24.20753774853756113, 20.45052083333332860, 13.97622843553589789 ) ) ;
#11286=CARTESIAN_POINT ( 'NONE',  ( 24.18731323226221974, 28.75222249907602290, -14.01125832528328985 ) ) ;
#11290=CARTESIAN_POINT ( 'NONE',  ( 19.09188309203694800, 51.53124999999999289, 19.09188309203660694 ) ) ;
#11294=CARTESIAN_POINT ( 'NONE',  ( 28.01184896238290278, 26.89583333333332860, -7.505752307973347470 ) ) ;
#11295=CARTESIAN_POINT ( 'NONE',  ( -20.47846945139902175, 23.75038166759064140, -20.53372385742072481 ) ) ;
#11312=CARTESIAN_POINT ( 'NONE',  ( -19.11951029504763611, 40.07850666759064495, 19.06425588902592239 ) ) ;
#11321=CARTESIAN_POINT ( 'NONE',  ( -7.468012846824272799, 57.54128499907602645, 28.02196122052058413 ) ) ;
#11324=CARTESIAN_POINT ( 'NONE',  ( 13.97622843553589966, 26.46614583333332149, -24.20753774853756113 ) ) ;
#11328=CARTESIAN_POINT ( 'NONE',  ( -7.505752307972844761, 31.47916666666666075, 28.01184896238304134 ) ) ;
#11331=CARTESIAN_POINT ( 'NONE',  ( -26.02091320914849959, 47.09673583425730214, 14.97647472619947528 ) ) ;
#11333=AXIS2_PLACEMENT_3D ( 'NONE', #11491, #19898, #19231 ) ;
#11334=CARTESIAN_POINT ( 'NONE',  ( -30.02300923189239512, 56.25781249999997868, 2.654126918244515359E-13 ) ) ;
#11353=CARTESIAN_POINT ( 'NONE',  ( -14.01125832528285109, 15.87277750092397710, 24.18731323226248264 ) ) ;
#11359=CARTESIAN_POINT ( 'NONE',  ( 26.07999730980477437, 54.39583333333332860, -6.988114217768290004 ) ) ;
#11360=CARTESIAN_POINT ( 'NONE',  ( -26.02091320914849959, 43.65923583425730925, 14.97647472619947528 ) ) ;
#11363=CARTESIAN_POINT ( 'NONE',  ( -20.47846945139866648, 26.89024333240934439, 20.53372385742108008 ) ) ;
#11366=CARTESIAN_POINT ( 'NONE',  ( -6.950374756619247307, 57.54128499907602645, 26.09010956794245217 ) ) ;
#11372=CARTESIAN_POINT ( 'NONE',  ( 26.06988505166735592, 49.24517333425730925, 7.025853678916393896 ) ) ;
#11376=CARTESIAN_POINT ( 'NONE',  ( -7.505752307972844761, 21.16666666666666430, 28.01184896238304134 ) ) ;
#11381=CARTESIAN_POINT ( 'NONE',  ( -2.584737979205441561E-13, 57.11718750000000711, -30.02300923189239512 ) ) ;
#11386=CARTESIAN_POINT ( 'NONE',  ( -7.025853678916861966, 17.72357666574268720, -26.06988505166722803 ) ) ;
#11392=CARTESIAN_POINT ( 'NONE',  ( 24.20753774853756113, 37.63802083333331439, 13.97622843553589789 ) ) ;
#11398=CARTESIAN_POINT ( 'NONE',  ( 28.00173670424549499, 11.43267333425730925, 7.543491769121417612 ) ) ;
#11399=CARTESIAN_POINT ( 'NONE',  ( -15.01150461594642138, 49.95572916666665009, -26.00068869287340334 ) ) ;
#11411=CARTESIAN_POINT ( 'NONE',  ( 13.94119854578937812, 22.17486083425730925, 24.22776226481240514 ) ) ;
#11417=CARTESIAN_POINT ( 'NONE',  ( -2.584737979205441561E-13, 50.24218750000000711, -30.02300923189239512 ) ) ;
#11421=CARTESIAN_POINT ( 'NONE',  ( 15.01150461594643204, 27.61197916666666430, 26.00068869287340334 ) ) ;
#11426=CARTESIAN_POINT ( 'NONE',  ( 28.00173670424535644, 46.08295166574269075, -7.543491769121920321 ) ) ;
#11428=CARTESIAN_POINT ( 'NONE',  ( -20.50609665440969209, 52.39062499999999289, 20.50609665441005092 ) ) ;
#11431=CARTESIAN_POINT ( 'NONE',  ( 13.97622843553589966, 16.15364583333333215, -24.20753774853756113 ) ) ;
#11437=CARTESIAN_POINT ( 'NONE',  ( 26.07999730980490227, 20.30729166666666430, 6.988114217767821046 ) ) ;
#11445=CARTESIAN_POINT ( 'NONE',  ( 26.09010956794244507, 32.61940999907601224, 6.950374756619249084 ) ) ;
#11449=CARTESIAN_POINT ( 'NONE',  ( -6.988114217767819270, 52.10416666666666430, 26.07999730980490583 ) ) ;
#11456=CARTESIAN_POINT ( 'NONE',  ( 15.01150461594596308, 26.46614583333332149, -26.00068869287367335 ) ) ;
#11457=CARTESIAN_POINT ( 'NONE',  ( 20.53372385742072481, 21.17225666759064850, -20.47846945139902175 ) ) ;
#11467=CARTESIAN_POINT ( 'NONE',  ( 20.47846945139902530, 59.84413166759065206, 20.53372385742071771 ) ) ;
#11472=CARTESIAN_POINT ( 'NONE',  ( -14.01125832528328985, 41.64284749907602645, -24.18731323226223040 ) ) ;
#11478=CARTESIAN_POINT ( 'NONE',  ( -24.22776226481240514, 40.22173583425730925, 13.94119854578937812 ) ) ;
#11485=CARTESIAN_POINT ( 'NONE',  ( -26.02091320914878025, 51.66888916574269075, -14.97647472619899389 ) ) ;
#11488=CARTESIAN_POINT ( 'NONE',  ( -24.20753774853756823, 29.04427083333332504, -13.97622843553588723 ) ) ;
#11490=CARTESIAN_POINT ( 'NONE',  ( 20.50609665441005092, 34.34374999999999289, 20.50609665440969209 ) ) ;
#11491=CARTESIAN_POINT ( 'NONE',  ( -19.79898987322349768, 67.00000000000000000, -19.79898987322315307 ) ) ;
#11493=CARTESIAN_POINT ( 'NONE',  ( 28.02196122052045268, 45.52121500092397355, -7.468012846824774620 ) ) ;
#11495=CARTESIAN_POINT ( 'NONE',  ( -2.584737979205441561E-13, 57.11718750000000711, -30.02300923189239512 ) ) ;
#11514=CARTESIAN_POINT ( 'NONE',  ( 27.95245687107222921, 64.85156249999998579, -2.463307335887066074E-13 ) ) ;
#11519=CARTESIAN_POINT ( 'NONE',  ( -27.95245687107223276, 45.94531249999998579, 2.498001805406602216E-13 ) ) ;
#11520=CARTESIAN_POINT ( 'NONE',  ( 0.04044903254992426173, 41.36756916759064495, -30.02300923189239867 ) ) ;
#11521=CARTESIAN_POINT ( 'NONE',  ( -25.98046417659831420, 27.03347249907602290, 15.04653450569339945 ) ) ;
#11524=CARTESIAN_POINT ( 'NONE',  ( 7.025853678916867295, 53.81732666574268364, 26.06988505166722803 ) ) ;
#11533=CARTESIAN_POINT ( 'NONE',  ( 28.01184896238290278, 30.33333333333332860, -7.505752307973347470 ) ) ;
#11538=CARTESIAN_POINT ( 'NONE',  ( -26.00068869287340334, 55.97135416666665719, 15.01150461594643382 ) ) ;
#11546=CARTESIAN_POINT ( 'NONE',  ( -14.01125832528328985, 14.14284749907602290, -24.18731323226223040 ) ) ;
#11554=CARTESIAN_POINT ( 'NONE',  ( 19.09188309203694800, 41.21875000000000000, 19.09188309203660694 ) ) ;
#11560=CARTESIAN_POINT ( 'NONE',  ( -7.543491769121417612, 12.29204833425730925, 28.00173670424549499 ) ) ;
#11561=CARTESIAN_POINT ( 'NONE',  ( -7.505752307973343918, 53.53645833333332860, -28.01184896238290989 ) ) ;
#11575=CARTESIAN_POINT ( 'NONE',  ( 24.18731323226247554, 21.88840250092397710, 14.01125832528285997 ) ) ;
#11580=CARTESIAN_POINT ( 'NONE',  ( 20.50609665440969565, 47.23437499999999289, -20.50609665441004736 ) ) ;
#11584=CARTESIAN_POINT ( 'NONE',  ( -30.02300923189239512, 28.75781249999999645, 2.654126918244515359E-13 ) ) ;
#11590=CARTESIAN_POINT ( 'NONE',  ( 0.04044903255045854962, 40.21055583240935505, 30.02300923189239867 ) ) ;
#11593=CARTESIAN_POINT ( 'NONE',  ( -7.505752307972844761, 62.41666666666666430, 28.01184896238304134 ) ) ;
#11596=CARTESIAN_POINT ( 'NONE',  ( 6.988114217768294445, 17.44270833333333215, 26.07999730980477437 ) ) ;
#11602=CARTESIAN_POINT ( 'NONE',  ( 2.584737979205442066E-13, 27.89843749999999645, 27.95245687107223276 ) ) ;
#11608=CARTESIAN_POINT ( 'NONE',  ( 28.02196122052058413, 25.74440999907601935, 7.468012846824272799 ) ) ;
#11610=CARTESIAN_POINT ( 'NONE',  ( -27.95245687107223986, 30.75743083240935505, 0.04044903255043252877 ) ) ;
#11614=CARTESIAN_POINT ( 'NONE',  ( -27.95245687107222921, 52.82031249999997868, 2.498001805406602216E-13 ) ) ;
#11615=ORIENTED_EDGE ( 'NONE', *, *, #33703, .F. ) ;
#11619=CARTESIAN_POINT ( 'NONE',  ( -7.505752307973343918, 26.03645833333333215, -28.01184896238290989 ) ) ;
#11620=CARTESIAN_POINT ( 'NONE',  ( 28.00173670424549499, 21.74517333425730925, 7.543491769121417612 ) ) ;
#11628=CARTESIAN_POINT ( 'NONE',  ( 15.04653450569292872, 51.96652750092398065, -25.98046417659857710 ) ) ;
#11631=CARTESIAN_POINT ( 'NONE',  ( -7.505752307972844761, 24.60416666666666430, 28.01184896238304134 ) ) ;
#11636=CARTESIAN_POINT ( 'NONE',  ( -26.06988505166722803, 40.92670166574268364, 7.025853678916877953 ) ) ;
#11642=CARTESIAN_POINT ( 'NONE',  ( 19.06425588902592239, 42.65663166759063785, 19.11951029504763611 ) ) ;
#11650=CARTESIAN_POINT ( 'NONE',  ( 20.53372385742108008, 60.40586833240935505, 20.47846945139866648 ) ) ;
#11654=CARTESIAN_POINT ( 'NONE',  ( -24.20753774853730889, 25.03385416666666785, 13.97622843553633842 ) ) ;
#11658=CARTESIAN_POINT ( 'NONE',  ( -26.00068869287340334, 35.34635416666666430, 15.01150461594643382 ) ) ;
#11661=CARTESIAN_POINT ( 'NONE',  ( 20.47846945139902530, 49.53163166759063785, 20.53372385742071771 ) ) ;
#11663=CARTESIAN_POINT ( 'NONE',  ( -26.00068869287368756, 59.98177083333332149, -15.01150461594595775 ) ) ;
#11682=CARTESIAN_POINT ( 'NONE',  ( -24.22776226481240514, 12.72173583425731458, 13.94119854578937812 ) ) ;
#11687=CARTESIAN_POINT ( 'NONE',  ( -19.09188309203660694, 48.95312500000000000, 19.09188309203694800 ) ) ;
#11688=CARTESIAN_POINT ( 'NONE',  ( 14.97647472619947351, 35.92486083425730214, 26.02091320914850314 ) ) ;
#11689=CARTESIAN_POINT ( 'NONE',  ( 7.468012846824281681, 24.88503499907601935, -28.02196122052058058 ) ) ;
#11692=CARTESIAN_POINT ( 'NONE',  ( 27.95245687107223276, 53.10118083240936215, -0.04044903255042905932 ) ) ;
#11701=CARTESIAN_POINT ( 'NONE',  ( 20.50609665441005092, 30.90624999999999645, 20.50609665440969209 ) ) ;
#11706=CARTESIAN_POINT ( 'NONE',  ( 15.01150461594596308, 53.96614583333333570, -26.00068869287367335 ) ) ;
#11713=CARTESIAN_POINT ( 'NONE',  ( 19.06425588902558133, 14.85899333240935505, -19.11951029504797006 ) ) ;
#11721=CARTESIAN_POINT ( 'NONE',  ( -19.09188309203660694, 42.07812499999999289, 19.09188309203694800 ) ) ;
#11727=CARTESIAN_POINT ( 'NONE',  ( -27.95245687107223986, 64.57069416759065916, -0.04044903254993292840 ) ) ;
#11728=CARTESIAN_POINT ( 'NONE',  ( -7.505752307973343918, 50.09895833333332860, -28.01184896238290989 ) ) ;
#11741=CARTESIAN_POINT ( 'NONE',  ( -13.94119854578936923, 34.20611083425730925, -24.22776226481241224 ) ) ;
#11747=CARTESIAN_POINT ( 'NONE',  ( 2.740863092043355209E-13, 48.52343750000000000, 30.02300923189239512 ) ) ;
#11751=CARTESIAN_POINT ( 'NONE',  ( -20.50609665441004736, 32.62500000000000000, -20.50609665440969565 ) ) ;
#11756=CARTESIAN_POINT ( 'NONE',  ( -20.47846945139866648, 44.07774333240935505, 20.53372385742108008 ) ) ;
#11758=CARTESIAN_POINT ( 'NONE',  ( 28.01184896238304134, 58.11979166666665719, 7.505752307972846538 ) ) ;
#11762=CARTESIAN_POINT ( 'NONE',  ( -13.97622843553632421, 12.14322916666666430, -24.20753774853731599 ) ) ;
#11768=CARTESIAN_POINT ( 'NONE',  ( 26.07999730980490227, 34.05729166666666430, 6.988114217767821046 ) ) ;
#11776=CARTESIAN_POINT ( 'NONE',  ( 0.04044903255045854962, 29.89805583240935860, 30.02300923189239867 ) ) ;
#11778=CARTESIAN_POINT ( 'NONE',  ( 0.04044903255044120238, 36.77305583240936215, 27.95245687107223276 ) ) ;
#11782=CARTESIAN_POINT ( 'NONE',  ( -19.06425588902591173, 10.00038166759064140, -19.11951029504763611 ) ) ;
#11787=CARTESIAN_POINT ( 'NONE',  ( -30.02300923189239512, 25.32031250000000000, 2.654126918244515359E-13 ) ) ;
#11788=CARTESIAN_POINT ( 'NONE',  ( -28.02196122052045268, 26.61496500092397355, 7.468012846824790607 ) ) ;
#11799=CARTESIAN_POINT ( 'NONE',  ( 25.98046417659858420, 52.82590250092398065, 15.04653450569292872 ) ) ;
#11802=CARTESIAN_POINT ( 'NONE',  ( 2.740863092043355209E-13, 27.89843749999999645, 30.02300923189239867 ) ) ;
#11807=CARTESIAN_POINT ( 'NONE',  ( -26.09010956794245217, 41.21315999907602645, -6.950374756619243755 ) ) ;
#11815=CARTESIAN_POINT ( 'NONE',  ( 7.025853678916403666, 51.82329833425730925, -26.06988505166735237 ) ) ;
#11821=CARTESIAN_POINT ( 'NONE',  ( -25.98046417659831420, 64.84597249907602645, 15.04653450569339945 ) ) ;
#11825=CARTESIAN_POINT ( 'NONE',  ( -26.07999730980490583, 22.02604166666666430, -6.988114217767815717 ) ) ;
#11828=CARTESIAN_POINT ( 'NONE',  ( 15.01150461594596308, 43.65364583333332860, -26.00068869287367335 ) ) ;
#11831=CARTESIAN_POINT ( 'NONE',  ( -20.47846945139902175, 47.81288166759064495, -20.53372385742072481 ) ) ;
#11833=CARTESIAN_POINT ( 'NONE',  ( -20.50609665440969209, 59.26562500000000000, 20.50609665441005092 ) ) ;
#11851=CARTESIAN_POINT ( 'NONE',  ( 24.18731323226247554, 15.01340250092397888, 14.01125832528285997 ) ) ;
#11856=CARTESIAN_POINT ( 'NONE',  ( -13.97622843553588901, 52.24739583333332860, 24.20753774853756823 ) ) ;
#11857=CARTESIAN_POINT ( 'NONE',  ( -25.98046417659859486, 40.79465250092398065, -15.04653450569291628 ) ) ;
#11859=CARTESIAN_POINT ( 'NONE',  ( 28.00173670424535644, 25.45795166574268364, -7.543491769121920321 ) ) ;
#11862=CARTESIAN_POINT ( 'NONE',  ( -0.04044903255042732459, 52.24180583240936215, -27.95245687107223986 ) ) ;
#11874=CARTESIAN_POINT ( 'NONE',  ( -2.584737979205441561E-13, 36.49218750000000000, -30.02300923189239512 ) ) ;
#11878=CARTESIAN_POINT ( 'NONE',  ( 26.00068869287340334, 61.12760416666665719, -15.01150461594642316 ) ) ;
#11887=CARTESIAN_POINT ( 'NONE',  ( -6.950374756619247307, 19.72878499907601935, 26.09010956794245217 ) ) ;
#11896=CARTESIAN_POINT ( 'NONE',  ( 19.09188309203661049, 36.92187499999999289, -19.09188309203694445 ) ) ;
#11901=CARTESIAN_POINT ( 'NONE',  ( -14.97647472619946285, 13.58111083425730925, -26.02091320914851025 ) ) ;
#11902=CARTESIAN_POINT ( 'NONE',  ( 30.02300923189239512, 57.97656249999997868, -2.619432448724977703E-13 ) ) ;
#11912=CARTESIAN_POINT ( 'NONE',  ( 19.06425588902592239, 28.90663166759063785, 19.11951029504763611 ) ) ;
#11918=CARTESIAN_POINT ( 'NONE',  ( 28.01184896238304134, 61.55729166666666430, 7.505752307972846538 ) ) ;
#11922=CARTESIAN_POINT ( 'NONE',  ( 26.00068869287367335, 27.32552083333332860, 15.01150461594596308 ) ) ;
#11929=CARTESIAN_POINT ( 'NONE',  ( -14.97647472619899389, 47.37201416574269786, 26.02091320914878025 ) ) ;
#11931=CARTESIAN_POINT ( 'NONE',  ( 26.00068869287367690, 54.82552083333332149, 15.01150461594596486 ) ) ;
#11935=CARTESIAN_POINT ( 'NONE',  ( 24.20753774853756113, 13.57552083333332682, 13.97622843553589789 ) ) ;
#11945=CARTESIAN_POINT ( 'NONE',  ( 26.02091320914876960, 22.45013916574269075, 14.97647472619900455 ) ) ;
#11947=CARTESIAN_POINT ( 'NONE',  ( 24.18731323226221974, 39.06472249907601935, -14.01125832528328985 ) ) ;
#11950=CARTESIAN_POINT ( 'NONE',  ( 26.07999730980477437, 64.70833333333334281, -6.988114217768290004 ) ) ;
#11955=CARTESIAN_POINT ( 'NONE',  ( -28.01184896238304134, 28.90104166666666785, -7.505752307972844761 ) ) ;
#11956=CARTESIAN_POINT ( 'NONE',  ( 7.543491769121427382, 34.63579833425730925, -28.00173670424548433 ) ) ;
#11965=CARTESIAN_POINT ( 'NONE',  ( 28.02196122052045268, 55.83371500092398065, -7.468012846824774620 ) ) ;
#11968=CARTESIAN_POINT ( 'NONE',  ( 15.01150461594596486, 26.46614583333332504, -26.00068869287367690 ) ) ;
#11974=CARTESIAN_POINT ( 'NONE',  ( 24.22776226481265383, 43.07513916574269786, 13.94119854578893580 ) ) ;
#11981=CARTESIAN_POINT ( 'NONE',  ( 13.94119854578937812, 46.23736083425730925, 24.22776226481240514 ) ) ;
#11986=CARTESIAN_POINT ( 'NONE',  ( 30.02300923189239867, 63.41368083240934794, -0.04044903255044467877 ) ) ;
#11991=CARTESIAN_POINT ( 'NONE',  ( 19.09188309203694800, 34.34374999999999289, 19.09188309203660694 ) ) ;
#11994=CARTESIAN_POINT ( 'NONE',  ( 2.740863092043355209E-13, 38.21093750000000000, 30.02300923189239512 ) ) ;
#11997=CARTESIAN_POINT ( 'NONE',  ( 28.02196122052045268, 52.39621500092398065, -7.468012846824774620 ) ) ;
#11998=CARTESIAN_POINT ( 'NONE',  ( -26.09010956794232428, 50.67746500092398065, 6.950374756619732253 ) ) ;
#12000=CARTESIAN_POINT ( 'NONE',  ( 2.740863092043355209E-13, 65.71093749999997158, 30.02300923189239512 ) ) ;
#12020=CARTESIAN_POINT ( 'NONE',  ( -0.04044903254992426173, 22.46131916759064850, 27.95245687107223276 ) ) ;
#12025=CARTESIAN_POINT ( 'NONE',  ( 24.20753774853756113, 54.82552083333332149, 13.97622843553589789 ) ) ;
#12026=CARTESIAN_POINT ( 'NONE',  ( 20.53372385742072481, 45.23475666759063785, -20.47846945139902175 ) ) ;
#12027=CARTESIAN_POINT ( 'NONE',  ( 20.53372385742108008, 36.34336833240934794, 20.47846945139866648 ) ) ;
#12031=CARTESIAN_POINT ( 'NONE',  ( -26.09010956794245217, 68.71315999907601224, -6.950374756619243755 ) ) ;
#12038=CARTESIAN_POINT ( 'NONE',  ( -28.01184896238290278, 35.48958333333332860, 7.505752307973363457 ) ) ;
#12053=CARTESIAN_POINT ( 'NONE',  ( -0.04044903255042732459, 24.74180583240935505, -27.95245687107223986 ) ) ;
#12061=CARTESIAN_POINT ( 'NONE',  ( 6.988114217767829928, 50.38541666666666430, -26.07999730980489872 ) ) ;
#12066=CARTESIAN_POINT ( 'NONE',  ( 14.97647472619947351, 15.29986083425731280, 26.02091320914850314 ) ) ;
#12068=CARTESIAN_POINT ( 'NONE',  ( 20.50609665441005092, 61.84374999999998579, 20.50609665440969209 ) ) ;
#12079=CARTESIAN_POINT ( 'NONE',  ( -7.025853678916393008, 29.47954833425730570, 26.06988505166735592 ) ) ;
#12084=CARTESIAN_POINT ( 'NONE',  ( -28.01184896238304134, 63.27604166666667140, -7.505752307972844761 ) ) ;
#12088=CARTESIAN_POINT ( 'NONE',  ( 2.740863092043355209E-13, 38.21093750000000000, 30.02300923189239512 ) ) ;
#12093=CARTESIAN_POINT ( 'NONE',  ( 25.98046417659831775, 49.37722249907602645, -15.04653450569338879 ) ) ;
#12095=CARTESIAN_POINT ( 'NONE',  ( 26.00068869287341045, 57.69010416666666430, -15.01150461594642493 ) ) ;
#12100=CARTESIAN_POINT ( 'NONE',  ( -19.09188309203660694, 18.01562499999999645, 19.09188309203694800 ) ) ;
#12110=CARTESIAN_POINT ( 'NONE',  ( 15.04653450569339945, 26.17409749907601935, 25.98046417659831775 ) ) ;
#12112=CARTESIAN_POINT ( 'NONE',  ( -19.11951029504797006, 34.62461833240934794, -19.06425588902558133 ) ) ;
#12116=CARTESIAN_POINT ( 'NONE',  ( -6.988114217767819270, 62.41666666666666430, 26.07999730980490583 ) ) ;
#12121=CARTESIAN_POINT ( 'NONE',  ( -28.01184896238290278, 32.05208333333332860, 7.505752307973363457 ) ) ;
#12122=CARTESIAN_POINT ( 'NONE',  ( 26.02091320914851025, 35.06548583425731636, -14.97647472619946463 ) ) ;
#12132=CARTESIAN_POINT ( 'NONE',  ( 28.00173670424549499, 52.68267333425730214, 7.543491769121417612 ) ) ;
#12135=CARTESIAN_POINT ( 'NONE',  ( 7.505752307973351023, 27.75520833333332860, 28.01184896238290278 ) ) ;
#12140=CARTESIAN_POINT ( 'NONE',  ( 26.06988505166722803, 46.08295166574269075, -7.025853678916862854 ) ) ;
#12147=CARTESIAN_POINT ( 'NONE',  ( 26.09010956794232428, 52.39621500092398065, -6.950374756619718042 ) ) ;
#12154=CARTESIAN_POINT ( 'NONE',  ( 26.02091320914876960, 63.70013916574268364, 14.97647472619900455 ) ) ;
#12160=CARTESIAN_POINT ( 'NONE',  ( 19.09188309203661049, 33.48437500000000000, -19.09188309203694445 ) ) ;
#12164=CARTESIAN_POINT ( 'NONE',  ( -28.01184896238304134, 35.77604166666666430, -7.505752307972844761 ) ) ;
#12167=CARTESIAN_POINT ( 'NONE',  ( -20.47846945139902175, 54.68788166759063785, -20.53372385742072481 ) ) ;
#12168=CARTESIAN_POINT ( 'NONE',  ( 19.11951029504763611, 58.98475666759065206, -19.06425588902591173 ) ) ;
#12171=CARTESIAN_POINT ( 'NONE',  ( 28.00173670424535644, 15.14545166574268897, -7.543491769121920321 ) ) ;
#12178=CARTESIAN_POINT ( 'NONE',  ( -19.09188309203694445, 67.00000000000000000, -19.09188309203661049 ) ) ;
#12192=CARTESIAN_POINT ( 'NONE',  ( 7.025853678916403666, 24.32329833425730214, -26.06988505166735237 ) ) ;
#12198=CARTESIAN_POINT ( 'NONE',  ( 20.53372385742072481, 48.67225666759065206, -20.47846945139902175 ) ) ;
#12199=CARTESIAN_POINT ( 'NONE',  ( -7.468012846824272799, 40.35378499907601935, 28.02196122052058413 ) ) ;
#12203=CARTESIAN_POINT ( 'NONE',  ( 26.09010956794244507, 63.55690999907603356, 6.950374756619249084 ) ) ;
#12206=CARTESIAN_POINT ( 'NONE',  ( 30.02300923189239512, 16.72656249999999645, -2.619432448724977703E-13 ) ) ;
#12213=CARTESIAN_POINT ( 'NONE',  ( -20.50609665440969209, 31.76562499999999289, 20.50609665441005092 ) ) ;
#12221=CARTESIAN_POINT ( 'NONE',  ( -7.505752307973343918, 15.72395833333332860, -28.01184896238290989 ) ) ;
#12226=CARTESIAN_POINT ( 'NONE',  ( 19.06425588902558133, 21.73399333240935505, -19.11951029504797006 ) ) ;
#12234=CARTESIAN_POINT ( 'NONE',  ( 13.97622843553589966, 47.09114583333332860, -24.20753774853756113 ) ) ;
#12239=CARTESIAN_POINT ( 'NONE',  ( 15.04653450569292872, 21.02902750092397710, -25.98046417659857710 ) ) ;
#12240=CARTESIAN_POINT ( 'NONE',  ( -2.584737979205441561E-13, 60.55468749999999289, -30.02300923189239512 ) ) ;
#12245=PRODUCT_DEFINITION ( 'UNKNOWN', '', #5506, #5835 ) ;
#12252=CARTESIAN_POINT ( 'NONE',  ( -0.04044903254992426173, 32.77381916759064495, 27.95245687107223276 ) ) ;
#12259=CARTESIAN_POINT ( 'NONE',  ( -28.01184896238304134, 39.21354166666666430, -7.505752307972844761 ) ) ;
#12264=CARTESIAN_POINT ( 'NONE',  ( -15.04653450569338524, 51.95534749907602645, -25.98046417659831775 ) ) ;
#12267=CARTESIAN_POINT ( 'NONE',  ( -15.01150461594642316, 56.83072916666665719, -26.00068869287341045 ) ) ;
#12273=CARTESIAN_POINT ( 'NONE',  ( 19.09188309203694800, 27.46875000000000000, 19.09188309203660694 ) ) ;
#12284=CARTESIAN_POINT ( 'NONE',  ( 20.47846945139867003, 28.60899333240935150, -20.53372385742107653 ) ) ;
#12286=CARTESIAN_POINT ( 'NONE',  ( -6.950374756619247307, 33.47878499907601935, 26.09010956794245217 ) ) ;
#12291=CARTESIAN_POINT ( 'NONE',  ( -26.07999730980477437, 66.42708333333332860, 6.988114217768305103 ) ) ;
#12297=CARTESIAN_POINT ( 'NONE',  ( 7.505752307973351023, 34.63020833333332860, 28.01184896238290278 ) ) ;
#12298=CARTESIAN_POINT ( 'NONE',  ( 7.468012846824777284, 32.63059000092395934, 28.02196122052045268 ) ) ;
#12309=CARTESIAN_POINT ( 'NONE',  ( 15.01150461594596308, 12.71614583333333037, -26.00068869287367335 ) ) ;
#12312=CARTESIAN_POINT ( 'NONE',  ( 15.01150461594643382, 27.61197916666666430, 26.00068869287340334 ) ) ;
#12319=CARTESIAN_POINT ( 'NONE',  ( -27.95245687107223986, 54.81993083240935505, 0.04044903255043252877 ) ) ;
#12326=CARTESIAN_POINT ( 'NONE',  ( -27.95245687107223986, 47.38319416759065206, -0.04044903254993292840 ) ) ;
#12333=CARTESIAN_POINT ( 'NONE',  ( 28.02196122052058413, 66.99440999907601224, 7.468012846824272799 ) ) ;
#12337=CARTESIAN_POINT ( 'NONE',  ( -6.988114217768288228, 36.34895833333333570, -26.07999730980477437 ) ) ;
#12340=CARTESIAN_POINT ( 'NONE',  ( 28.01184896238304134, 40.93229166666666430, 7.505752307972846538 ) ) ;
#12344=CARTESIAN_POINT ( 'NONE',  ( -26.02091320914849959, 57.40923583425731636, 14.97647472619947528 ) ) ;
#12345=CARTESIAN_POINT ( 'NONE',  ( 14.01125832528286352, 58.84152750092397355, -24.18731323226246843 ) ) ;
#12347=CARTESIAN_POINT ( 'NONE',  ( 28.00173670424535644, 18.58295166574268364, -7.543491769121920321 ) ) ;
#12367=CARTESIAN_POINT ( 'NONE',  ( -19.06425588902591173, 16.87538166759064140, -19.11951029504763611 ) ) ;
#12372=CARTESIAN_POINT ( 'NONE',  ( -25.98046417659859486, 51.10715250092397355, -15.04653450569291628 ) ) ;
#12374=CARTESIAN_POINT ( 'NONE',  ( 28.00173670424535644, 35.77045166574266943, -7.543491769121920321 ) ) ;
#12378=CARTESIAN_POINT ( 'NONE',  ( -19.11951029504797006, 62.12461833240934794, -19.06425588902558133 ) ) ;
#12382=CARTESIAN_POINT ( 'NONE',  ( -7.505752307973343918, 15.72395833333332860, -28.01184896238290989 ) ) ;
#12388=CARTESIAN_POINT ( 'NONE',  ( 15.01150461594596308, 40.21614583333332860, -26.00068869287367335 ) ) ;
#12396=CARTESIAN_POINT ( 'NONE',  ( -2.584737979205442066E-13, 15.86718749999999822, -30.02300923189239867 ) ) ;
#12402=CARTESIAN_POINT ( 'NONE',  ( -24.22776226481266448, 24.16888916574269075, -13.94119854578892514 ) ) ;
#12411=CARTESIAN_POINT ( 'NONE',  ( -13.97622843553632421, 49.95572916666665009, -24.20753774853731599 ) ) ;
#12415=CARTESIAN_POINT ( 'NONE',  ( 24.20753774853756113, 30.76302083333332860, 13.97622843553589789 ) ) ;
#12417=CARTESIAN_POINT ( 'NONE',  ( -25.98046417659859486, 23.60715250092398421, -15.04653450569291628 ) ) ;
#12418=CARTESIAN_POINT ( 'NONE',  ( -15.01150461594595775, 59.12239583333333570, 26.00068869287368756 ) ) ;
#12429=CARTESIAN_POINT ( 'NONE',  ( -26.06988505166735237, 30.33892333425730925, -7.025853678916388567 ) ) ;
#12434=CARTESIAN_POINT ( 'NONE',  ( -28.01184896238304134, 15.15104166666666252, -7.505752307972844761 ) ) ;
#12438=CARTESIAN_POINT ( 'NONE',  ( -26.00068869287368756, 35.91927083333332860, -15.01150461594595775 ) ) ;
#12444=CARTESIAN_POINT ( 'NONE',  ( -28.02196122052058413, 51.52565999907602645, -7.468012846824272799 ) ) ;
#12451=CARTESIAN_POINT ( 'NONE',  ( 24.20753774853731244, 19.87760416666666430, -13.97622843553632599 ) ) ;
#12463=CARTESIAN_POINT ( 'NONE',  ( -26.09010956794245217, 37.77565999907600514, -6.950374756619243755 ) ) ;
#12467=CARTESIAN_POINT ( 'NONE',  ( -24.20753774853730889, 62.84635416666667851, 13.97622843553633842 ) ) ;
#12472=CARTESIAN_POINT ( 'NONE',  ( -20.50609665441004736, 36.06250000000000000, -20.50609665440969565 ) ) ;
#12473=CARTESIAN_POINT ( 'NONE',  ( -20.47846945139902175, 30.62538166759064495, -20.53372385742072481 ) ) ;
#12484=CARTESIAN_POINT ( 'NONE',  ( 7.505752307973351023, 14.00520833333333215, 28.01184896238290278 ) ) ;
#12487=CARTESIAN_POINT ( 'NONE',  ( 7.505752307972854531, 29.76041666666666430, -28.01184896238303423 ) ) ;
#12492=CARTESIAN_POINT ( 'NONE',  ( -14.01125832528328985, 48.51784749907601935, -24.18731323226223040 ) ) ;
#12498=CARTESIAN_POINT ( 'NONE',  ( -6.988114217767819270, 17.72916666666666430, 26.07999730980490583 ) ) ;
#12507=CARTESIAN_POINT ( 'NONE',  ( -7.543491769121917656, 65.84857666574268364, -28.00173670424536354 ) ) ;
#12511=CARTESIAN_POINT ( 'NONE',  ( 19.09188309203694800, 37.78124999999999289, 19.09188309203660694 ) ) ;
#12515=CARTESIAN_POINT ( 'NONE',  ( -30.02300923189239512, 35.63281249999998579, 2.654126918244515359E-13 ) ) ;
#12518=CARTESIAN_POINT ( 'NONE',  ( 0.04044903254992426173, 61.99256916759065206, -30.02300923189239867 ) ) ;
#12519=CARTESIAN_POINT ( 'NONE',  ( -19.06425588902591173, 58.12538166759063785, -19.11951029504763611 ) ) ;
#12521=CARTESIAN_POINT ( 'NONE',  ( -20.47846945139866648, 20.01524333240935505, 20.53372385742108008 ) ) ;
#12527=DIRECTION ( 'NONE',  ( 0.7071067811865526798, 0.000000000000000000, 0.7071067811865423547 ) ) ;
#12541=CARTESIAN_POINT ( 'NONE',  ( -0.04044903254992426173, 19.02381916759064495, 27.95245687107223276 ) ) ;
#12546=CARTESIAN_POINT ( 'NONE',  ( -20.47846945139902175, 47.81288166759064495, -20.53372385742072481 ) ) ;
#12548=CARTESIAN_POINT ( 'NONE',  ( 28.00173670424535644, 39.20795166574269075, -7.543491769121920321 ) ) ;
#12552=CARTESIAN_POINT ( 'NONE',  ( 6.950374756619257965, 66.13503499907601224, -26.09010956794244507 ) ) ;
#12561=CARTESIAN_POINT ( 'NONE',  ( 26.00068869287367335, 41.07552083333331439, 15.01150461594596308 ) ) ;
#12569=CARTESIAN_POINT ( 'NONE',  ( 26.00068869287367690, 13.57552083333333037, 15.01150461594596486 ) ) ;
#12574=CARTESIAN_POINT ( 'NONE',  ( 26.09010956794244507, 22.30690999907601579, 6.950374756619249084 ) ) ;
#12582=CARTESIAN_POINT ( 'NONE',  ( -24.20753774853730889, 52.53385416666666430, 13.97622843553633842 ) ) ;
#12586=CARTESIAN_POINT ( 'NONE',  ( -26.07999730980490583, 32.33854166666666430, -6.988114217767815717 ) ) ;
#12587=CARTESIAN_POINT ( 'NONE',  ( -25.98046417659859486, 16.73215250092398065, -15.04653450569291628 ) ) ;
#12588=CARTESIAN_POINT ( 'NONE',  ( 30.02300923189239512, 64.85156249999998579, -2.619432448724977703E-13 ) ) ;
#12594=CARTESIAN_POINT ( 'NONE',  ( -24.20753774853730889, 66.28385416666664298, 13.97622843553634020 ) ) ;
#12599=CARTESIAN_POINT ( 'NONE',  ( 14.01125832528286352, 45.09152750092398065, -24.18731323226246843 ) ) ;
#12604=CARTESIAN_POINT ( 'NONE',  ( 26.00068869287367335, 13.57552083333332682, 15.01150461594596308 ) ) ;
#12608=CARTESIAN_POINT ( 'NONE',  ( 26.00068869287340334, 40.50260416666666430, -15.01150461594642316 ) ) ;
#12613=CARTESIAN_POINT ( 'NONE',  ( 28.00173670424535644, 52.95795166574269075, -7.543491769121920321 ) ) ;
#12620=CARTESIAN_POINT ( 'NONE',  ( 24.20753774853731244, 23.31510416666666430, -13.97622843553632599 ) ) ;
#12635=CARTESIAN_POINT ( 'NONE',  ( -27.95245687107223986, 16.44569416759064140, -0.04044903254993292840 ) ) ;
#12639=CARTESIAN_POINT ( 'NONE',  ( -30.02300923189239512, 35.63281249999998579, 2.654126918244515359E-13 ) ) ;
#12650=CARTESIAN_POINT ( 'NONE',  ( -28.01184896238290278, 14.86458333333333037, 7.505752307973363457 ) ) ;
#12653=CARTESIAN_POINT ( 'NONE',  ( -28.01184896238304134, 39.21354166666666430, -7.505752307972844761 ) ) ;
#12659=CARTESIAN_POINT ( 'NONE',  ( -19.06425588902558133, 50.95274333240935505, 19.11951029504797006 ) ) ;
#12664=CARTESIAN_POINT ( 'NONE',  ( 6.988114217767829928, 12.57291666666666252, -26.07999730980489872 ) ) ;
#12673=CARTESIAN_POINT ( 'NONE',  ( 24.18731323226221974, 18.43972249907602290, -14.01125832528328985 ) ) ;
#12679=CARTESIAN_POINT ( 'NONE',  ( -26.07999730980477437, 35.48958333333332860, 6.988114217768305103 ) ) ;
#12683=CARTESIAN_POINT ( 'NONE',  ( 2.740863092043355209E-13, 45.08593750000000711, 30.02300923189239512 ) ) ;
#12687=CARTESIAN_POINT ( 'NONE',  ( -20.47846945139902175, 61.56288166759063074, -20.53372385742072481 ) ) ;
#12688=CARTESIAN_POINT ( 'NONE',  ( 26.09010956794232428, 62.70871500092398065, -6.950374756619718042 ) ) ;
#12690=CARTESIAN_POINT ( 'NONE',  ( 20.53372385742108008, 19.15586833240934794, 20.47846945139866648 ) ) ;
#12695=CARTESIAN_POINT ( 'NONE',  ( -20.50609665441004736, 63.56249999999999289, -20.50609665440969565 ) ) ;
#12710=CARTESIAN_POINT ( 'NONE',  ( -27.95245687107223986, 23.32069416759064140, -0.04044903254993292840 ) ) ;
#12715=CARTESIAN_POINT ( 'NONE',  ( -25.98046417659859486, 44.23215250092398065, -15.04653450569291628 ) ) ;
#12717=CARTESIAN_POINT ( 'NONE',  ( -7.543491769121917656, 41.78607666574268364, -28.00173670424536354 ) ) ;
#12721=CARTESIAN_POINT ( 'NONE',  ( -24.18731323226221974, 61.40847249907603356, 14.01125832528330406 ) ) ;
#12724=FACE_OUTER_BOUND ( 'NONE', #25806, .T. ) ;
#12731=CARTESIAN_POINT ( 'NONE',  ( -28.01184896238290278, 42.36458333333332860, 7.505752307973363457 ) ) ;
#12732=CARTESIAN_POINT ( 'NONE',  ( -26.00068869287368756, 59.98177083333332149, -15.01150461594595775 ) ) ;
#12748=CARTESIAN_POINT ( 'NONE',  ( 14.01125832528330051, 22.73659749907601935, 24.18731323226221974 ) ) ;
#12757=CARTESIAN_POINT ( 'NONE',  ( 27.95245687107222921, 54.53906249999998579, -2.463307335887066074E-13 ) ) ;
#12761=CARTESIAN_POINT ( 'NONE',  ( -13.97622843553588901, 31.62239583333333215, 24.20753774853756823 ) ) ;
#12762=CARTESIAN_POINT ( 'NONE',  ( 30.02300923189239867, 18.16444416759064140, 0.04044903254992252006 ) ) ;
#12763=CARTESIAN_POINT ( 'NONE',  ( -7.505752307972844761, 65.85416666666665719, 28.01184896238304134 ) ) ;
#12773=CARTESIAN_POINT ( 'NONE',  ( 19.11951029504763611, 41.79725666759063785, -19.06425588902591173 ) ) ;
#12778=CARTESIAN_POINT ( 'NONE',  ( -20.50609665441004736, 18.87499999999999645, -20.50609665440969565 ) ) ;
#12782=CARTESIAN_POINT ( 'NONE',  ( 7.505752307973351023, 38.06770833333332860, 28.01184896238290278 ) ) ;
#12787=CARTESIAN_POINT ( 'NONE',  ( 7.468012846824281681, 52.38503499907601224, -28.02196122052058058 ) ) ;
#12794=CARTESIAN_POINT ( 'NONE',  ( 26.07999730980490227, 23.74479166666666430, 6.988114217767821046 ) ) ;
#12811=CARTESIAN_POINT ( 'NONE',  ( 6.950374756619721595, 18.88059000092397355, 26.09010956794232428 ) ) ;
#12815=CARTESIAN_POINT ( 'NONE',  ( 28.01184896238304134, 44.36979166666666430, 7.505752307972846538 ) ) ;
#12828=CARTESIAN_POINT ( 'NONE',  ( -20.53372385742071771, 64.14100666759063074, 20.47846945139902530 ) ) ;
#12830=CARTESIAN_POINT ( 'NONE',  ( 28.01184896238304134, 40.93229166666666430, 7.505752307972846538 ) ) ;
#12836=CARTESIAN_POINT ( 'NONE',  ( 14.01125832528330051, 50.23659749907603356, 24.18731323226221974 ) ) ;
#12849=CARTESIAN_POINT ( 'NONE',  ( 19.11951029504797006, 19.15586833240934794, 19.06425588902558133 ) ) ;
#12853=CARTESIAN_POINT ( 'NONE',  ( 6.988114217768294445, 41.50520833333333570, 26.07999730980477437 ) ) ;
#12856=CARTESIAN_POINT ( 'NONE',  ( -2.584737979205441561E-13, 46.80468750000000000, -30.02300923189239512 ) ) ;
#12858=CARTESIAN_POINT ( 'NONE',  ( -2.584737979205441561E-13, 19.30468749999999645, -30.02300923189239512 ) ) ;
#12859=CARTESIAN_POINT ( 'NONE',  ( 7.468012846824777284, 15.44309000092397355, 28.02196122052045268 ) ) ;
#12861=CARTESIAN_POINT ( 'NONE',  ( -28.02196122052058413, 20.58815999907601935, -7.468012846824272799 ) ) ;
#12881=CARTESIAN_POINT ( 'NONE',  ( -19.11951029504763611, 33.20350666759063074, 19.06425588902592239 ) ) ;
#12887=CARTESIAN_POINT ( 'NONE',  ( 30.02300923189239867, 49.66368083240936215, -0.04044903255044467877 ) ) ;
#12892=CARTESIAN_POINT ( 'NONE',  ( -24.20753774853730889, 18.15885416666666075, 13.97622843553633842 ) ) ;
#12895=CARTESIAN_POINT ( 'NONE',  ( 15.01150461594596308, 23.02864583333332149, -26.00068869287367335 ) ) ;
#12901=CARTESIAN_POINT ( 'NONE',  ( -28.01184896238290278, 45.80208333333333570, 7.505752307973363457 ) ) ;
#12902=CARTESIAN_POINT ( 'NONE',  ( 26.00068869287340334, 57.69010416666667140, -15.01150461594642316 ) ) ;
#12916=CARTESIAN_POINT ( 'NONE',  ( -27.95245687107223986, 30.75743083240935505, 0.04044903255043252877 ) ) ;
#12924=CARTESIAN_POINT ( 'NONE',  ( -19.09188309203660694, 59.26562500000000000, 19.09188309203694800 ) ) ;
#12928=CARTESIAN_POINT ( 'NONE',  ( -2.428612866367529427E-13, 43.36718749999999289, -27.95245687107223276 ) ) ;
#12929=CARTESIAN_POINT ( 'NONE',  ( 30.02300923189239867, 25.03944416759064495, 0.04044903254992252006 ) ) ;
#12931=CARTESIAN_POINT ( 'NONE',  ( -7.468012846824272799, 19.72878499907601935, 28.02196122052058413 ) ) ;
#12942=CARTESIAN_POINT ( 'NONE',  ( 6.950374756619721595, 42.94309000092397355, 26.09010956794232428 ) ) ;
#12947=CARTESIAN_POINT ( 'NONE',  ( -7.505752307973343918, 19.16145833333332860, -28.01184896238290989 ) ) ;
#12952=CARTESIAN_POINT ( 'NONE',  ( 15.01150461594643204, 51.67447916666665719, 26.00068869287340334 ) ) ;
#12957=CARTESIAN_POINT ( 'NONE',  ( -15.04653450569338524, 62.26784749907602645, -25.98046417659831775 ) ) ;
#12962=CARTESIAN_POINT ( 'NONE',  ( 19.09188309203661049, 57.54687500000000000, -19.09188309203694445 ) ) ;
#12965=CARTESIAN_POINT ( 'NONE',  ( 24.20753774853731244, 26.75260416666666430, -13.97622843553632599 ) ) ;
#12971=CARTESIAN_POINT ( 'NONE',  ( 26.09010956794232428, 48.95871500092396644, -6.950374756619718042 ) ) ;
#12982=CARTESIAN_POINT ( 'NONE',  ( 0.04044903254993986036, 17.30506916759064140, -27.95245687107223986 ) ) ;
#12989=CARTESIAN_POINT ( 'NONE',  ( 26.00068869287340334, 43.94010416666665719, -15.01150461594642316 ) ) ;
#12999=CARTESIAN_POINT ( 'NONE',  ( -0.04044903255044120238, 31.61680583240936215, -30.02300923189239867 ) ) ;
#13001=CARTESIAN_POINT ( 'NONE',  ( 28.01184896238290278, 40.64583333333332860, -7.505752307973347470 ) ) ;
#13007=CARTESIAN_POINT ( 'NONE',  ( 13.94119854578893580, 55.96576416574269786, -24.22776226481265383 ) ) ;
#13013=CARTESIAN_POINT ( 'NONE',  ( 27.95245687107223276, 13.28906249999999467, -2.463307335887066074E-13 ) ) ;
#13021=CARTESIAN_POINT ( 'NONE',  ( -26.09010956794245217, 17.15065999907602290, -6.950374756619243755 ) ) ;
#13025=CARTESIAN_POINT ( 'NONE',  ( -2.428612866367529427E-13, 46.80468750000000000, -27.95245687107222921 ) ) ;
#13028=CARTESIAN_POINT ( 'NONE',  ( 7.505752307973351023, 48.38020833333332860, 28.01184896238290278 ) ) ;
#13031=CARTESIAN_POINT ( 'NONE',  ( -7.505752307972844761, 14.29166666666666430, 28.01184896238304134 ) ) ;
#13032=CARTESIAN_POINT ( 'NONE',  ( -30.02300923189239867, 13.00819416759064318, -0.04044903254991731589 ) ) ;
#13052=CARTESIAN_POINT ( 'NONE',  ( -19.06425588902591173, 34.06288166759063785, -19.11951029504763611 ) ) ;
#13058=CARTESIAN_POINT ( 'NONE',  ( -28.00173670424535644, 51.23920166574269786, 7.543491769121936308 ) ) ;
#13061=CARTESIAN_POINT ( 'NONE',  ( 13.97622843553633665, 20.73697916666666075, 24.20753774853730889 ) ) ;
#13064=CARTESIAN_POINT ( 'NONE',  ( -30.02300923189239512, 18.44531249999999645, 2.654126918244515359E-13 ) ) ;
#13068=CARTESIAN_POINT ( 'NONE',  ( -28.02196122052045268, 43.80246500092398776, 7.468012846824790607 ) ) ;
#13070=CARTESIAN_POINT ( 'NONE',  ( -30.02300923189239512, 42.50781249999997868, 2.654126918244515359E-13 ) ) ;
#13071=CARTESIAN_POINT ( 'NONE',  ( 20.50609665440969565, 57.54687500000000000, -20.50609665441004736 ) ) ;
#13082=CARTESIAN_POINT ( 'NONE',  ( -2.584737979205442066E-13, 19.30468749999999645, -30.02300923189239867 ) ) ;
#13087=CARTESIAN_POINT ( 'NONE',  ( 24.18731323226221974, 35.62722249907602645, -14.01125832528328985 ) ) ;
#13094=CARTESIAN_POINT ( 'NONE',  ( -24.20753774853730889, 59.40885416666666430, 13.97622843553633842 ) ) ;
#13099=CARTESIAN_POINT ( 'NONE',  ( 6.988114217768294445, 44.94270833333332860, 26.07999730980477437 ) ) ;
#13100=CARTESIAN_POINT ( 'NONE',  ( 7.543491769121427382, 31.19829833425730570, -28.00173670424548433 ) ) ;
#13101=CARTESIAN_POINT ( 'NONE',  ( -15.04653450569338524, 17.58034749907602290, -25.98046417659831775 ) ) ;
#13105=CARTESIAN_POINT ( 'NONE',  ( 26.09010956794244507, 42.93190999907601935, 6.950374756619249084 ) ) ;
#13111=CARTESIAN_POINT ( 'NONE',  ( -14.01125832528285109, 43.37277750092397355, 24.18731323226248264 ) ) ;
#13115=CARTESIAN_POINT ( 'NONE',  ( 20.50609665441005092, 17.15624999999999645, 20.50609665440969209 ) ) ;
#13119=CARTESIAN_POINT ( 'NONE',  ( 28.01184896238290278, 50.95833333333332860, -7.505752307973347470 ) ) ;
#13123=CARTESIAN_POINT ( 'NONE',  ( -28.02196122052058413, 61.83815999907601935, -7.468012846824272799 ) ) ;
#13125=CARTESIAN_POINT ( 'NONE',  ( -30.02300923189239867, 63.13281249999999289, 2.654126918244514854E-13 ) ) ;
#13128=CARTESIAN_POINT ( 'NONE',  ( 27.95245687107223276, 64.85156249999997158, -2.463307335887066074E-13 ) ) ;
#13131=CARTESIAN_POINT ( 'NONE',  ( -6.988114217768288228, 36.34895833333333570, -26.07999730980477437 ) ) ;
#13137=CARTESIAN_POINT ( 'NONE',  ( 19.06425588902592239, 56.40663166759065206, 19.11951029504763611 ) ) ;
#13149=CARTESIAN_POINT ( 'NONE',  ( 14.01125832528286352, 14.15402750092397532, -24.18731323226246843 ) ) ;
#13153=CARTESIAN_POINT ( 'NONE',  ( -28.01184896238304134, 42.65104166666666430, -7.505752307972844761 ) ) ;
#13157=CARTESIAN_POINT ( 'NONE',  ( 26.00068869287340334, 23.31510416666666430, -15.01150461594642316 ) ) ;
#13163=CARTESIAN_POINT ( 'NONE',  ( 14.97647472619900455, 31.90326416574268364, -26.02091320914876960 ) ) ;
#13165=CARTESIAN_POINT ( 'NONE',  ( -15.01150461594595775, 38.49739583333332860, 26.00068869287368756 ) ) ;
#13171=CARTESIAN_POINT ( 'NONE',  ( -19.06425588902558133, 57.82774333240935505, 19.11951029504797006 ) ) ;
#13185=CARTESIAN_POINT ( 'NONE',  ( 14.01125832528330051, 15.86159749907602112, 24.18731323226221974 ) ) ;
#13190=CARTESIAN_POINT ( 'NONE',  ( -6.988114217768288228, 46.66145833333332860, -26.07999730980477437 ) ) ;
#13194=CARTESIAN_POINT ( 'NONE',  ( 15.01150461594596308, 19.59114583333332149, -26.00068869287367335 ) ) ;
#13195=CARTESIAN_POINT ( 'NONE',  ( 26.02091320914851025, 14.44048583425730925, -14.97647472619946463 ) ) ;
#13214=CARTESIAN_POINT ( 'NONE',  ( 7.025853678916403666, 27.76079833425730925, -26.06988505166735237 ) ) ;
#13223=CARTESIAN_POINT ( 'NONE',  ( 7.468012846824281681, 48.94753499907601935, -28.02196122052058058 ) ) ;
#13227=CARTESIAN_POINT ( 'NONE',  ( -6.988114217767819270, 17.72916666666666430, 26.07999730980490583 ) ) ;
#13230=CARTESIAN_POINT ( 'NONE',  ( -20.50609665440969209, 24.89062500000000000, 20.50609665441005092 ) ) ;
#13235=CARTESIAN_POINT ( 'NONE',  ( 7.543491769121427382, 44.94829833425730925, -28.00173670424548433 ) ) ;
#13237=CARTESIAN_POINT ( 'NONE',  ( 20.50609665441005092, 48.09375000000000000, 20.50609665440969209 ) ) ;
#13249=CARTESIAN_POINT ( 'NONE',  ( -28.01184896238304134, 25.46354166666666430, -7.505752307972844761 ) ) ;
#13254=CARTESIAN_POINT ( 'NONE',  ( 26.09010956794244507, 32.61940999907601224, 6.950374756619249084 ) ) ;
#13261=CARTESIAN_POINT ( 'NONE',  ( 27.95245687107222921, 57.97656249999997868, -2.463307335887066074E-13 ) ) ;
#13266=CARTESIAN_POINT ( 'NONE',  ( 19.09188309203694800, 41.21875000000000000, 19.09188309203660694 ) ) ;
#13267=CARTESIAN_POINT ( 'NONE',  ( -30.02300923189239867, 33.63319416759063785, -0.04044903254991731589 ) ) ;
#13268=CARTESIAN_POINT ( 'NONE',  ( -20.53372385742107653, 17.43711833240935505, -20.47846945139867003 ) ) ;
#13272=CARTESIAN_POINT ( 'NONE',  ( -6.950374756619247307, 50.66628499907601935, 26.09010956794245217 ) ) ;
#13278=CARTESIAN_POINT ( 'NONE',  ( -27.95245687107223986, 43.94569416759065206, -0.04044903254993292840 ) ) ;
#13282=CARTESIAN_POINT ( 'NONE',  ( -28.01184896238304134, 28.90104166666666785, -7.505752307972844761 ) ) ;
#13287=CARTESIAN_POINT ( 'NONE',  ( 26.00068869287340334, 47.37760416666666430, -15.01150461594642316 ) ) ;
#13295=CARTESIAN_POINT ( 'NONE',  ( 15.04653450569339945, 60.54909749907603356, 25.98046417659831775 ) ) ;
#13300=CARTESIAN_POINT ( 'NONE',  ( 27.95245687107223276, 57.97656249999998579, -2.463307335887066074E-13 ) ) ;
#13303=CARTESIAN_POINT ( 'NONE',  ( 26.07999730980490227, 30.61979166666666075, 6.988114217767821046 ) ) ;
#13310=CARTESIAN_POINT ( 'NONE',  ( 26.06988505166735592, 59.55767333425731636, 7.025853678916393896 ) ) ;
#13323=CARTESIAN_POINT ( 'NONE',  ( -14.01125832528285109, 12.43527750092397532, 24.18731323226248264 ) ) ;
#13328=CARTESIAN_POINT ( 'NONE',  ( 7.505752307972854531, 46.94791666666666430, -28.01184896238303423 ) ) ;
#13332=CARTESIAN_POINT ( 'NONE',  ( 2.740863092043355209E-13, 24.46093749999999645, 30.02300923189239512 ) ) ;
#13339=CARTESIAN_POINT ( 'NONE',  ( -30.02300923189239867, 30.75743083240935505, 0.04044903255044988294 ) ) ;
#13341=CARTESIAN_POINT ( 'NONE',  ( 30.02300923189239867, 44.22656249999999289, -2.619432448724978208E-13 ) ) ;
#13346=CARTESIAN_POINT ( 'NONE',  ( -26.06988505166722803, 58.11420166574269075, 7.025853678916877953 ) ) ;
#13352=CARTESIAN_POINT ( 'NONE',  ( -27.95245687107223276, 25.32031250000000000, 2.498001805406602216E-13 ) ) ;
#13360=CARTESIAN_POINT ( 'NONE',  ( 14.01125832528330051, 22.73659749907601935, 24.18731323226221974 ) ) ;
#13364=CARTESIAN_POINT ( 'NONE',  ( 26.07999730980490227, 47.80729166666666430, 6.988114217767821046 ) ) ;
#13371=CARTESIAN_POINT ( 'NONE',  ( -26.00068869287340334, 14.72135416666666607, 15.01150461594643382 ) ) ;
#13372=CARTESIAN_POINT ( 'NONE',  ( 20.53372385742072481, 17.73475666759064140, -20.47846945139902175 ) ) ;
#13392=CARTESIAN_POINT ( 'NONE',  ( -26.06988505166735237, 30.33892333425730925, -7.025853678916388567 ) ) ;
#13401=CARTESIAN_POINT ( 'NONE',  ( -25.98046417659831420, 47.65847249907603356, 15.04653450569339945 ) ) ;
#13405=CARTESIAN_POINT ( 'NONE',  ( 13.97622843553589966, 12.71614583333333037, -24.20753774853756113 ) ) ;
#13407=CARTESIAN_POINT ( 'NONE',  ( 26.00068869287367335, 20.45052083333332504, 15.01150461594596308 ) ) ;
#13412=CARTESIAN_POINT ( 'NONE',  ( -7.543491769121417612, 36.35454833425730925, 28.00173670424549499 ) ) ;
#13414=CARTESIAN_POINT ( 'NONE',  ( -28.01184896238290278, 52.67708333333333570, 7.505752307973363457 ) ) ;
#13424=CARTESIAN_POINT ( 'NONE',  ( -7.505752307973343918, 22.59895833333332860, -28.01184896238290989 ) ) ;
#13429=CARTESIAN_POINT ( 'NONE',  ( -27.95245687107223986, 34.19493083240935505, 0.04044903255043252877 ) ) ;
#13438=CARTESIAN_POINT ( 'NONE',  ( -24.20753774853756823, 56.54427083333332149, -13.97622843553588723 ) ) ;
#13442=CARTESIAN_POINT ( 'NONE',  ( 2.584737979205442066E-13, 41.64843749999999289, 27.95245687107223276 ) ) ;
#13443=CARTESIAN_POINT ( 'NONE',  ( -28.00173670424549499, 30.33892333425730925, -7.543491769121417612 ) ) ;
#13444=CARTESIAN_POINT ( 'NONE',  ( -14.97647472619899389, 16.43451416574268720, 26.02091320914878025 ) ) ;
#13448=CARTESIAN_POINT ( 'NONE',  ( 27.95245687107223276, 46.22618083240936215, -0.04044903255042905932 ) ) ;
#13455=CARTESIAN_POINT ( 'NONE',  ( 6.950374756619721595, 49.81809000092397355, 26.09010956794232428 ) ) ;
#13459=CARTESIAN_POINT ( 'NONE',  ( 30.02300923189239512, 27.03906250000000000, -2.619432448724977703E-13 ) ) ;
#13460=AXIS2_PLACEMENT_3D ( 'NONE', #5605, #18151, #5435 ) ;
#13465=CARTESIAN_POINT ( 'NONE',  ( -2.584737979205441561E-13, 46.80468750000000000, -30.02300923189239512 ) ) ;
#13473=CARTESIAN_POINT ( 'NONE',  ( 7.468012846824281681, 59.26003499907601935, -28.02196122052058058 ) ) ;
#13478=CARTESIAN_POINT ( 'NONE',  ( 13.97622843553633842, 61.98697916666665719, 24.20753774853730889 ) ) ;
#13481=CARTESIAN_POINT ( 'NONE',  ( -27.95245687107222921, 28.75781249999999645, 2.498001805406602216E-13 ) ) ;
#13486=CARTESIAN_POINT ( 'NONE',  ( -19.06425588902591173, 54.68788166759063785, -19.11951029504763611 ) ) ;
#13498=CARTESIAN_POINT ( 'NONE',  ( 14.01125832528286352, 24.46652750092397355, -24.18731323226246843 ) ) ;
#13505=CARTESIAN_POINT ( 'NONE',  ( -26.00068869287340334, 45.65885416666666430, 15.01150461594643382 ) ) ;
#13509=CARTESIAN_POINT ( 'NONE',  ( -28.01184896238290278, 18.30208333333332860, 7.505752307973363457 ) ) ;
#13515=CARTESIAN_POINT ( 'NONE',  ( 28.00173670424535644, 35.77045166574266943, -7.543491769121920321 ) ) ;
#13517=CARTESIAN_POINT ( 'NONE',  ( -26.00068869287340334, 52.53385416666666430, 15.01150461594643559 ) ) ;
#13522=CARTESIAN_POINT ( 'NONE',  ( 19.06425588902558133, 62.98399333240935505, -19.11951029504797006 ) ) ;
#13528=CARTESIAN_POINT ( 'NONE',  ( -27.95245687107223276, 18.44531249999999645, 2.498001805406602216E-13 ) ) ;
#13536=CARTESIAN_POINT ( 'NONE',  ( 19.06425588902558133, 25.17149333240934439, -19.11951029504797006 ) ) ;
#13539=CARTESIAN_POINT ( 'NONE',  ( 2.584737979205441561E-13, 48.52343750000000000, 27.95245687107222921 ) ) ;
#13543=CARTESIAN_POINT ( 'NONE',  ( 30.02300923189239512, 13.28906249999999289, -2.619432448724977703E-13 ) ) ;
#13544=CARTESIAN_POINT ( 'NONE',  ( 15.04653450569292872, 10.71652750092397888, -25.98046417659857710 ) ) ;
#13568=CARTESIAN_POINT ( 'NONE',  ( 14.01125832528286352, 31.34152750092398421, -24.18731323226246843 ) ) ;
#13576=CARTESIAN_POINT ( 'NONE',  ( -15.04653450569338524, 45.08034749907603356, -25.98046417659831775 ) ) ;
#13580=CARTESIAN_POINT ( 'NONE',  ( 6.988114217768294445, 17.44270833333333215, 26.07999730980477437 ) ) ;
#13583=CARTESIAN_POINT ( 'NONE',  ( 20.50609665441005092, 24.03124999999999645, 20.50609665440969209 ) ) ;
#13585=ORIENTED_EDGE ( 'NONE', *, *, #1215, .F. ) ;
#13586=CARTESIAN_POINT ( 'NONE',  ( 14.97647472619947351, 39.36236083425731636, 26.02091320914850314 ) ) ;
#13588=CARTESIAN_POINT ( 'NONE',  ( 26.00068869287340334, 50.81510416666667140, -15.01150461594642316 ) ) ;
#13597=CARTESIAN_POINT ( 'NONE',  ( 26.00068869287341045, 19.87760416666666430, -15.01150461594642493 ) ) ;
#13610=CARTESIAN_POINT ( 'NONE',  ( -19.09188309203660694, 55.82812499999999289, 19.09188309203694800 ) ) ;
#13614=CARTESIAN_POINT ( 'NONE',  ( -2.428612866367529427E-13, 36.49218749999999289, -27.95245687107223276 ) ) ;
#13615=CARTESIAN_POINT ( 'NONE',  ( -0.04044903254990864921, 29.33631916759064850, 30.02300923189239867 ) ) ;
#13616=CARTESIAN_POINT ( 'NONE',  ( 20.53372385742108008, 15.71836833240935327, 20.47846945139866648 ) ) ;
#13620=CARTESIAN_POINT ( 'NONE',  ( 27.95245687107223276, 49.66368083240936215, -0.04044903255042905932 ) ) ;
#13627=CARTESIAN_POINT ( 'NONE',  ( -19.06425588902591173, 54.68788166759063785, -19.11951029504763611 ) ) ;
#13631=CARTESIAN_POINT ( 'NONE',  ( -30.02300923189239512, 21.88281249999999645, 2.654126918244515359E-13 ) ) ;
#13635=CARTESIAN_POINT ( 'NONE',  ( -30.02300923189239512, 49.38281249999997868, 2.654126918244515359E-13 ) ) ;
#13641=CARTESIAN_POINT ( 'NONE',  ( 28.02196122052058413, 63.55690999907603356, 7.468012846824272799 ) ) ;
#13645=CARTESIAN_POINT ( 'NONE',  ( -27.95245687107223276, 63.13281249999999289, 2.498001805406602216E-13 ) ) ;
#13648=CARTESIAN_POINT ( 'NONE',  ( 19.09188309203694800, 30.90624999999999645, 19.09188309203660694 ) ) ;
#13653=CARTESIAN_POINT ( 'NONE',  ( 13.94119854578937812, 59.98736083425730925, 24.22776226481240514 ) ) ;
#13666=CARTESIAN_POINT ( 'NONE',  ( -13.94119854578936923, 20.45611083425730925, -24.22776226481241224 ) ) ;
#13671=CARTESIAN_POINT ( 'NONE',  ( -26.00068869287340334, 55.97135416666665719, 15.01150461594643382 ) ) ;
#13675=CARTESIAN_POINT ( 'NONE',  ( 20.50609665441005092, 20.59374999999999645, 20.50609665440969209 ) ) ;
#13681=CARTESIAN_POINT ( 'NONE',  ( 25.98046417659831775, 32.18972249907602645, -15.04653450569338879 ) ) ;
#13683=CARTESIAN_POINT ( 'NONE',  ( -7.505752307972844761, 52.10416666666666430, 28.01184896238304134 ) ) ;
#13686=CARTESIAN_POINT ( 'NONE',  ( -19.06425588902558133, 61.26524333240935505, 19.11951029504797006 ) ) ;
#13692=CARTESIAN_POINT ( 'NONE',  ( -24.20753774853756823, 25.60677083333332860, -13.97622843553588723 ) ) ;
#13700=CARTESIAN_POINT ( 'NONE',  ( -24.18731323226221974, 27.03347249907602290, 14.01125832528330406 ) ) ;
#13702=CARTESIAN_POINT ( 'NONE',  ( -13.97622843553632421, 53.39322916666665009, -24.20753774853731599 ) ) ;
#13706=CARTESIAN_POINT ( 'NONE',  ( -15.01150461594595775, 28.18489583333332860, 26.00068869287368756 ) ) ;
#13707=CARTESIAN_POINT ( 'NONE',  ( -28.00173670424549499, 23.46392333425730570, -7.543491769121417612 ) ) ;
#13728=CARTESIAN_POINT ( 'NONE',  ( -7.025853678916393008, 43.22954833425730925, 26.06988505166735592 ) ) ;
#13734=CARTESIAN_POINT ( 'NONE',  ( -25.98046417659831420, 57.97097249907601935, 15.04653450569339945 ) ) ;
#13737=CARTESIAN_POINT ( 'NONE',  ( 19.09188309203661049, 23.17187499999999289, -19.09188309203694445 ) ) ;
#13740=CARTESIAN_POINT ( 'NONE',  ( -7.505752307972844761, 34.91666666666666430, 28.01184896238304134 ) ) ;
#13743=CARTESIAN_POINT ( 'NONE',  ( 0.04044903254992426173, 41.36756916759064495, -30.02300923189239867 ) ) ;
#13745=CARTESIAN_POINT ( 'NONE',  ( -7.505752307972844761, 48.66666666666666430, 28.01184896238304134 ) ) ;
#13766=CARTESIAN_POINT ( 'NONE',  ( 6.988114217768294445, 65.56770833333332860, 26.07999730980477437 ) ) ;
#13771=CARTESIAN_POINT ( 'NONE',  ( -26.07999730980477437, 52.67708333333333570, 6.988114217768305103 ) ) ;
#13772=CARTESIAN_POINT ( 'NONE',  ( 26.02091320914851025, 28.19048583425731636, -14.97647472619946463 ) ) ;
#13773=CARTESIAN_POINT ( 'NONE',  ( 30.02300923189239867, 32.47618083240936215, -0.04044903255044467877 ) ) ;
#13779=CARTESIAN_POINT ( 'NONE',  ( -19.11951029504797006, 44.93711833240935505, -19.06425588902558133 ) ) ;
#13786=CARTESIAN_POINT ( 'NONE',  ( 26.06988505166735592, 52.68267333425730214, 7.025853678916393896 ) ) ;
#13791=CARTESIAN_POINT ( 'NONE',  ( 7.505752307972854531, 22.88541666666666430, -28.01184896238303423 ) ) ;
#13797=CARTESIAN_POINT ( 'NONE',  ( -26.00068869287368756, 59.98177083333332149, -15.01150461594595775 ) ) ;
#13803=CARTESIAN_POINT ( 'NONE',  ( 27.95245687107223276, 15.28868083240935505, -0.04044903255042905932 ) ) ;
#13810=CARTESIAN_POINT ( 'NONE',  ( 27.95245687107222921, 30.47656250000000355, -2.463307335887066074E-13 ) ) ;
#13817=CARTESIAN_POINT ( 'NONE',  ( 0.04044903254993986036, 58.55506916759063785, -27.95245687107223986 ) ) ;
#13829=CARTESIAN_POINT ( 'NONE',  ( 7.025853678916403666, 20.88579833425730925, -26.06988505166735237 ) ) ;
#13834=CARTESIAN_POINT ( 'NONE',  ( 26.00068869287367335, 47.95052083333331439, 15.01150461594596308 ) ) ;
#13838=CARTESIAN_POINT ( 'NONE',  ( 20.50609665441005092, 17.15624999999999645, 20.50609665440969209 ) ) ;
#13845=CARTESIAN_POINT ( 'NONE',  ( -25.98046417659831420, 47.65847249907603356, 15.04653450569339945 ) ) ;
#13847=CARTESIAN_POINT ( 'NONE',  ( -28.01184896238304134, 49.52604166666666430, -7.505752307972844761 ) ) ;
#13851=CARTESIAN_POINT ( 'NONE',  ( -24.18731323226221974, 57.97097249907601935, 14.01125832528330406 ) ) ;
#13858=CARTESIAN_POINT ( 'NONE',  ( 24.20753774853731244, 19.87760416666666430, -13.97622843553633132 ) ) ;
#13865=CARTESIAN_POINT ( 'NONE',  ( -14.01125832528328985, 24.45534749907602290, -24.18731323226223040 ) ) ;
#13869=CARTESIAN_POINT ( 'NONE',  ( 19.09188309203661049, 57.54687500000000000, -19.09188309203694445 ) ) ;
#13873=CARTESIAN_POINT ( 'NONE',  ( 28.01184896238304134, 23.74479166666666430, 7.505752307972846538 ) ) ;
#13874=CARTESIAN_POINT ( 'NONE',  ( 25.98046417659858420, 21.88840250092397710, 15.04653450569292872 ) ) ;
#13895=CARTESIAN_POINT ( 'NONE',  ( 24.18731323226247554, 35.63840250092398065, 14.01125832528285997 ) ) ;
#13903=CARTESIAN_POINT ( 'NONE',  ( 20.47846945139867003, 52.67149333240935505, -20.53372385742107653 ) ) ;
#13907=CARTESIAN_POINT ( 'NONE',  ( 27.95245687107222921, 23.60156250000000000, -2.463307335887066074E-13 ) ) ;
#13909=CARTESIAN_POINT ( 'NONE',  ( 7.505752307973351023, 31.19270833333333215, 28.01184896238290278 ) ) ;
#13912=CARTESIAN_POINT ( 'NONE',  ( -30.02300923189239867, 50.82069416759063785, -0.04044903254991731589 ) ) ;
#13914=CARTESIAN_POINT ( 'NONE',  ( 20.50609665441005092, 54.96875000000000000, 20.50609665440969209 ) ) ;
#13934=CARTESIAN_POINT ( 'NONE',  ( 19.06425588902592239, 11.71913166759064318, 19.11951029504763611 ) ) ;
#13939=CARTESIAN_POINT ( 'NONE',  ( -6.988114217767819270, 52.10416666666666430, 26.07999730980490583 ) ) ;
#13940=CARTESIAN_POINT ( 'NONE',  ( -15.04653450569291984, 43.37277750092397355, 25.98046417659859486 ) ) ;
#13941=CARTESIAN_POINT ( 'NONE',  ( -14.97647472619899389, 26.74701416574268720, 26.02091320914878025 ) ) ;
#13943=( GEOMETRIC_REPRESENTATION_CONTEXT ( 3 ) GLOBAL_UNCERTAINTY_ASSIGNED_CONTEXT ( ( #24689 ) ) GLOBAL_UNIT_ASSIGNED_CONTEXT ( ( #5485, #21286, #24019 ) ) REPRESENTATION_CONTEXT ( 'NONE', 'WORKASPACE' ) );
#13945=CARTESIAN_POINT ( 'NONE',  ( -7.025853678916861966, 58.97357666574269786, -26.06988505166722803 ) ) ;
#13951=CARTESIAN_POINT ( 'NONE',  ( -26.09010956794232428, 54.11496500092397355, 6.950374756619732253 ) ) ;
#13955=CARTESIAN_POINT ( 'NONE',  ( -20.50609665441004736, 25.74999999999999645, -20.50609665440969565 ) ) ;
#13959=CARTESIAN_POINT ( 'NONE',  ( 15.01150461594643204, 55.11197916666664298, 26.00068869287340334 ) ) ;
#13965=CARTESIAN_POINT ( 'NONE',  ( 7.025853678916867295, 16.00482666574268720, 26.06988505166722803 ) ) ;
#13973=CARTESIAN_POINT ( 'NONE',  ( -19.09188309203694445, 39.49999999999999289, -19.09188309203661049 ) ) ;
#13979=CARTESIAN_POINT ( 'NONE',  ( -24.22776226481240514, 64.28423583425730214, 13.94119854578937812 ) ) ;
#13982=CARTESIAN_POINT ( 'NONE',  ( 7.505752307972854531, 57.26041666666666430, -28.01184896238303423 ) ) ;
#13995=CARTESIAN_POINT ( 'NONE',  ( -6.950374756619716266, 20.59934000092397355, -26.09010956794232428 ) ) ;
#13999=CARTESIAN_POINT ( 'NONE',  ( -28.01184896238290278, 49.23958333333332860, 7.505752307973363457 ) ) ;
#14003=CARTESIAN_POINT ( 'NONE',  ( 20.50609665441005092, 34.34374999999999289, 20.50609665440969209 ) ) ;
#14009=CARTESIAN_POINT ( 'NONE',  ( 28.02196122052058413, 39.49440999907601224, 7.468012846824272799 ) ) ;
#14011=CARTESIAN_POINT ( 'NONE',  ( 28.01184896238304134, 47.80729166666666430, 7.505752307972846538 ) ) ;
#14014=CARTESIAN_POINT ( 'NONE',  ( -24.18731323226221974, 68.28347249907602645, 14.01125832528330406 ) ) ;
#14020=CARTESIAN_POINT ( 'NONE',  ( 2.584737979205442066E-13, 21.02343750000000000, 27.95245687107223276 ) ) ;
#14028=CARTESIAN_POINT ( 'NONE',  ( 24.18731323226221974, 32.18972249907602645, -14.01125832528328985 ) ) ;
#14033=CARTESIAN_POINT ( 'NONE',  ( 26.07999730980490227, 54.68229166666665719, 6.988114217767821046 ) ) ;
#14038=CARTESIAN_POINT ( 'NONE',  ( -15.01150461594642138, 25.89322916666666430, -26.00068869287340334 ) ) ;
#14039=CARTESIAN_POINT ( 'NONE',  ( -25.98046417659859486, 27.04465250092397000, -15.04653450569291628 ) ) ;
#14049=CARTESIAN_POINT ( 'NONE',  ( 0.04044903254992426173, 51.68006916759063785, -30.02300923189239867 ) ) ;
#14055=CARTESIAN_POINT ( 'NONE',  ( -19.11951029504797006, 44.93711833240935505, -19.06425588902558133 ) ) ;
#14061=CARTESIAN_POINT ( 'NONE',  ( -14.01125832528285109, 36.49777750092397355, 24.18731323226248264 ) ) ;
#14069=CARTESIAN_POINT ( 'NONE',  ( 20.53372385742108008, 53.53086833240935505, 20.47846945139866648 ) ) ;
#14074=CARTESIAN_POINT ( 'NONE',  ( 19.09188309203661049, 26.60937499999999645, -19.09188309203694445 ) ) ;
#14077=CARTESIAN_POINT ( 'NONE',  ( 28.01184896238304134, 27.18229166666666430, 7.505752307972846538 ) ) ;
#14080=CARTESIAN_POINT ( 'NONE',  ( 20.47846945139902530, 52.96913166759063785, 20.53372385742071771 ) ) ;
#14083=CARTESIAN_POINT ( 'NONE',  ( -28.01184896238290278, 62.98958333333332149, 7.505752307973363457 ) ) ;
#14104=CARTESIAN_POINT ( 'NONE',  ( -0.04044903254992426173, 15.58631916759064495, 27.95245687107223276 ) ) ;
#14109=CARTESIAN_POINT ( 'NONE',  ( 6.988114217767829928, 46.94791666666666430, -26.07999730980489872 ) ) ;
#14110=CARTESIAN_POINT ( 'NONE',  ( -15.04653450569291984, 39.93527750092397355, 25.98046417659859486 ) ) ;
#14111=CARTESIAN_POINT ( 'NONE',  ( 20.53372385742108008, 29.46836833240935505, 20.47846945139866648 ) ) ;
#14114=CARTESIAN_POINT ( 'NONE',  ( 26.09010956794244507, 60.11940999907602645, 6.950374756619249084 ) ) ;
#14121=CARTESIAN_POINT ( 'NONE',  ( 24.22776226481241224, 55.69048583425730925, -13.94119854578936923 ) ) ;
#14125=CARTESIAN_POINT ( 'NONE',  ( -7.505752307972844761, 34.91666666666666430, 28.01184896238304134 ) ) ;
#14130=CARTESIAN_POINT ( 'NONE',  ( -15.01150461594595775, 55.68489583333332860, 26.00068869287368756 ) ) ;
#14136=CARTESIAN_POINT ( 'NONE',  ( 0.04044903255045854962, 67.71055583240935505, 30.02300923189239867 ) ) ;
#14144=CARTESIAN_POINT ( 'NONE',  ( 26.07999730980490227, 44.36979166666666430, 6.988114217767821046 ) ) ;
#14150=CARTESIAN_POINT ( 'NONE',  ( -26.09010956794232428, 64.42746500092397355, 6.950374756619732253 ) ) ;
#14151=CARTESIAN_POINT ( 'NONE',  ( 15.01150461594643204, 58.54947916666665009, 26.00068869287340334 ) ) ;
#14157=CIRCLE ( 'NONE', #11333, 0.9999999999999988898 ) ;
#14162=CARTESIAN_POINT ( 'NONE',  ( 24.22776226481241224, 28.19048583425731636, -13.94119854578936923 ) ) ;
#14167=CARTESIAN_POINT ( 'NONE',  ( 28.01184896238290278, 50.95833333333332860, -7.505752307973347470 ) ) ;
#14171=CARTESIAN_POINT ( 'NONE',  ( 26.00068869287340334, 33.62760416666665719, -15.01150461594642316 ) ) ;
#14176=CARTESIAN_POINT ( 'NONE',  ( -28.00173670424535644, 40.92670166574268364, 7.543491769121936308 ) ) ;
#14178=CARTESIAN_POINT ( 'NONE',  ( 15.01150461594643382, 61.98697916666665719, 26.00068869287340334 ) ) ;
#14181=CARTESIAN_POINT ( 'NONE',  ( -26.07999730980490583, 15.15104166666666252, -6.988114217767815717 ) ) ;
#14187=CARTESIAN_POINT ( 'NONE',  ( 2.584737979205442066E-13, 34.77343750000000000, 27.95245687107223276 ) ) ;
#14194=CARTESIAN_POINT ( 'NONE',  ( 26.02091320914876960, 29.32513916574269075, 14.97647472619900455 ) ) ;
#14196=CARTESIAN_POINT ( 'NONE',  ( -19.11951029504797006, 31.18711833240935150, -19.06425588902558133 ) ) ;
#14201=CARTESIAN_POINT ( 'NONE',  ( -27.95245687107222921, 49.38281249999997868, 2.498001805406602216E-13 ) ) ;
#14206=CARTESIAN_POINT ( 'NONE',  ( 7.505752307972854531, 22.88541666666666430, -28.01184896238303423 ) ) ;
#14207=CARTESIAN_POINT ( 'NONE',  ( -20.47846945139902175, 27.18788166759063785, -20.53372385742072481 ) ) ;
#14216=CARTESIAN_POINT ( 'NONE',  ( 14.97647472619947351, 59.98736083425730925, 26.02091320914850314 ) ) ;
#14219=CARTESIAN_POINT ( 'NONE',  ( -26.00068869287368756, 25.60677083333332860, -15.01150461594595775 ) ) ;
#14224=CARTESIAN_POINT ( 'NONE',  ( -13.94119854578892514, 47.37201416574269786, 24.22776226481266448 ) ) ;
#14230=CARTESIAN_POINT ( 'NONE',  ( 6.950374756619721595, 39.50559000092398065, 26.09010956794232428 ) ) ;
#14237=CARTESIAN_POINT ( 'NONE',  ( 30.02300923189239867, 56.53868083240936215, -0.04044903255044467877 ) ) ;
#14240=CARTESIAN_POINT ( 'NONE',  ( 24.20753774853756113, 23.88802083333331794, 13.97622843553589789 ) ) ;
#14243=CARTESIAN_POINT ( 'NONE',  ( 7.505752307972854531, 29.76041666666666430, -28.01184896238303423 ) ) ;
#14246=CARTESIAN_POINT ( 'NONE',  ( 14.97647472619947351, 53.11236083425731636, 26.02091320914850314 ) ) ;
#14248=CARTESIAN_POINT ( 'NONE',  ( 2.740863092043355209E-13, 58.83593750000000000, 30.02300923189239512 ) ) ;
#14269=CARTESIAN_POINT ( 'NONE',  ( 13.94119854578937812, 11.86236083425730925, 24.22776226481240514 ) ) ;
#14274=CARTESIAN_POINT ( 'NONE',  ( 13.97622843553589966, 50.52864583333332149, -24.20753774853756113 ) ) ;
#14275=CARTESIAN_POINT ( 'NONE',  ( 7.543491769121427382, 38.07329833425730925, -28.00173670424548433 ) ) ;
#14276=CARTESIAN_POINT ( 'NONE',  ( -28.02196122052058413, 30.90065999907601579, -7.468012846824272799 ) ) ;
#14279=CARTESIAN_POINT ( 'NONE',  ( 19.11951029504797006, 56.96836833240936215, 19.06425588902558133 ) ) ;
#14288=CARTESIAN_POINT ( 'NONE',  ( -26.00068869287340334, 35.34635416666666430, 15.01150461594643382 ) ) ;
#14293=CARTESIAN_POINT ( 'NONE',  ( -30.02300923189239512, 59.69531250000000711, 2.654126918244515359E-13 ) ) ;
#14301=CARTESIAN_POINT ( 'NONE',  ( -0.04044903255042732459, 17.86680583240935860, -27.95245687107223986 ) ) ;
#14310=CARTESIAN_POINT ( 'NONE',  ( -13.97622843553588901, 38.49739583333332860, 24.20753774853756823 ) ) ;
#14315=CARTESIAN_POINT ( 'NONE',  ( 24.18731323226247554, 63.13840250092397355, 14.01125832528285997 ) ) ;
#14316=CARTESIAN_POINT ( 'NONE',  ( -7.505752307972844761, 55.54166666666667140, 28.01184896238304134 ) ) ;
#14327=CARTESIAN_POINT ( 'NONE',  ( -19.11951029504763611, 29.76600666759063429, 19.06425588902592239 ) ) ;
#14332=CARTESIAN_POINT ( 'NONE',  ( 15.01150461594596308, 50.52864583333333570, -26.00068869287367335 ) ) ;
#14336=CARTESIAN_POINT ( 'NONE',  ( 20.50609665441005092, 27.46875000000000000, 20.50609665440969209 ) ) ;
#14341=CARTESIAN_POINT ( 'NONE',  ( -0.04044903255044120238, 41.92930583240936215, -30.02300923189239867 ) ) ;
#14344=CARTESIAN_POINT ( 'NONE',  ( -26.00068869287340334, 55.97135416666665719, 15.01150461594643559 ) ) ;
#14348=CARTESIAN_POINT ( 'NONE',  ( -13.97622843553588901, 14.43489583333332682, 24.20753774853756823 ) ) ;
#14354=CARTESIAN_POINT ( 'NONE',  ( 6.988114217768294445, 31.19270833333333215, 26.07999730980477437 ) ) ;
#14359=CARTESIAN_POINT ( 'NONE',  ( 15.04653450569339945, 29.61159749907602290, 25.98046417659831775 ) ) ;
#14361=CARTESIAN_POINT ( 'NONE',  ( -19.11951029504797006, 41.49961833240934794, -19.06425588902558133 ) ) ;
#14365=CARTESIAN_POINT ( 'NONE',  ( 26.07999730980477437, 57.83333333333333570, -6.988114217768290004 ) ) ;
#14370=CARTESIAN_POINT ( 'NONE',  ( -30.02300923189239512, 28.75781249999999645, 2.654126918244515359E-13 ) ) ;
#14371=CARTESIAN_POINT ( 'NONE',  ( 30.02300923189239867, 21.60194416759064495, 0.04044903254992252006 ) ) ;
#14379=CARTESIAN_POINT ( 'NONE',  ( -14.97647472619946285, 54.83111083425730214, -26.02091320914851025 ) ) ;
#14382=CARTESIAN_POINT ( 'NONE',  ( 7.505752307973351023, 31.19270833333333215, 28.01184896238290278 ) ) ;
#14389=CARTESIAN_POINT ( 'NONE',  ( -26.09010956794245217, 48.08815999907601935, -6.950374756619243755 ) ) ;
#14397=CARTESIAN_POINT ( 'NONE',  ( -7.025853678916393008, 36.35454833425730925, 26.06988505166735592 ) ) ;
#14406=CARTESIAN_POINT ( 'NONE',  ( 14.97647472619900455, 52.52826416574268364, -26.02091320914876960 ) ) ;
#14409=CARTESIAN_POINT ( 'NONE',  ( 26.07999730980477437, 30.33333333333332860, -6.988114217768290004 ) ) ;
#14413=CARTESIAN_POINT ( 'NONE',  ( 26.00068869287340334, 26.75260416666666430, -15.01150461594642316 ) ) ;
#14416=CARTESIAN_POINT ( 'NONE',  ( 25.98046417659858420, 49.38840250092398776, 15.04653450569292872 ) ) ;
#14418=CARTESIAN_POINT ( 'NONE',  ( 28.01184896238304134, 64.99479166666665719, 7.505752307972846538 ) ) ;
#14436=CARTESIAN_POINT ( 'NONE',  ( 7.025853678916403666, 10.57329833425730747, -26.06988505166735237 ) ) ;
#14441=CARTESIAN_POINT ( 'NONE',  ( 13.97622843553633842, 51.67447916666665719, 24.20753774853730889 ) ) ;
#14442=CARTESIAN_POINT ( 'NONE',  ( 26.02091320914851025, 38.50298583425730925, -14.97647472619946463 ) ) ;
#14443=CARTESIAN_POINT ( 'NONE',  ( 25.98046417659831775, 25.31472249907601579, -15.04653450569338879 ) ) ;
#14446=CARTESIAN_POINT ( 'NONE',  ( -14.01125832528328985, 58.83034749907602645, -24.18731323226223040 ) ) ;
#14456=CARTESIAN_POINT ( 'NONE',  ( 15.01150461594643204, 31.04947916666666075, 26.00068869287340334 ) ) ;
#14460=CARTESIAN_POINT ( 'NONE',  ( 15.01150461594596308, 60.84114583333332860, -26.00068869287367335 ) ) ;
#14468=CARTESIAN_POINT ( 'NONE',  ( -14.01125832528328985, 17.58034749907602290, -24.18731323226223040 ) ) ;
#14476=CARTESIAN_POINT ( 'NONE',  ( -19.09188309203694445, 42.93750000000000000, -19.09188309203661049 ) ) ;
#14482=CARTESIAN_POINT ( 'NONE',  ( -28.00173670424549499, 13.15142333425730925, -7.543491769121417612 ) ) ;
#14483=CARTESIAN_POINT ( 'NONE',  ( -28.01184896238290278, 56.11458333333332860, 7.505752307973363457 ) ) ;
#14494=CARTESIAN_POINT ( 'NONE',  ( 24.22776226481241224, 31.62798583425730925, -13.94119854578936923 ) ) ;
#14500=CARTESIAN_POINT ( 'NONE',  ( -20.50609665441004736, 56.68749999999998579, -20.50609665440969565 ) ) ;
#14504=CARTESIAN_POINT ( 'NONE',  ( -20.50609665440969209, 31.76562499999999289, 20.50609665441005092 ) ) ;
#14509=CARTESIAN_POINT ( 'NONE',  ( 26.02091320914876960, 46.51263916574269786, 14.97647472619900455 ) ) ;
#14511=CARTESIAN_POINT ( 'NONE',  ( 20.50609665441005092, 58.40625000000000711, 20.50609665440969209 ) ) ;
#14515=CARTESIAN_POINT ( 'NONE',  ( 26.07999730980477437, 16.58333333333333215, -6.988114217768290004 ) ) ;
#14526=CARTESIAN_POINT ( 'NONE',  ( -26.02091320914878025, 24.16888916574269075, -14.97647472619899389 ) ) ;
#14528=CARTESIAN_POINT ( 'NONE',  ( -24.22776226481266448, 34.48138916574268364, -13.94119854578892514 ) ) ;
#14532=CARTESIAN_POINT ( 'NONE',  ( -27.95245687107222921, 63.13281250000000000, 2.498001805406602216E-13 ) ) ;
#14539=CARTESIAN_POINT ( 'NONE',  ( -7.505752307973343918, 32.91145833333332860, -28.01184896238290989 ) ) ;
#14540=CARTESIAN_POINT ( 'NONE',  ( 7.468012846824777284, 29.19309000092397000, 28.02196122052045268 ) ) ;
#14550=CARTESIAN_POINT ( 'NONE',  ( -30.02300923189239867, 57.69569416759065206, -0.04044903254991731589 ) ) ;
#14553=CARTESIAN_POINT ( 'NONE',  ( -20.50609665440969209, 35.20312500000000000, 20.50609665441005092 ) ) ;
#14558=CARTESIAN_POINT ( 'NONE',  ( 14.01125832528330051, 43.36159749907602645, 24.18731323226221974 ) ) ;
#14565=CARTESIAN_POINT ( 'NONE',  ( -24.18731323226248264, 51.10715250092397355, -14.01125832528284931 ) ) ;
#14571=CARTESIAN_POINT ( 'NONE',  ( -30.02300923189239867, 61.69493083240936926, 0.04044903255044988294 ) ) ;
#14575=CARTESIAN_POINT ( 'NONE',  ( 24.20753774853756113, 30.76302083333332504, 13.97622843553589789 ) ) ;
#14578=CARTESIAN_POINT ( 'NONE',  ( 28.01184896238290278, 44.08333333333332860, -7.505752307973347470 ) ) ;
#14581=CARTESIAN_POINT ( 'NONE',  ( -7.468012846824771955, 51.53684000092397355, -28.02196122052045624 ) ) ;
#14585=CARTESIAN_POINT ( 'NONE',  ( -7.505752307972844761, 58.97916666666666430, 28.01184896238304134 ) ) ;
#14607=CARTESIAN_POINT ( 'NONE',  ( -6.950374756619716266, 17.16184000092397000, -26.09010956794232428 ) ) ;
#14612=CARTESIAN_POINT ( 'NONE',  ( 6.988114217768294445, 55.25520833333333570, 26.07999730980477437 ) ) ;
#14613=CARTESIAN_POINT ( 'NONE',  ( 14.97647472619947351, 42.79986083425731636, 26.02091320914850314 ) ) ;
#14614=CARTESIAN_POINT ( 'NONE',  ( 25.98046417659831775, 39.06472249907601935, -15.04653450569338879 ) ) ;
#14617=CARTESIAN_POINT ( 'NONE',  ( 0.04044903255044120238, 53.96055583240936926, 27.95245687107223276 ) ) ;
#14619=CARTESIAN_POINT ( 'NONE',  ( -15.01150461594642138, 12.14322916666666430, -26.00068869287340334 ) ) ;
#14625=CARTESIAN_POINT ( 'NONE',  ( 28.01184896238304134, 34.05729166666666430, 7.505752307972846538 ) ) ;
#14631=CARTESIAN_POINT ( 'NONE',  ( 28.01184896238290278, 64.70833333333334281, -7.505752307973347470 ) ) ;
#14639=CARTESIAN_POINT ( 'NONE',  ( 0.04044903255044120238, 23.02305583240935860, 27.95245687107223276 ) ) ;
#14649=CARTESIAN_POINT ( 'NONE',  ( 13.97622843553589966, 53.96614583333333570, -24.20753774853756113 ) ) ;
#14654=CARTESIAN_POINT ( 'NONE',  ( -7.543491769121417612, 15.72954833425730925, 28.00173670424549499 ) ) ;
#14655=CARTESIAN_POINT ( 'NONE',  ( 7.468012846824281681, 14.57253499907601935, -28.02196122052058058 ) ) ;
#14664=CARTESIAN_POINT ( 'NONE',  ( 19.11951029504763611, 34.92225666759063074, -19.06425588902591173 ) ) ;
#14669=CARTESIAN_POINT ( 'NONE',  ( 7.505752307972854531, 64.13541666666667140, -28.01184896238303423 ) ) ;
#14673=CARTESIAN_POINT ( 'NONE',  ( 28.01184896238304134, 30.61979166666666075, 7.505752307972846538 ) ) ;
#14678=CARTESIAN_POINT ( 'NONE',  ( 30.02300923189239867, 53.10118083240936215, -0.04044903255044467877 ) ) ;
#14680=CARTESIAN_POINT ( 'NONE',  ( 15.01150461594596486, 57.40364583333332860, -26.00068869287367690 ) ) ;
#14685=CARTESIAN_POINT ( 'NONE',  ( 24.20753774853731244, 13.00260416666666430, -13.97622843553632599 ) ) ;
#14698=CARTESIAN_POINT ( 'NONE',  ( 14.97647472619900455, 25.02826416574268720, -26.02091320914876960 ) ) ;
#14700=CARTESIAN_POINT ( 'NONE',  ( -26.06988505166722803, 34.05170166574267654, 7.025853678916877953 ) ) ;
#14704=CARTESIAN_POINT ( 'NONE',  ( -19.09188309203660694, 59.26562500000000000, 19.09188309203694800 ) ) ;
#14709=CARTESIAN_POINT ( 'NONE',  ( -7.505752307972844761, 34.91666666666666430, 28.01184896238304134 ) ) ;
#14710=CARTESIAN_POINT ( 'NONE',  ( -26.02091320914849959, 33.34673583425730214, 14.97647472619947528 ) ) ;
#14719=CARTESIAN_POINT ( 'NONE',  ( -30.02300923189239867, 54.25819416759065206, -0.04044903254991731589 ) ) ;
#14722=CARTESIAN_POINT ( 'NONE',  ( 7.505752307972854531, 26.32291666666666075, -28.01184896238303423 ) ) ;
#14727=CARTESIAN_POINT ( 'NONE',  ( 24.18731323226221974, 42.50222249907603356, -14.01125832528328985 ) ) ;
#14733=CARTESIAN_POINT ( 'NONE',  ( 19.06425588902592239, 49.53163166759063785, 19.11951029504763611 ) ) ;
#14740=CARTESIAN_POINT ( 'NONE',  ( 30.02300923189239867, 66.85118083240935505, -0.04044903255044467877 ) ) ;
#14745=CARTESIAN_POINT ( 'NONE',  ( -26.07999730980477437, 38.92708333333333570, 6.988114217768305103 ) ) ;
#14748=CARTESIAN_POINT ( 'NONE',  ( -26.00068869287368756, 35.91927083333332860, -15.01150461594595775 ) ) ;
#14751=CARTESIAN_POINT ( 'NONE',  ( -15.04653450569291984, 60.56027750092398065, 25.98046417659859486 ) ) ;
#14752=CARTESIAN_POINT ( 'NONE',  ( -24.18731323226248264, 64.85715250092397355, -14.01125832528284931 ) ) ;
#14754=CARTESIAN_POINT ( 'NONE',  ( -15.01150461594642138, 63.70572916666667140, -26.00068869287340334 ) ) ;
#14774=CARTESIAN_POINT ( 'NONE',  ( -27.95245687107223986, 19.88319416759064495, -0.04044903254993292840 ) ) ;
#14779=CARTESIAN_POINT ( 'NONE',  ( -28.00173670424549499, 44.08892333425729504, -7.543491769121417612 ) ) ;
#14780=CARTESIAN_POINT ( 'NONE',  ( 26.02091320914876960, 39.63763916574268364, 14.97647472619900455 ) ) ;
#14783=CARTESIAN_POINT ( 'NONE',  ( -6.988114217768288228, 12.28645833333333037, -26.07999730980477437 ) ) ;
#14787=CARTESIAN_POINT ( 'NONE',  ( 7.505752307973351023, 14.00520833333333215, 28.01184896238290278 ) ) ;
#14794=CARTESIAN_POINT ( 'NONE',  ( 20.50609665441005092, 37.78124999999999289, 20.50609665440969209 ) ) ;
#14800=CARTESIAN_POINT ( 'NONE',  ( -15.01150461594595775, 62.55989583333332860, 26.00068869287368756 ) ) ;
#14803=CARTESIAN_POINT ( 'NONE',  ( 26.00068869287341045, 13.00260416666666430, -15.01150461594642493 ) ) ;
#14808=CARTESIAN_POINT ( 'NONE',  ( -19.11951029504797006, 24.31211833240934794, -19.06425588902558133 ) ) ;
#14816=CARTESIAN_POINT ( 'NONE',  ( 6.988114217768294445, 51.81770833333332860, 26.07999730980477437 ) ) ;
#14822=CARTESIAN_POINT ( 'NONE',  ( -28.00173670424549499, 16.58892333425730570, -7.543491769121417612 ) ) ;
#14824=CARTESIAN_POINT ( 'NONE',  ( -26.00068869287340334, 59.40885416666666430, 15.01150461594643382 ) ) ;
#14836=CARTESIAN_POINT ( 'NONE',  ( 24.18731323226247554, 32.20090250092397355, 14.01125832528285997 ) ) ;
#14837=ORIENTED_EDGE ( 'NONE', *, *, #30899, .T. ) ;
#14843=CARTESIAN_POINT ( 'NONE',  ( -20.50609665440969209, 38.64062500000000000, 20.50609665441005092 ) ) ;
#14848=CARTESIAN_POINT ( 'NONE',  ( -14.97647472619899389, 54.24701416574269075, 26.02091320914878025 ) ) ;
#14850=CARTESIAN_POINT ( 'NONE',  ( 7.505752307972854531, 60.69791666666667140, -28.01184896238303423 ) ) ;
#14855=CARTESIAN_POINT ( 'NONE',  ( 13.97622843553633665, 24.17447916666666785, 24.20753774853730889 ) ) ;
#14865=CARTESIAN_POINT ( 'NONE',  ( 7.543491769121922985, 26.31732666574268364, 28.00173670424535644 ) ) ;
#14867=CARTESIAN_POINT ( 'NONE',  ( 19.06425588902558133, 38.92149333240934794, -19.11951029504797006 ) ) ;
#14872=CARTESIAN_POINT ( 'NONE',  ( 19.09188309203694800, 65.28125000000000000, 19.09188309203660694 ) ) ;
#14878=CARTESIAN_POINT ( 'NONE',  ( -15.01150461594642138, 29.33072916666665719, -26.00068869287340334 ) ) ;
#14879=CARTESIAN_POINT ( 'NONE',  ( -25.98046417659859486, 30.48215250092397710, -15.04653450569291628 ) ) ;
#14891=CARTESIAN_POINT ( 'NONE',  ( 20.50609665440969565, 16.29687499999999645, -20.50609665441004736 ) ) ;
#14894=CARTESIAN_POINT ( 'NONE',  ( 15.01150461594643382, 31.04947916666666430, 26.00068869287340334 ) ) ;
#14897=CARTESIAN_POINT ( 'NONE',  ( -24.18731323226221974, 51.09597249907602645, 14.01125832528330406 ) ) ;
#14904=CARTESIAN_POINT ( 'NONE',  ( -0.04044903254992426173, 49.96131916759065206, 27.95245687107223276 ) ) ;
#14911=CARTESIAN_POINT ( 'NONE',  ( 0.04044903255045854962, 64.27305583240934084, 30.02300923189239867 ) ) ;
#14915=CARTESIAN_POINT ( 'NONE',  ( -6.988114217768288228, 39.78645833333332860, -26.07999730980477437 ) ) ;
#14918=CARTESIAN_POINT ( 'NONE',  ( 26.00068869287367335, 37.63802083333331439, 15.01150461594596308 ) ) ;
#14922=CARTESIAN_POINT ( 'NONE',  ( -7.468012846824771955, 58.41184000092398065, -28.02196122052045624 ) ) ;
#14923=CARTESIAN_POINT ( 'NONE',  ( -19.11951029504763611, 64.14100666759063074, 19.06425588902592239 ) ) ;
#14926=CARTESIAN_POINT ( 'NONE',  ( -26.00068869287368756, 66.85677083333334281, -15.01150461594595775 ) ) ;
#14946=CARTESIAN_POINT ( 'NONE',  ( 19.06425588902592239, 22.03163166759064495, 19.11951029504763611 ) ) ;
#14952=CARTESIAN_POINT ( 'NONE',  ( -14.97647472619946285, 47.95611083425732346, -26.02091320914851025 ) ) ;
#14955=CARTESIAN_POINT ( 'NONE',  ( -25.98046417659831420, 37.34597249907603356, 15.04653450569339945 ) ) ;
#14958=CARTESIAN_POINT ( 'NONE',  ( -13.94119854578892514, 61.12201416574268364, 24.22776226481266448 ) ) ;
#14967=CARTESIAN_POINT ( 'NONE',  ( -7.505752307973343918, 46.66145833333332860, -28.01184896238290989 ) ) ;
#14975=CARTESIAN_POINT ( 'NONE',  ( -20.50609665440969209, 14.57812499999999645, 20.50609665441005092 ) ) ;
#14979=CARTESIAN_POINT ( 'NONE',  ( 19.06425588902558133, 25.17149333240934439, -19.11951029504797006 ) ) ;
#14987=CARTESIAN_POINT ( 'NONE',  ( 19.09188309203694800, 54.96875000000000000, 19.09188309203660694 ) ) ;
#14992=CARTESIAN_POINT ( 'NONE',  ( -19.09188309203660694, 28.32812499999999645, 19.09188309203694800 ) ) ;
#14994=CARTESIAN_POINT ( 'NONE',  ( -7.543491769121417612, 19.16704833425730570, 28.00173670424549499 ) ) ;
#14995=CARTESIAN_POINT ( 'NONE',  ( -15.04653450569338524, 14.14284749907602290, -25.98046417659831775 ) ) ;
#15002=CARTESIAN_POINT ( 'NONE',  ( -6.988114217767819270, 65.85416666666665719, 26.07999730980490583 ) ) ;
#15007=CARTESIAN_POINT ( 'NONE',  ( -13.94119854578936923, 37.64361083425730925, -24.22776226481241224 ) ) ;
#15014=CARTESIAN_POINT ( 'NONE',  ( 7.505752307972854531, 40.07291666666666430, -28.01184896238303423 ) ) ;
#15020=CARTESIAN_POINT ( 'NONE',  ( 14.97647472619900455, 49.09076416574269786, -26.02091320914876960 ) ) ;
#15023=CARTESIAN_POINT ( 'NONE',  ( -28.01184896238304134, 66.71354166666665719, -7.505752307972844761 ) ) ;
#15031=CARTESIAN_POINT ( 'NONE',  ( 2.584737979205441561E-13, 24.46093749999999645, 27.95245687107222921 ) ) ;
#15044=CARTESIAN_POINT ( 'NONE',  ( -7.025853678916861966, 34.91107666574267654, -26.06988505166722803 ) ) ;
#15048=CARTESIAN_POINT ( 'NONE',  ( 19.09188309203694800, 58.40625000000000711, 19.09188309203660694 ) ) ;
#15053=CARTESIAN_POINT ( 'NONE',  ( 20.50609665440969565, 33.48437500000000000, -20.50609665441004736 ) ) ;
#15054=CARTESIAN_POINT ( 'NONE',  ( 30.02300923189239867, 28.47694416759064495, 0.04044903254992252006 ) ) ;
#15063=CARTESIAN_POINT ( 'NONE',  ( -28.00173670424549499, 64.71392333425730214, -7.543491769121417612 ) ) ;
#15066=CARTESIAN_POINT ( 'NONE',  ( 26.00068869287341045, 26.75260416666666075, -15.01150461594642493 ) ) ;
#15071=CARTESIAN_POINT ( 'NONE',  ( 26.06988505166722803, 56.39545166574268364, -7.025853678916862854 ) ) ;
#15084=CARTESIAN_POINT ( 'NONE',  ( -25.98046417659831420, 61.40847249907603356, 15.04653450569339945 ) ) ;
#15088=CARTESIAN_POINT ( 'NONE',  ( 27.95245687107222921, 37.35156249999997868, -2.463307335887066074E-13 ) ) ;
#15092=CARTESIAN_POINT ( 'NONE',  ( -20.50609665440969209, 42.07812499999999289, 20.50609665441005092 ) ) ;
#15097=CARTESIAN_POINT ( 'NONE',  ( -7.468012846824771955, 61.84934000092397355, -28.02196122052045624 ) ) ;
#15098=CARTESIAN_POINT ( 'NONE',  ( 6.950374756619721595, 60.13059000092398065, 26.09010956794232428 ) ) ;
#15101=CARTESIAN_POINT ( 'NONE',  ( -14.97647472619899389, 19.87201416574269075, 26.02091320914878025 ) ) ;
#15121=CARTESIAN_POINT ( 'NONE',  ( -26.06988505166735237, 23.46392333425730570, -7.025853678916388567 ) ) ;
#15127=CARTESIAN_POINT ( 'NONE',  ( -7.543491769121417612, 50.10454833425731636, 28.00173670424549499 ) ) ;
#15130=CARTESIAN_POINT ( 'NONE',  ( -30.02300923189239867, 41.06993083240934794, 0.04044903255044988294 ) ) ;
#15134=CARTESIAN_POINT ( 'NONE',  ( -26.09010956794245217, 61.83815999907601935, -6.950374756619243755 ) ) ;
#15143=CARTESIAN_POINT ( 'NONE',  ( -26.00068869287340334, 38.78385416666665719, 15.01150461594643382 ) ) ;
#15156=CARTESIAN_POINT ( 'NONE',  ( -24.18731323226221974, 27.03347249907602290, 14.01125832528330406 ) ) ;
#15164=CARTESIAN_POINT ( 'NONE',  ( 24.20753774853731244, 50.81510416666667140, -13.97622843553632599 ) ) ;
#15168=CARTESIAN_POINT ( 'NONE',  ( 26.07999730980490227, 27.18229166666666430, 6.988114217767821046 ) ) ;
#15169=CARTESIAN_POINT ( 'NONE',  ( 14.97647472619947351, 18.73736083425731636, 26.02091320914850314 ) ) ;
#15170=CARTESIAN_POINT ( 'NONE',  ( 26.00068869287340334, 64.56510416666667140, -15.01150461594642316 ) ) ;
#15181=CARTESIAN_POINT ( 'NONE',  ( 24.18731323226247554, 39.07590250092398065, 14.01125832528285997 ) ) ;
#15186=CARTESIAN_POINT ( 'NONE',  ( 7.505752307972854531, 16.01041666666666075, -28.01184896238303423 ) ) ;
#15190=CARTESIAN_POINT ( 'NONE',  ( -7.505752307973343918, 39.78645833333332860, -28.01184896238290989 ) ) ;
#15195=CARTESIAN_POINT ( 'NONE',  ( 28.02196122052058413, 49.80690999907602645, 7.468012846824272799 ) ) ;
#15202=CARTESIAN_POINT ( 'NONE',  ( 6.988114217767829928, 19.44791666666666075, -26.07999730980489872 ) ) ;
#15214=CARTESIAN_POINT ( 'NONE',  ( 0.04044903255044120238, 43.64805583240936215, 27.95245687107223276 ) ) ;
#15218=CARTESIAN_POINT ( 'NONE',  ( -19.09188309203694445, 63.56249999999999289, -19.09188309203661049 ) ) ;
#15222=CARTESIAN_POINT ( 'NONE',  ( -26.00068869287368756, 35.91927083333332860, -15.01150461594595775 ) ) ;
#15233=CARTESIAN_POINT ( 'NONE',  ( -20.47846945139902175, 61.56288166759063074, -20.53372385742072481 ) ) ;
#15236=CARTESIAN_POINT ( 'NONE',  ( -26.00068869287340334, 38.78385416666665719, 15.01150461594643559 ) ) ;
#15242=CARTESIAN_POINT ( 'NONE',  ( -6.950374756619247307, 54.10378499907602645, 26.09010956794245217 ) ) ;
#15247=CARTESIAN_POINT ( 'NONE',  ( -19.09188309203694445, 15.43749999999999645, -19.09188309203661049 ) ) ;
#15256=CARTESIAN_POINT ( 'NONE',  ( -19.06425588902558133, 23.45274333240935150, 19.11951029504797006 ) ) ;
#15261=CARTESIAN_POINT ( 'NONE',  ( 2.584737979205441561E-13, 38.21093750000000000, 27.95245687107222921 ) ) ;
#15264=CARTESIAN_POINT ( 'NONE',  ( 7.505752307972854531, 43.51041666666666430, -28.01184896238303423 ) ) ;
#15267=CARTESIAN_POINT ( 'NONE',  ( 0.04044903254992426173, 55.11756916759064495, -30.02300923189239867 ) ) ;
#15268=CARTESIAN_POINT ( 'NONE',  ( 24.22776226481241224, 62.56548583425730925, -13.94119854578936923 ) ) ;
#15271=CARTESIAN_POINT ( 'NONE',  ( 0.04044903255045854962, 16.14805583240936215, 30.02300923189239867 ) ) ;
#15291=CARTESIAN_POINT ( 'NONE',  ( 26.06988505166735592, 18.30767333425730214, 7.025853678916393896 ) ) ;
#15296=CARTESIAN_POINT ( 'NONE',  ( -26.02091320914849959, 50.53423583425731636, 14.97647472619947528 ) ) ;
#15298=CARTESIAN_POINT ( 'NONE',  ( -26.02091320914878025, 41.35638916574269075, -14.97647472619899389 ) ) ;
#15303=CARTESIAN_POINT ( 'NONE',  ( -26.06988505166722803, 61.55170166574269786, 7.025853678916877953 ) ) ;
#15306=CARTESIAN_POINT ( 'NONE',  ( -20.50609665440969209, 14.57812499999999645, 20.50609665441005092 ) ) ;
#15312=CARTESIAN_POINT ( 'NONE',  ( 7.505752307972854531, 43.51041666666666430, -28.01184896238303423 ) ) ;
#15313=CARTESIAN_POINT ( 'NONE',  ( -7.505752307973343918, 60.41145833333332149, -28.01184896238290989 ) ) ;
#15330=CARTESIAN_POINT ( 'NONE',  ( 24.18731323226221974, 28.75222249907602290, -14.01125832528328985 ) ) ;
#15338=CARTESIAN_POINT ( 'NONE',  ( 26.07999730980490227, 51.24479166666666430, 6.988114217767821046 ) ) ;
#15342=CARTESIAN_POINT ( 'NONE',  ( 13.97622843553589966, 29.90364583333332860, -24.20753774853756113 ) ) ;
#15344=CARTESIAN_POINT ( 'NONE',  ( -28.02196122052045268, 23.17746500092398065, 7.468012846824790607 ) ) ;
#15345=CARTESIAN_POINT ( 'NONE',  ( -20.50609665441004736, 63.56249999999999289, -20.50609665440969565 ) ) ;
#15352=CARTESIAN_POINT ( 'NONE',  ( -19.09188309203694445, 67.00000000000000000, -19.09188309203661049 ) ) ;
#15356=CARTESIAN_POINT ( 'NONE',  ( 19.06425588902592239, 46.09413166759064495, 19.11951029504763611 ) ) ;
#15360=CARTESIAN_POINT ( 'NONE',  ( -15.01150461594642138, 19.01822916666666785, -26.00068869287340334 ) ) ;
#15365=CARTESIAN_POINT ( 'NONE',  ( -15.01150461594642138, 36.20572916666666430, -26.00068869287340334 ) ) ;
#15366=FACE_OUTER_BOUND ( 'NONE', #3031, .T. ) ;
#15369=CARTESIAN_POINT ( 'NONE',  ( 20.47846945139867003, 52.67149333240935505, -20.53372385742107653 ) ) ;
#15376=CARTESIAN_POINT ( 'NONE',  ( 19.09188309203661049, 26.60937499999999645, -19.09188309203694445 ) ) ;
#15392=CARTESIAN_POINT ( 'NONE',  ( 27.95245687107223986, 11.28944416759064140, 0.04044903254993640479 ) ) ;
#15397=CARTESIAN_POINT ( 'NONE',  ( -20.50609665441004736, 39.49999999999999289, -20.50609665440969565 ) ) ;
#15409=CARTESIAN_POINT ( 'NONE',  ( 28.01184896238304134, 13.43229166666666607, 7.505752307972846538 ) ) ;
#15411=CARTESIAN_POINT ( 'NONE',  ( 15.01150461594596486, 36.77864583333332860, -26.00068869287367690 ) ) ;
#15412=SHAPE_DEFINITION_REPRESENTATION ( #8539, #8075 ) ;
#15417=CARTESIAN_POINT ( 'NONE',  ( 27.95245687107223276, 56.53868083240936215, -0.04044903255042905932 ) ) ;
#15422=CARTESIAN_POINT ( 'NONE',  ( 19.09188309203661049, 16.29687499999999645, -19.09188309203694445 ) ) ;
#15430=CARTESIAN_POINT ( 'NONE',  ( 7.025853678916867295, 16.00482666574268720, 26.06988505166722803 ) ) ;
#15435=CARTESIAN_POINT ( 'NONE',  ( 13.97622843553589966, 43.65364583333332860, -24.20753774853756113 ) ) ;
#15438=CARTESIAN_POINT ( 'NONE',  ( -26.00068869287340334, 49.09635416666665719, 15.01150461594643382 ) ) ;
#15440=CARTESIAN_POINT ( 'NONE',  ( 28.00173670424549499, 62.99517333425730214, 7.543491769121417612 ) ) ;
#15441=CARTESIAN_POINT ( 'NONE',  ( 24.18731323226247554, 59.70090250092397355, 14.01125832528285997 ) ) ;
#15444=CARTESIAN_POINT ( 'NONE',  ( -30.02300923189239512, 66.57031250000000000, 2.654126918244515359E-13 ) ) ;
#15466=CARTESIAN_POINT ( 'NONE',  ( -19.11951029504763611, 26.32850666759063785, 19.06425588902592239 ) ) ;
#15473=CARTESIAN_POINT ( 'NONE',  ( 14.97647472619900455, 49.09076416574269786, -26.02091320914876960 ) ) ;
#15477=CARTESIAN_POINT ( 'NONE',  ( -19.11951029504797006, 65.56211833240934084, -19.06425588902558133 ) ) ;
#15480=CARTESIAN_POINT ( 'NONE',  ( -7.505752307973343918, 22.59895833333332860, -28.01184896238290989 ) ) ;
#15486=CARTESIAN_POINT ( 'NONE',  ( -26.00068869287368756, 42.79427083333331439, -15.01150461594595775 ) ) ;
#15487=CARTESIAN_POINT ( 'NONE',  ( 20.50609665440969565, 60.98437499999999289, -20.50609665441004736 ) ) ;
#15502=CARTESIAN_POINT ( 'NONE',  ( -7.025853678916861966, 34.91107666574267654, -26.06988505166722803 ) ) ;
#15512=CARTESIAN_POINT ( 'NONE',  ( 24.20753774853756113, 58.26302083333332149, 13.97622843553589789 ) ) ;
#15517=CARTESIAN_POINT ( 'NONE',  ( 19.09188309203694800, 44.65624999999999289, 19.09188309203660694 ) ) ;
#15518=CARTESIAN_POINT ( 'NONE',  ( -26.02091320914849959, 19.59673583425730925, 14.97647472619947528 ) ) ;
#15519=CARTESIAN_POINT ( 'NONE',  ( 14.97647472619900455, 21.59076416574269430, -26.02091320914876960 ) ) ;
#15529=CARTESIAN_POINT ( 'NONE',  ( -14.01125832528285109, 46.81027750092398776, 24.18731323226248264 ) ) ;
#15534=CARTESIAN_POINT ( 'NONE',  ( -7.505752307972844761, 17.72916666666666430, 28.01184896238304134 ) ) ;
#15538=CARTESIAN_POINT ( 'NONE',  ( -15.01150461594595775, 38.49739583333332860, 26.00068869287368756 ) ) ;
#15543=CARTESIAN_POINT ( 'NONE',  ( 25.98046417659831775, 66.56472249907604066, -15.04653450569338879 ) ) ;
#15545=CARTESIAN_POINT ( 'NONE',  ( -28.01184896238290278, 62.98958333333332149, 7.505752307973363457 ) ) ;
#15548=CARTESIAN_POINT ( 'NONE',  ( 2.584737979205442066E-13, 62.27343749999999289, 27.95245687107223276 ) ) ;
#15551=CARTESIAN_POINT ( 'NONE',  ( -26.07999730980477437, 21.73958333333332860, 6.988114217768305103 ) ) ;
#15557=CARTESIAN_POINT ( 'NONE',  ( -26.06988505166735237, 44.08892333425729504, -7.025853678916388567 ) ) ;
#15570=CARTESIAN_POINT ( 'NONE',  ( -14.01125832528285109, 15.87277750092397710, 24.18731323226248264 ) ) ;
#15574=CARTESIAN_POINT ( 'NONE',  ( -20.50609665440969209, 42.07812499999999289, 20.50609665441005092 ) ) ;
#15586=CARTESIAN_POINT ( 'NONE',  ( 7.505752307972854531, 16.01041666666666075, -28.01184896238303423 ) ) ;
#15588=CARTESIAN_POINT ( 'NONE',  ( -28.01184896238304134, 42.65104166666666430, -7.505752307972844761 ) ) ;
#15593=CARTESIAN_POINT ( 'NONE',  ( 19.11951029504797006, 53.53086833240935505, 19.06425588902558133 ) ) ;
#15598=CARTESIAN_POINT ( 'NONE',  ( -19.09188309203694445, 11.99999999999999645, -19.09188309203661049 ) ) ;
#15606=CARTESIAN_POINT ( 'NONE',  ( -24.18731323226221974, 16.72097249907602290, 14.01125832528330406 ) ) ;
#15613=CARTESIAN_POINT ( 'NONE',  ( -6.988114217767819270, 45.22916666666665719, 26.07999730980490583 ) ) ;
#15616=CARTESIAN_POINT ( 'NONE',  ( -26.00068869287368756, 46.23177083333331439, -15.01150461594595775 ) ) ;
#15618=CARTESIAN_POINT ( 'NONE',  ( 26.00068869287367335, 17.01302083333332504, 15.01150461594596308 ) ) ;
#15619=CARTESIAN_POINT ( 'NONE',  ( -20.53372385742071771, 12.57850666759064140, 20.47846945139902530 ) ) ;
#15627=CARTESIAN_POINT ( 'NONE',  ( -28.01184896238304134, 63.27604166666667140, -7.505752307972844761 ) ) ;
#15640=CARTESIAN_POINT ( 'NONE',  ( 24.18731323226247554, 32.20090250092397355, 14.01125832528285997 ) ) ;
#15647=CARTESIAN_POINT ( 'NONE',  ( -20.47846945139866648, 50.95274333240935505, 20.53372385742108008 ) ) ;
#15651=FILL_AREA_STYLE ('',( #31415 ) ) ;
#15652=CARTESIAN_POINT ( 'NONE',  ( 19.09188309203661049, 19.73437500000000000, -19.09188309203694445 ) ) ;
#15655=CARTESIAN_POINT ( 'NONE',  ( -28.01184896238290278, 18.30208333333332860, 7.505752307973363457 ) ) ;
#15659=CARTESIAN_POINT ( 'NONE',  ( -28.02196122052045268, 40.36496500092396644, 7.468012846824790607 ) ) ;
#15662=CARTESIAN_POINT ( 'NONE',  ( -2.584737979205441561E-13, 39.92968750000000000, -30.02300923189239512 ) ) ;
#15663=CARTESIAN_POINT ( 'NONE',  ( -15.01150461594642138, 63.70572916666667140, -26.00068869287340334 ) ) ;
#15673=CARTESIAN_POINT ( 'NONE',  ( 20.50609665440969565, 19.73437500000000000, -20.50609665441004736 ) ) ;
#15678=CARTESIAN_POINT ( 'NONE',  ( -26.09010956794245217, 37.77565999907600514, -6.950374756619243755 ) ) ;
#15685=CARTESIAN_POINT ( 'NONE',  ( 6.988114217768294445, 58.69270833333332860, 26.07999730980477437 ) ) ;
#15690=CARTESIAN_POINT ( 'NONE',  ( 24.20753774853756113, 41.07552083333332149, 13.97622843553589789 ) ) ;
#15691=CARTESIAN_POINT ( 'NONE',  ( -7.543491769121417612, 29.47954833425730570, 28.00173670424549499 ) ) ;
#15692=CARTESIAN_POINT ( 'NONE',  ( 25.98046417659831775, 18.43972249907602290, -15.04653450569338879 ) ) ;
#15700=CARTESIAN_POINT ( 'NONE',  ( -7.025853678916393008, 43.22954833425730925, 26.06988505166735592 ) ) ;
#15704=CARTESIAN_POINT ( 'NONE',  ( -7.505752307973343918, 12.28645833333333037, -28.01184896238290989 ) ) ;
#15708=CARTESIAN_POINT ( 'NONE',  ( -28.01184896238290278, 52.67708333333333570, 7.505752307973363457 ) ) ;
#15715=CARTESIAN_POINT ( 'NONE',  ( 25.98046417659831775, 59.68972249907602645, -15.04653450569338879 ) ) ;
#15717=CARTESIAN_POINT ( 'NONE',  ( -28.01184896238290278, 66.42708333333332860, 7.505752307973363457 ) ) ;
#15720=CARTESIAN_POINT ( 'NONE',  ( 13.97622843553589966, 60.84114583333332860, -24.20753774853756113 ) ) ;
#15723=CARTESIAN_POINT ( 'NONE',  ( -24.20753774853730889, 31.90885416666666430, 13.97622843553633842 ) ) ;
#15729=CARTESIAN_POINT ( 'NONE',  ( 26.06988505166735592, 56.12017333425732346, 7.025853678916393896 ) ) ;
#15739=CARTESIAN_POINT ( 'NONE',  ( 24.22776226481241224, 17.87798583425730570, -13.94119854578936923 ) ) ;
#15744=CARTESIAN_POINT ( 'NONE',  ( -30.02300923189239512, 42.50781249999997868, 2.654126918244515359E-13 ) ) ;
#15748=CARTESIAN_POINT ( 'NONE',  ( -15.01150461594642138, 19.01822916666666785, -26.00068869287340334 ) ) ;
#15755=CARTESIAN_POINT ( 'NONE',  ( 7.468012846824281681, 38.63503499907601224, -28.02196122052058058 ) ) ;
#15757=CARTESIAN_POINT ( 'NONE',  ( -7.505752307973343918, 43.22395833333332860, -28.01184896238290989 ) ) ;
#15764=CARTESIAN_POINT ( 'NONE',  ( -26.06988505166722803, 64.98920166574268364, 7.025853678916877953 ) ) ;
#15769=CARTESIAN_POINT ( 'NONE',  ( -19.09188309203660694, 14.57812499999999645, 19.09188309203694800 ) ) ;
#15777=CARTESIAN_POINT ( 'NONE',  ( 26.09010956794244507, 22.30690999907601579, 6.950374756619249084 ) ) ;
#15781=CARTESIAN_POINT ( 'NONE',  ( 24.20753774853731244, 40.50260416666666430, -13.97622843553632599 ) ) ;
#15785=CARTESIAN_POINT ( 'NONE',  ( -20.50609665441004736, 11.99999999999999645, -20.50609665440969565 ) ) ;
#15786=CARTESIAN_POINT ( 'NONE',  ( -7.468012846824771955, 17.16184000092397000, -28.02196122052045624 ) ) ;
#15806=CARTESIAN_POINT ( 'NONE',  ( 13.94119854578937812, 29.04986083425730570, 24.22776226481240514 ) ) ;
#15814=CARTESIAN_POINT ( 'NONE',  ( 15.04653450569339945, 46.79909749907603356, 25.98046417659831775 ) ) ;
#15818=( LENGTH_UNIT ( ) NAMED_UNIT ( * ) SI_UNIT ( .MILLI., .METRE. ) );
#15819=CARTESIAN_POINT ( 'NONE',  ( -24.20753774853756823, 18.73177083333332149, -13.97622843553588723 ) ) ;
#15822=CARTESIAN_POINT ( 'NONE',  ( 2.740863092043355209E-13, 21.02343749999999645, 30.02300923189239512 ) ) ;
#15826=CARTESIAN_POINT ( 'NONE',  ( 0.04044903254992426173, 44.80506916759064495, -30.02300923189239867 ) ) ;
#15828=CARTESIAN_POINT ( 'NONE',  ( -2.584737979205441561E-13, 53.67968750000000000, -30.02300923189239512 ) ) ;
#15837=CARTESIAN_POINT ( 'NONE',  ( -15.01150461594595775, 17.87239583333332860, 26.00068869287368756 ) ) ;
#15842=CARTESIAN_POINT ( 'NONE',  ( -26.09010956794245217, 34.33815999907601224, -6.950374756619243755 ) ) ;
#15850=CARTESIAN_POINT ( 'NONE',  ( -19.09188309203694445, 63.56249999999999289, -19.09188309203661049 ) ) ;
#15854=CARTESIAN_POINT ( 'NONE',  ( 6.988114217768294445, 38.06770833333332860, 26.07999730980477437 ) ) ;
#15855=CARTESIAN_POINT ( 'NONE',  ( 20.53372385742072481, 31.48475666759063074, -20.47846945139902175 ) ) ;
#15856=CARTESIAN_POINT ( 'NONE',  ( 28.02196122052058413, 18.86940999907601935, 7.468012846824272799 ) ) ;
#15860=CARTESIAN_POINT ( 'NONE',  ( -24.18731323226221974, 44.22097249907603356, 14.01125832528330406 ) ) ;
#15866=CARTESIAN_POINT ( 'NONE',  ( 26.06988505166735592, 38.93267333425729504, 7.025853678916393896 ) ) ;
#15870=CARTESIAN_POINT ( 'NONE',  ( -15.01150461594642138, 12.14322916666666430, -26.00068869287340334 ) ) ;
#15874=CARTESIAN_POINT ( 'NONE',  ( -26.00068869287340334, 45.65885416666666430, 15.01150461594643382 ) ) ;
#15880=CARTESIAN_POINT ( 'NONE',  ( 28.02196122052058413, 60.11940999907602645, 7.468012846824272799 ) ) ;
#15886=CARTESIAN_POINT ( 'NONE',  ( -19.09188309203660694, 59.26562500000000000, 19.09188309203694800 ) ) ;
#15889=CARTESIAN_POINT ( 'NONE',  ( 6.988114217768294445, 34.63020833333332860, 26.07999730980477437 ) ) ;
#15895=CARTESIAN_POINT ( 'NONE',  ( -24.18731323226248264, 54.54465250092398776, -14.01125832528284931 ) ) ;
#15907=CARTESIAN_POINT ( 'NONE',  ( -0.04044903254992426173, 12.14881916759064140, 27.95245687107223276 ) ) ;
#15913=CARTESIAN_POINT ( 'NONE',  ( -15.01150461594642138, 46.51822916666666430, -26.00068869287340334 ) ) ;
#15917=CARTESIAN_POINT ( 'NONE',  ( -26.00068869287340334, 21.59635416666666785, 15.01150461594643382 ) ) ;
#15923=CARTESIAN_POINT ( 'NONE',  ( 30.02300923189239867, 32.47618083240936215, -0.04044903255044467877 ) ) ;
#15925=CARTESIAN_POINT ( 'NONE',  ( -20.50609665440969209, 42.07812499999999289, 20.50609665441005092 ) ) ;
#15931=CARTESIAN_POINT ( 'NONE',  ( -7.025853678916861966, 58.97357666574269786, -26.06988505166722803 ) ) ;
#15937=CARTESIAN_POINT ( 'NONE',  ( 2.584737979205442066E-13, 17.58593749999999645, 27.95245687107223276 ) ) ;
#15944=CARTESIAN_POINT ( 'NONE',  ( -7.025853678916861966, 21.16107666574269075, -26.06988505166722803 ) ) ;
#15949=CARTESIAN_POINT ( 'NONE',  ( -19.09188309203660694, 45.51562500000000000, 19.09188309203694800 ) ) ;
#15953=CARTESIAN_POINT ( 'NONE',  ( -7.543491769121417612, 63.85454833425732346, 28.00173670424549499 ) ) ;
#15954=CARTESIAN_POINT ( 'NONE',  ( -28.00173670424549499, 13.15142333425730925, -7.543491769121417612 ) ) ;
#15964=SURFACE_STYLE_USAGE ( .BOTH. , #318 ) ;
#15974=CARTESIAN_POINT ( 'NONE',  ( -0.04044903254992426173, 32.77381916759064495, 27.95245687107223276 ) ) ;
#15983=CARTESIAN_POINT ( 'NONE',  ( 25.98046417659831775, 49.37722249907602645, -15.04653450569338879 ) ) ;
#15987=CARTESIAN_POINT ( 'NONE',  ( -2.428612866367529427E-13, 15.86718749999999645, -27.95245687107222921 ) ) ;
#15990=CARTESIAN_POINT ( 'NONE',  ( -20.50609665441004736, 25.74999999999999645, -20.50609665440969565 ) ) ;
#15994=CARTESIAN_POINT ( 'NONE',  ( -30.02300923189239867, 43.94569416759065206, -0.04044903254991731589 ) ) ;
#15996=CARTESIAN_POINT ( 'NONE',  ( -26.00068869287368756, 49.66927083333330728, -15.01150461594595775 ) ) ;
#16007=CARTESIAN_POINT ( 'NONE',  ( -26.00068869287340334, 18.15885416666666075, 15.01150461594643559 ) ) ;
#16013=CARTESIAN_POINT ( 'NONE',  ( -19.11951029504797006, 38.06211833240934084, -19.06425588902558133 ) ) ;
#16020=CARTESIAN_POINT ( 'NONE',  ( 13.97622843553633665, 61.98697916666665009, 24.20753774853730889 ) ) ;
#16024=CARTESIAN_POINT ( 'NONE',  ( 24.20753774853756113, 37.63802083333331439, 13.97622843553589789 ) ) ;
#16025=CARTESIAN_POINT ( 'NONE',  ( 28.02196122052045268, 28.33371500092397355, -7.468012846824774620 ) ) ;
#16026=CARTESIAN_POINT ( 'NONE',  ( 30.02300923189239867, 22.16368083240936215, -0.04044903255044467877 ) ) ;
#16030=CARTESIAN_POINT ( 'NONE',  ( 19.11951029504797006, 50.09336833240935505, 19.06425588902558133 ) ) ;
#16033=VERTEX_POINT ( 'NONE', #6542 ) ;
#16036=CARTESIAN_POINT ( 'NONE',  ( -14.01125832528285109, 53.68527750092398065, 24.18731323226248264 ) ) ;
#16040=CARTESIAN_POINT ( 'NONE',  ( 15.01150461594596308, 23.02864583333332149, -26.00068869287367335 ) ) ;
#16045=CARTESIAN_POINT ( 'NONE',  ( -28.01184896238304134, 46.08854166666666430, -7.505752307972844761 ) ) ;
#16053=CARTESIAN_POINT ( 'NONE',  ( -30.02300923189239867, 65.13243083240935505, 0.04044903255044988294 ) ) ;
#16057=CARTESIAN_POINT ( 'NONE',  ( -19.09188309203694445, 56.68749999999998579, -19.09188309203661049 ) ) ;
#16060=CARTESIAN_POINT ( 'NONE',  ( -13.97622843553588901, 35.05989583333332860, 24.20753774853756823 ) ) ;
#16065=CARTESIAN_POINT ( 'NONE',  ( -27.95245687107223986, 54.25819416759065206, -0.04044903254993292840 ) ) ;
#16078=CARTESIAN_POINT ( 'NONE',  ( 6.950374756619721595, 15.44309000092397355, 26.09010956794232428 ) ) ;
#16084=CARTESIAN_POINT ( 'NONE',  ( -15.01150461594595775, 38.49739583333332860, 26.00068869287368756 ) ) ;
#16088=CARTESIAN_POINT ( 'NONE',  ( -7.505752307972844761, 21.16666666666666430, 28.01184896238304134 ) ) ;
#16096=CARTESIAN_POINT ( 'NONE',  ( -0.04044903255044120238, 35.05430583240935505, -30.02300923189239867 ) ) ;
#16098=CARTESIAN_POINT ( 'NONE',  ( -7.505752307973343918, 50.09895833333332860, -28.01184896238290989 ) ) ;
#16104=CARTESIAN_POINT ( 'NONE',  ( 6.950374756619257965, 59.26003499907601935, -26.09010956794244507 ) ) ;
#16110=CARTESIAN_POINT ( 'NONE',  ( -6.988114217768288228, 26.03645833333333215, -26.07999730980477437 ) ) ;
#16116=CARTESIAN_POINT ( 'NONE',  ( -7.025853678916861966, 24.59857666574268720, -26.06988505166722803 ) ) ;
#16119=CARTESIAN_POINT ( 'NONE',  ( -26.07999730980477437, 45.80208333333333570, 6.988114217768305103 ) ) ;
#16124=CARTESIAN_POINT ( 'NONE',  ( 7.505752307972854531, 16.01041666666666075, -28.01184896238303423 ) ) ;
#16125=CARTESIAN_POINT ( 'NONE',  ( -28.00173670424549499, 16.58892333425730570, -7.543491769121417612 ) ) ;
#16135=FILL_AREA_STYLE_COLOUR ( '', #17246 ) ;
#16147=CARTESIAN_POINT ( 'NONE',  ( 7.025853678916403666, 31.19829833425730570, -26.06988505166735237 ) ) ;
#16154=CARTESIAN_POINT ( 'NONE',  ( 7.468012846824281681, 45.51003499907601935, -28.02196122052058058 ) ) ;
#16157=CARTESIAN_POINT ( 'NONE',  ( 13.97622843553589966, 16.15364583333333215, -24.20753774853756113 ) ) ;
#16159=CARTESIAN_POINT ( 'NONE',  ( 26.00068869287340334, 23.31510416666666430, -15.01150461594642316 ) ) ;
#16163=CARTESIAN_POINT ( 'NONE',  ( 15.04653450569292872, 41.65402750092398065, -25.98046417659857710 ) ) ;
#16165=CARTESIAN_POINT ( 'NONE',  ( 7.505752307973351023, 55.25520833333333570, 28.01184896238290278 ) ) ;
#16175=CARTESIAN_POINT ( 'NONE',  ( 20.50609665440969565, 23.17187499999999289, -20.50609665441004736 ) ) ;
#16189=CARTESIAN_POINT ( 'NONE',  ( 6.988114217767829928, 64.13541666666667140, -26.07999730980489872 ) ) ;
#16193=CARTESIAN_POINT ( 'NONE',  ( -26.07999730980477437, 38.92708333333333570, 6.988114217768305103 ) ) ;
#16194=CARTESIAN_POINT ( 'NONE',  ( -26.02091320914849959, 26.47173583425730925, 14.97647472619947528 ) ) ;
#16195=CARTESIAN_POINT ( 'NONE',  ( -7.543491769121917656, 21.16107666574269075, -28.00173670424536354 ) ) ;
#16199=CARTESIAN_POINT ( 'NONE',  ( -27.95245687107223986, 47.94493083240935505, 0.04044903255043252877 ) ) ;
#16205=CARTESIAN_POINT ( 'NONE',  ( 19.06425588902592239, 52.96913166759063785, 19.11951029504763611 ) ) ;
#16209=CARTESIAN_POINT ( 'NONE',  ( -26.00068869287340334, 21.59635416666666785, 15.01150461594643382 ) ) ;
#16215=CARTESIAN_POINT ( 'NONE',  ( 2.740863092043355209E-13, 45.08593750000000711, 30.02300923189239512 ) ) ;
#16221=CARTESIAN_POINT ( 'NONE',  ( -7.543491769121917656, 65.84857666574268364, -28.00173670424536354 ) ) ;
#16226=CARTESIAN_POINT ( 'NONE',  ( 26.07999730980477437, 61.27083333333332860, -6.988114217768290004 ) ) ;
#16229=CARTESIAN_POINT ( 'NONE',  ( -24.20753774853756823, 35.91927083333332860, -13.97622843553588723 ) ) ;
#16234=CARTESIAN_POINT ( 'NONE',  ( 19.11951029504763611, 58.98475666759065206, -19.06425588902591173 ) ) ;
#16245=CARTESIAN_POINT ( 'NONE',  ( -24.18731323226248264, 27.04465250092397000, -14.01125832528284931 ) ) ;
#16250=CARTESIAN_POINT ( 'NONE',  ( 2.740863092043355209E-13, 55.39843749999999289, 30.02300923189239512 ) ) ;
#16254=CARTESIAN_POINT ( 'NONE',  ( 30.02300923189239512, 20.16406249999999645, -2.619432448724977703E-13 ) ) ;
#16260=CARTESIAN_POINT ( 'NONE',  ( -30.02300923189239867, 37.63243083240935505, 0.04044903255044988294 ) ) ;
#16262=CARTESIAN_POINT ( 'NONE',  ( -15.01150461594595775, 48.80989583333332860, 26.00068869287368756 ) ) ;
#16266=CARTESIAN_POINT ( 'NONE',  ( 26.09010956794244507, 63.55690999907603356, 6.950374756619249084 ) ) ;
#16272=CARTESIAN_POINT ( 'NONE',  ( 24.20753774853731244, 26.75260416666666075, -13.97622843553633132 ) ) ;
#16280=CARTESIAN_POINT ( 'NONE',  ( 6.950374756619257965, 24.88503499907601935, -26.09010956794244507 ) ) ;
#16283=CARTESIAN_POINT ( 'NONE',  ( -13.97622843553632421, 49.95572916666665009, -24.20753774853731599 ) ) ;
#16287=CARTESIAN_POINT ( 'NONE',  ( -7.505752307973343918, 19.16145833333332860, -28.01184896238290989 ) ) ;
#16288=CARTESIAN_POINT ( 'NONE',  ( 28.00173670424549499, 11.43267333425730925, 7.543491769121417612 ) ) ;
#16311=CARTESIAN_POINT ( 'NONE',  ( 27.95245687107223986, 35.35194416759064495, 0.04044903254993640479 ) ) ;
#16318=CARTESIAN_POINT ( 'NONE',  ( -28.02196122052058413, 54.96315999907602645, -7.468012846824272799 ) ) ;
#16322=CARTESIAN_POINT ( 'NONE',  ( -19.09188309203694445, 25.74999999999999645, -19.09188309203661049 ) ) ;
#16325=CARTESIAN_POINT ( 'NONE',  ( 20.50609665440969565, 26.60937499999999645, -20.50609665441004736 ) ) ;
#16328=CARTESIAN_POINT ( 'NONE',  ( -28.00173670424549499, 40.65142333425730214, -7.543491769121417612 ) ) ;
#16330=CARTESIAN_POINT ( 'NONE',  ( 30.02300923189239512, 54.53906249999998579, -2.619432448724977703E-13 ) ) ;
#16351=CARTESIAN_POINT ( 'NONE',  ( 7.025853678916403666, 14.01079833425730747, -26.06988505166735237 ) ) ;
#16356=CARTESIAN_POINT ( 'NONE',  ( 19.09188309203694800, 48.09375000000000000, 19.09188309203660694 ) ) ;
#16357=CARTESIAN_POINT ( 'NONE',  ( -28.02196122052045268, 30.05246500092397000, 7.468012846824790607 ) ) ;
#16358=CARTESIAN_POINT ( 'NONE',  ( -26.02091320914878025, 27.60638916574269075, -14.97647472619899389 ) ) ;
#16362=CARTESIAN_POINT ( 'NONE',  ( 19.06425588902558133, 42.35899333240935505, -19.11951029504797006 ) ) ;
#16369=CARTESIAN_POINT ( 'NONE',  ( 7.025853678916403666, 48.38579833425730925, -26.06988505166735237 ) ) ;
#16374=CARTESIAN_POINT ( 'NONE',  ( 7.505752307973351023, 24.31770833333332504, 28.01184896238290278 ) ) ;
#16378=CARTESIAN_POINT ( 'NONE',  ( 28.01184896238304134, 51.24479166666666430, 7.505752307972846538 ) ) ;
#16384=CARTESIAN_POINT ( 'NONE',  ( 28.02196122052058413, 66.99440999907601224, 7.468012846824272799 ) ) ;
#16391=CARTESIAN_POINT ( 'NONE',  ( 26.07999730980490227, 34.05729166666666430, 6.988114217767821046 ) ) ;
#16397=CARTESIAN_POINT ( 'NONE',  ( 19.06425588902592239, 59.84413166759065206, 19.11951029504763611 ) ) ;
#16411=CARTESIAN_POINT ( 'NONE',  ( -7.025853678916393008, 22.60454833425730925, 26.06988505166735592 ) ) ;
#16417=CARTESIAN_POINT ( 'NONE',  ( 15.01150461594596308, 53.96614583333333570, -26.00068869287367335 ) ) ;
#16421=CARTESIAN_POINT ( 'NONE',  ( -7.505752307972844761, 17.72916666666666430, 28.01184896238304134 ) ) ;
#16427=CARTESIAN_POINT ( 'NONE',  ( 26.02091320914876960, 36.20013916574269075, 14.97647472619900455 ) ) ;
#16429=CARTESIAN_POINT ( 'NONE',  ( -28.01184896238304134, 46.08854166666666430, -7.505752307972844761 ) ) ;
#16432=CARTESIAN_POINT ( 'NONE',  ( 19.11951029504797006, 60.40586833240935505, 19.06425588902558133 ) ) ;
#16438=CARTESIAN_POINT ( 'NONE',  ( 13.97622843553589966, 23.02864583333332504, -24.20753774853756113 ) ) ;
#16444=CARTESIAN_POINT ( 'NONE',  ( 6.950374756619257965, 28.32253499907601579, -26.09010956794244507 ) ) ;
#16448=CARTESIAN_POINT ( 'NONE',  ( -26.07999730980490583, 56.40104166666666430, -6.988114217767815717 ) ) ;
#16452=CARTESIAN_POINT ( 'NONE',  ( 2.740863092043355209E-13, 27.89843750000000000, 30.02300923189239512 ) ) ;
#16453=CARTESIAN_POINT ( 'NONE',  ( 15.04653450569292872, 24.46652750092397355, -25.98046417659857710 ) ) ;
#16470=CARTESIAN_POINT ( 'NONE',  ( 27.95245687107223986, 38.78944416759064495, 0.04044903254993640479 ) ) ;
#16476=CARTESIAN_POINT ( 'NONE',  ( 28.00173670424535644, 59.83295166574269075, -7.543491769121920321 ) ) ;
#16480=CARTESIAN_POINT ( 'NONE',  ( -13.97622843553588901, 28.18489583333332860, 24.20753774853756823 ) ) ;
#16483=CARTESIAN_POINT ( 'NONE',  ( 28.01184896238304134, 30.61979166666666075, 7.505752307972846538 ) ) ;
#16486=CARTESIAN_POINT ( 'NONE',  ( -14.97647472619946285, 47.95611083425732346, -26.02091320914851025 ) ) ;
#16489=CARTESIAN_POINT ( 'NONE',  ( -7.505752307973343918, 53.53645833333332860, -28.01184896238290989 ) ) ;
#16511=CARTESIAN_POINT ( 'NONE',  ( -0.04044903254992426173, 12.14881916759064140, 27.95245687107223276 ) ) ;
#16516=CARTESIAN_POINT ( 'NONE',  ( -19.09188309203694445, 53.25000000000000000, -19.09188309203661049 ) ) ;
#16517=CARTESIAN_POINT ( 'NONE',  ( 28.00173670424549499, 38.93267333425729504, 7.543491769121417612 ) ) ;
#16518=CARTESIAN_POINT ( 'NONE',  ( 15.04653450569339945, 29.61159749907602290, 25.98046417659831775 ) ) ;
#16522=CARTESIAN_POINT ( 'NONE',  ( 26.06988505166722803, 56.39545166574268364, -7.025853678916862854 ) ) ;
#16530=CARTESIAN_POINT ( 'NONE',  ( -6.950374756619716266, 51.53684000092397355, -26.09010956794232428 ) ) ;
#16534=CARTESIAN_POINT ( 'NONE',  ( 20.50609665440969565, 26.60937499999999645, -20.50609665441004736 ) ) ;
#16539=CARTESIAN_POINT ( 'NONE',  ( -2.584737979205441561E-13, 53.67968750000000000, -30.02300923189239512 ) ) ;
#16545=CARTESIAN_POINT ( 'NONE',  ( 26.06988505166722803, 15.14545166574268897, -7.025853678916862854 ) ) ;
#16552=CARTESIAN_POINT ( 'NONE',  ( 24.20753774853756113, 41.07552083333331439, 13.97622843553589789 ) ) ;
#16559=CARTESIAN_POINT ( 'NONE',  ( 19.06425588902592239, 63.28163166759064495, 19.11951029504763611 ) ) ;
#16561=CARTESIAN_POINT ( 'NONE',  ( 7.505752307973351023, 51.81770833333332860, 28.01184896238290278 ) ) ;
#16572=CARTESIAN_POINT ( 'NONE',  ( -7.025853678916393008, 26.04204833425729859, 26.06988505166735592 ) ) ;
#16577=CARTESIAN_POINT ( 'NONE',  ( 20.50609665440969565, 54.10937499999999289, -20.50609665441004736 ) ) ;
#16581=CARTESIAN_POINT ( 'NONE',  ( -26.00068869287340334, 31.90885416666666430, 15.01150461594643382 ) ) ;
#16587=CARTESIAN_POINT ( 'NONE',  ( -7.543491769121917656, 41.78607666574268364, -28.00173670424536354 ) ) ;
#16589=CARTESIAN_POINT ( 'NONE',  ( 7.505752307973351023, 51.81770833333332860, 28.01184896238290278 ) ) ;
#16592=CARTESIAN_POINT ( 'NONE',  ( -19.06425588902558133, 68.14024333240935505, 19.11951029504797006 ) ) ;
#16602=CARTESIAN_POINT ( 'NONE',  ( -24.20753774853730889, 21.59635416666666430, 13.97622843553634020 ) ) ;
#16609=CARTESIAN_POINT ( 'NONE',  ( -0.04044903255042732459, 31.61680583240936215, -27.95245687107223986 ) ) ;
#16613=CARTESIAN_POINT ( 'NONE',  ( 19.09188309203694800, 54.96875000000000000, 19.09188309203660694 ) ) ;
#16617=CARTESIAN_POINT ( 'NONE',  ( -15.01150461594642138, 22.45572916666666430, -26.00068869287340334 ) ) ;
#16618=CARTESIAN_POINT ( 'NONE',  ( 20.47846945139902530, 25.46913166759064140, 20.53372385742071771 ) ) ;
#16628=CARTESIAN_POINT ( 'NONE',  ( -28.02196122052045268, 54.11496500092397355, 7.468012846824790607 ) ) ;
#16633=CARTESIAN_POINT ( 'NONE',  ( 13.94119854578893580, 31.90326416574268364, -24.22776226481265383 ) ) ;
#16641=CARTESIAN_POINT ( 'NONE',  ( 19.11951029504763611, 34.92225666759063074, -19.06425588902591173 ) ) ;
#16649=CARTESIAN_POINT ( 'NONE',  ( -7.543491769121917656, 55.53607666574269075, -28.00173670424536354 ) ) ;
#16652=( NAMED_UNIT ( * ) SI_UNIT ( $, .STERADIAN. ) SOLID_ANGLE_UNIT ( ) );
#16653=CARTESIAN_POINT ( 'NONE',  ( 6.988114217767829928, 22.88541666666666430, -26.07999730980489872 ) ) ;
#16655=CARTESIAN_POINT ( 'NONE',  ( -26.00068869287340334, 31.90885416666666430, 15.01150461594643382 ) ) ;
#16658=CARTESIAN_POINT ( 'NONE',  ( 25.98046417659858420, 52.82590250092398065, 15.04653450569292872 ) ) ;
#16660=CARTESIAN_POINT ( 'NONE',  ( -7.505752307973343918, 60.41145833333332149, -28.01184896238290989 ) ) ;
#16679=CARTESIAN_POINT ( 'NONE',  ( 19.09188309203694800, 65.28125000000000000, 19.09188309203660694 ) ) ;
#16684=CARTESIAN_POINT ( 'NONE',  ( -24.20753774853756823, 46.23177083333332149, -13.97622843553588723 ) ) ;
#16685=CARTESIAN_POINT ( 'NONE',  ( 14.97647472619947351, 39.36236083425731636, 26.02091320914850314 ) ) ;
#16686=CARTESIAN_POINT ( 'NONE',  ( -7.543491769121917656, 24.59857666574268720, -28.00173670424536354 ) ) ;
#16690=CARTESIAN_POINT ( 'NONE',  ( 26.06988505166722803, 59.83295166574269075, -7.025853678916862854 ) ) ;
#16697=CARTESIAN_POINT ( 'NONE',  ( 14.01125832528286352, 48.52902750092398065, -24.18731323226246843 ) ) ;
#16702=CARTESIAN_POINT ( 'NONE',  ( 7.505752307973351023, 31.19270833333333215, 28.01184896238290278 ) ) ;
#16706=CARTESIAN_POINT ( 'NONE',  ( 26.00068869287367335, 54.82552083333331439, 15.01150461594596308 ) ) ;
#16714=CARTESIAN_POINT ( 'NONE',  ( 26.06988505166722803, 18.58295166574268364, -7.025853678916862854 ) ) ;
#16722=CARTESIAN_POINT ( 'NONE',  ( -26.07999730980477437, 45.80208333333333570, 6.988114217768305103 ) ) ;
#16728=CARTESIAN_POINT ( 'NONE',  ( 0.04044903254992426173, 10.43006916759064495, -30.02300923189239867 ) ) ;
#16729=CARTESIAN_POINT ( 'NONE',  ( 26.00068869287367335, 58.26302083333332149, 15.01150461594596308 ) ) ;
#16740=CARTESIAN_POINT ( 'NONE',  ( -26.09010956794232428, 26.61496500092397355, 6.950374756619732253 ) ) ;
#16745=CARTESIAN_POINT ( 'NONE',  ( -26.00068869287368756, 53.10677083333331439, -15.01150461594595775 ) ) ;
#16749=CARTESIAN_POINT ( 'NONE',  ( 30.02300923189239512, 30.47656250000000355, -2.619432448724977703E-13 ) ) ;
#16754=CARTESIAN_POINT ( 'NONE',  ( -28.02196122052058413, 48.08815999907601935, -7.468012846824272799 ) ) ;
#16756=CARTESIAN_POINT ( 'NONE',  ( -30.02300923189239867, 52.82031249999998579, 2.654126918244514854E-13 ) ) ;
#16759=CARTESIAN_POINT ( 'NONE',  ( 14.01125832528330051, 67.42409749907601224, 24.18731323226221974 ) ) ;
#16765=CARTESIAN_POINT ( 'NONE',  ( -19.09188309203660694, 21.45312499999999645, 19.09188309203694800 ) ) ;
#16771=CARTESIAN_POINT ( 'NONE',  ( -20.47846945139866648, 23.45274333240935150, 20.53372385742108008 ) ) ;
#16773=CARTESIAN_POINT ( 'NONE',  ( -24.22776226481266448, 27.60638916574269075, -13.94119854578892514 ) ) ;
#16777=CARTESIAN_POINT ( 'NONE',  ( -19.09188309203694445, 56.68749999999998579, -19.09188309203661049 ) ) ;
#16783=CARTESIAN_POINT ( 'NONE',  ( 7.505752307973351023, 24.31770833333332504, 28.01184896238290278 ) ) ;
#16784=CARTESIAN_POINT ( 'NONE',  ( -20.53372385742071771, 22.89100666759064495, 20.47846945139902530 ) ) ;
#16794=CARTESIAN_POINT ( 'NONE',  ( -28.00173670424549499, 54.40142333425730925, -7.543491769121417612 ) ) ;
#16796=CARTESIAN_POINT ( 'NONE',  ( 15.01150461594643382, 24.17447916666666075, 26.00068869287340334 ) ) ;
#16802=CARTESIAN_POINT ( 'NONE',  ( 14.01125832528330051, 46.79909749907603356, 24.18731323226221974 ) ) ;
#16809=CARTESIAN_POINT ( 'NONE',  ( 0.04044903254993986036, 41.36756916759064495, -27.95245687107223986 ) ) ;
#16817=CARTESIAN_POINT ( 'NONE',  ( -28.02196122052058413, 58.40065999907601935, -7.468012846824272799 ) ) ;
#16820=CARTESIAN_POINT ( 'NONE',  ( 6.988114217767829928, 29.76041666666666430, -26.07999730980489872 ) ) ;
#16823=CARTESIAN_POINT ( 'NONE',  ( -20.50609665440969209, 35.20312500000000000, 20.50609665441005092 ) ) ;
#16827=CARTESIAN_POINT ( 'NONE',  ( -28.02196122052045268, 50.67746500092398065, 7.468012846824790607 ) ) ;
#16830=CARTESIAN_POINT ( 'NONE',  ( 20.50609665440969565, 60.98437499999999289, -20.50609665441004736 ) ) ;
#16849=CARTESIAN_POINT ( 'NONE',  ( -13.97622843553588901, 65.99739583333334281, 24.20753774853756823 ) ) ;
#16854=CARTESIAN_POINT ( 'NONE',  ( -13.97622843553632777, 46.51822916666666430, -24.20753774853731599 ) ) ;
#16855=CARTESIAN_POINT ( 'NONE',  ( 7.543491769121427382, 34.63579833425730925, -28.00173670424548433 ) ) ;
#16856=CARTESIAN_POINT ( 'NONE',  ( 14.97647472619900455, 25.02826416574268720, -26.02091320914876960 ) ) ;
#16859=CARTESIAN_POINT ( 'NONE',  ( -0.04044903255042732459, 55.67930583240935505, -27.95245687107223986 ) ) ;
#16867=CARTESIAN_POINT ( 'NONE',  ( 30.02300923189239512, 37.35156249999997868, -2.619432448724977703E-13 ) ) ;
#16871=CARTESIAN_POINT ( 'NONE',  ( 7.505752307973351023, 58.69270833333332860, 28.01184896238290278 ) ) ;
#16878=CARTESIAN_POINT ( 'NONE',  ( 14.01125832528330051, 15.86159749907602112, 24.18731323226221974 ) ) ;
#16886=CARTESIAN_POINT ( 'NONE',  ( 19.09188309203694800, 37.78124999999999289, 19.09188309203660694 ) ) ;
#16892=CARTESIAN_POINT ( 'NONE',  ( 14.97647472619947351, 11.86236083425730925, 26.02091320914850314 ) ) ;
#16893=CARTESIAN_POINT ( 'NONE',  ( 15.01150461594643204, 55.11197916666664298, 26.00068869287340334 ) ) ;
#16905=CARTESIAN_POINT ( 'NONE',  ( 0.04044903254993986036, 34.49256916759064495, -27.95245687107223986 ) ) ;
#16910=CARTESIAN_POINT ( 'NONE',  ( -20.50609665440969209, 52.39062499999999289, 20.50609665441005092 ) ) ;
#16914=CARTESIAN_POINT ( 'NONE',  ( 26.00068869287340334, 30.19010416666665719, -15.01150461594642316 ) ) ;
#16920=CARTESIAN_POINT ( 'NONE',  ( 7.543491769121922985, 40.06732666574268364, 28.00173670424535644 ) ) ;
#16922=CARTESIAN_POINT ( 'NONE',  ( -7.505752307972844761, 55.54166666666667140, 28.01184896238304134 ) ) ;
#16928=CARTESIAN_POINT ( 'NONE',  ( 0.04044903255044120238, 67.71055583240935505, 27.95245687107223276 ) ) ;
#16934=CARTESIAN_POINT ( 'NONE',  ( -13.97622843553632777, 32.76822916666666430, -24.20753774853731599 ) ) ;
#16940=CARTESIAN_POINT ( 'NONE',  ( 7.468012846824281681, 24.88503499907601935, -28.02196122052058058 ) ) ;
#16942=CARTESIAN_POINT ( 'NONE',  ( 24.18731323226221974, 35.62722249907602645, -14.01125832528328985 ) ) ;
#16946=CARTESIAN_POINT ( 'NONE',  ( -2.428612866367529427E-13, 57.11718750000000711, -27.95245687107222921 ) ) ;
#16951=CARTESIAN_POINT ( 'NONE',  ( 20.50609665440969565, 26.60937499999999645, -20.50609665441004736 ) ) ;
#16952=CARTESIAN_POINT ( 'NONE',  ( -7.468012846824771955, 20.59934000092397355, -28.02196122052045624 ) ) ;
#16961=CARTESIAN_POINT ( 'NONE',  ( 30.02300923189239867, 59.41444416759064495, 0.04044903254992252006 ) ) ;
#16964=CARTESIAN_POINT ( 'NONE',  ( 30.02300923189239867, 33.91406249999998579, -2.619432448724978208E-13 ) ) ;
#16968=CARTESIAN_POINT ( 'NONE',  ( -26.06988505166722803, 47.80170166574269786, 7.025853678916877953 ) ) ;
#16974=CARTESIAN_POINT ( 'NONE',  ( 0.04044903254993986036, 37.93006916759064495, -27.95245687107223986 ) ) ;
#16982=CARTESIAN_POINT ( 'NONE',  ( 28.00173670424535644, 52.95795166574269075, -7.543491769121920321 ) ) ;
#16986=CARTESIAN_POINT ( 'NONE',  ( -6.988114217768288228, 29.47395833333332860, -26.07999730980477437 ) ) ;
#16988=CARTESIAN_POINT ( 'NONE',  ( 28.01184896238290278, 26.89583333333332860, -7.505752307973347470 ) ) ;
#16991=CARTESIAN_POINT ( 'NONE',  ( -28.02196122052045268, 54.11496500092397355, 7.468012846824790607 ) ) ;
#16994=CARTESIAN_POINT ( 'NONE',  ( 28.01184896238290278, 64.70833333333334281, -7.505752307973347470 ) ) ;
#17013=CARTESIAN_POINT ( 'NONE',  ( -19.06425588902591173, 13.43788166759064140, -19.11951029504763611 ) ) ;
#17019=CARTESIAN_POINT ( 'NONE',  ( 24.20753774853756113, 47.95052083333332149, 13.97622843553589789 ) ) ;
#17020=CARTESIAN_POINT ( 'NONE',  ( 25.98046417659858420, 42.51340250092398065, 15.04653450569292872 ) ) ;
#17022=CARTESIAN_POINT ( 'NONE',  ( -28.00173670424535644, 30.61420166574267654, 7.543491769121936308 ) ) ;
#17025=CARTESIAN_POINT ( 'NONE',  ( -19.06425588902558133, 57.82774333240935505, 19.11951029504797006 ) ) ;
#17033=CARTESIAN_POINT ( 'NONE',  ( 2.740863092043355209E-13, 31.33593749999999289, 30.02300923189239512 ) ) ;
#17038=CARTESIAN_POINT ( 'NONE',  ( -15.01150461594642138, 53.39322916666665009, -26.00068869287340334 ) ) ;
#17045=CARTESIAN_POINT ( 'NONE',  ( 30.02300923189239867, 66.85118083240935505, -0.04044903255044467877 ) ) ;
#17054=CARTESIAN_POINT ( 'NONE',  ( 24.20753774853731244, 43.94010416666665719, -13.97622843553632599 ) ) ;
#17059=CARTESIAN_POINT ( 'NONE',  ( 28.02196122052045268, 11.14621500092397532, -7.468012846824774620 ) ) ;
#17061=CARTESIAN_POINT ( 'NONE',  ( -20.50609665441004736, 56.68749999999998579, -20.50609665440969565 ) ) ;
#17072=CARTESIAN_POINT ( 'NONE',  ( 6.950374756619721595, 29.19309000092397000, 26.09010956794232428 ) ) ;
#17078=CARTESIAN_POINT ( 'NONE',  ( 28.01184896238290278, 61.27083333333332860, -7.505752307973347470 ) ) ;
#17082=CARTESIAN_POINT ( 'NONE',  ( 2.740863092043355209E-13, 27.89843750000000000, 30.02300923189239512 ) ) ;
#17087=CARTESIAN_POINT ( 'NONE',  ( -7.543491769121917656, 45.22357666574267654, -28.00173670424536354 ) ) ;
#17090=CARTESIAN_POINT ( 'NONE',  ( -20.50609665441004736, 60.12500000000000000, -20.50609665440969565 ) ) ;
#17094=CARTESIAN_POINT ( 'NONE',  ( 26.07999730980477437, 13.14583333333332860, -6.988114217768290004 ) ) ;
#17101=CARTESIAN_POINT ( 'NONE',  ( 19.09188309203694800, 30.90624999999999645, 19.09188309203660694 ) ) ;
#17106=CARTESIAN_POINT ( 'NONE',  ( 26.02091320914876960, 25.88763916574269075, 14.97647472619900455 ) ) ;
#17108=CARTESIAN_POINT ( 'NONE',  ( 19.11951029504797006, 36.34336833240934794, 19.06425588902558133 ) ) ;
#17112=CARTESIAN_POINT ( 'NONE',  ( 13.97622843553633665, 58.54947916666665009, 24.20753774853730889 ) ) ;
#17118=CARTESIAN_POINT ( 'NONE',  ( -20.50609665441004736, 22.31250000000000000, -20.50609665440969565 ) ) ;
#17119=CARTESIAN_POINT ( 'NONE',  ( -14.97647472619946285, 20.45611083425730925, -26.02091320914851025 ) ) ;
#17130=CARTESIAN_POINT ( 'NONE',  ( 26.02091320914851025, 55.69048583425730925, -14.97647472619946463 ) ) ;
#17133=CARTESIAN_POINT ( 'NONE',  ( 15.01150461594596486, 33.34114583333332860, -26.00068869287367690 ) ) ;
#17140=CARTESIAN_POINT ( 'NONE',  ( 26.09010956794244507, 42.93190999907601935, 6.950374756619249084 ) ) ;
#17146=CARTESIAN_POINT ( 'NONE',  ( 26.06988505166735592, 52.68267333425730214, 7.025853678916393896 ) ) ;
#17152=CARTESIAN_POINT ( 'NONE',  ( -26.02091320914878025, 65.41888916574268364, -14.97647472619899389 ) ) ;
#17158=CARTESIAN_POINT ( 'NONE',  ( 24.20753774853756113, 37.63802083333331439, 13.97622843553589789 ) ) ;
#17162=CARTESIAN_POINT ( 'NONE',  ( 26.00068869287340334, 37.06510416666666430, -15.01150461594642316 ) ) ;
#17165=CARTESIAN_POINT ( 'NONE',  ( 7.543491769121427382, 48.38579833425730925, -28.00173670424548433 ) ) ;
#17168=CARTESIAN_POINT ( 'NONE',  ( 20.50609665441005092, 65.28125000000000000, 20.50609665440969209 ) ) ;
#17186=CARTESIAN_POINT ( 'NONE',  ( 14.01125832528286352, 17.59152750092397355, -24.18731323226246843 ) ) ;
#17191=CARTESIAN_POINT ( 'NONE',  ( -24.20753774853730889, 55.97135416666665719, 13.97622843553634020 ) ) ;
#17192=CARTESIAN_POINT ( 'NONE',  ( -15.04653450569291984, 36.49777750092397355, 25.98046417659859486 ) ) ;
#17193=CARTESIAN_POINT ( 'NONE',  ( -30.02300923189239867, 34.19493083240935505, 0.04044903255044988294 ) ) ;
#17196=CARTESIAN_POINT ( 'NONE',  ( -24.22776226481266448, 55.10638916574269786, -13.94119854578892514 ) ) ;
#17204=CARTESIAN_POINT ( 'NONE',  ( 15.01150461594643204, 34.48697916666667140, 26.00068869287340334 ) ) ;
#17218=CARTESIAN_POINT ( 'NONE',  ( 24.22776226481265383, 25.88763916574269075, 13.94119854578893580 ) ) ;
#17225=CARTESIAN_POINT ( 'NONE',  ( 26.07999730980477437, 40.64583333333332860, -6.988114217768290004 ) ) ;
#17230=CARTESIAN_POINT ( 'NONE',  ( 20.47846945139902530, 15.15663166759064495, 20.53372385742071771 ) ) ;
#17231=CARTESIAN_POINT ( 'NONE',  ( -20.50609665440969209, 52.39062499999999289, 20.50609665441005092 ) ) ;
#17242=CARTESIAN_POINT ( 'NONE',  ( 7.025853678916403666, 31.19829833425730570, -26.06988505166735237 ) ) ;
#17246=COLOUR_RGB ( '', 0.08235294, 0.09019608, 0.10196078) ;
#17248=CARTESIAN_POINT ( 'NONE',  ( 15.01150461594643204, 61.98697916666665009, 26.00068869287340334 ) ) ;
#17252=CARTESIAN_POINT ( 'NONE',  ( -26.00068869287368756, 32.48177083333332860, -15.01150461594595775 ) ) ;
#17257=CARTESIAN_POINT ( 'NONE',  ( -15.04653450569338524, 45.08034749907603356, -25.98046417659831775 ) ) ;
#17258=CARTESIAN_POINT ( 'NONE',  ( -28.01184896238290278, 59.55208333333332149, 7.505752307973363457 ) ) ;
#17262=CARTESIAN_POINT ( 'NONE',  ( -6.988114217767819270, 17.72916666666666430, 26.07999730980490583 ) ) ;
#17273=CARTESIAN_POINT ( 'NONE',  ( 25.98046417659831775, 21.87722249907602290, -15.04653450569338879 ) ) ;
#17275=CARTESIAN_POINT ( 'NONE',  ( 13.94119854578893580, 38.77826416574269075, -24.22776226481265383 ) ) ;
#17279=CARTESIAN_POINT ( 'NONE',  ( -26.07999730980477437, 62.98958333333332149, 6.988114217768305103 ) ) ;
#17284=CARTESIAN_POINT ( 'NONE',  ( 28.01184896238304134, 30.61979166666666075, 7.505752307972846538 ) ) ;
#17285=CARTESIAN_POINT ( 'NONE',  ( 14.97647472619947351, 32.48736083425731636, 26.02091320914850314 ) ) ;
#17296=CARTESIAN_POINT ( 'NONE',  ( -15.04653450569291984, 53.68527750092398065, 25.98046417659859486 ) ) ;
#17299=CARTESIAN_POINT ( 'NONE',  ( -7.505752307973343918, 32.91145833333332860, -28.01184896238290989 ) ) ;
#17304=CARTESIAN_POINT ( 'NONE',  ( 13.94119854578893580, 45.65326416574269786, -24.22776226481265383 ) ) ;
#17311=CARTESIAN_POINT ( 'NONE',  ( 7.025853678916403666, 48.38579833425730925, -26.06988505166735237 ) ) ;
#17318=CARTESIAN_POINT ( 'NONE',  ( -7.025853678916861966, 14.28607666574268720, -26.06988505166722803 ) ) ;
#17322=CARTESIAN_POINT ( 'NONE',  ( -6.988114217768288228, 32.91145833333332860, -26.07999730980477437 ) ) ;
#17325=CARTESIAN_POINT ( 'NONE',  ( -7.505752307973343918, 43.22395833333332860, -28.01184896238290989 ) ) ;
#17328=CARTESIAN_POINT ( 'NONE',  ( 7.468012846824777284, 63.56809000092398065, 28.02196122052045268 ) ) ;
#17329=CARTESIAN_POINT ( 'NONE',  ( 0.04044903254993986036, 58.55506916759063785, -27.95245687107223986 ) ) ;
#17332=CARTESIAN_POINT ( 'NONE',  ( 20.50609665441005092, 61.84374999999998579, 20.50609665440969209 ) ) ;
#17352=CARTESIAN_POINT ( 'NONE',  ( -19.06425588902591173, 23.75038166759064140, -19.11951029504763611 ) ) ;
#17357=CARTESIAN_POINT ( 'NONE',  ( 0.04044903254992426173, 48.24256916759064495, -30.02300923189239867 ) ) ;
#17359=CARTESIAN_POINT ( 'NONE',  ( -30.02300923189239867, 37.63243083240935505, 0.04044903255044988294 ) ) ;
#17362=CARTESIAN_POINT ( 'NONE',  ( -19.11951029504797006, 68.99961833240934084, -19.06425588902558133 ) ) ;
#17366=CARTESIAN_POINT ( 'NONE',  ( 20.50609665440969565, 16.29687499999999645, -20.50609665441004736 ) ) ;
#17373=CARTESIAN_POINT ( 'NONE',  ( 20.50609665440969565, 36.92187499999999289, -20.50609665441004736 ) ) ;
#17387=CARTESIAN_POINT ( 'NONE',  ( -19.11951029504797006, 20.87461833240935505, -19.06425588902558133 ) ) ;
#17396=CARTESIAN_POINT ( 'NONE',  ( -27.95245687107222921, 52.82031249999997868, 2.498001805406602216E-13 ) ) ;
#17401=CARTESIAN_POINT ( 'NONE',  ( -20.47846945139902175, 20.31288166759063785, -20.53372385742072481 ) ) ;
#17402=CARTESIAN_POINT ( 'NONE',  ( 28.01184896238304134, 64.99479166666665719, 7.505752307972846538 ) ) ;
#17415=CARTESIAN_POINT ( 'NONE',  ( -24.22776226481240514, 29.90923583425730925, 13.94119854578937812 ) ) ;
#17421=CARTESIAN_POINT ( 'NONE',  ( -15.01150461594642138, 60.26822916666665009, -26.00068869287340334 ) ) ;
#17424=CARTESIAN_POINT ( 'NONE',  ( -15.01150461594595775, 41.93489583333333570, 26.00068869287368756 ) ) ;
#17429=CARTESIAN_POINT ( 'NONE',  ( 26.02091320914876960, 49.95013916574269786, 14.97647472619900455 ) ) ;
#17431=CARTESIAN_POINT ( 'NONE',  ( -28.01184896238304134, 59.83854166666666430, -7.505752307972844761 ) ) ;
#17436=CARTESIAN_POINT ( 'NONE',  ( -2.428612866367529427E-13, 26.17968750000000000, -27.95245687107222921 ) ) ;
#17448=CARTESIAN_POINT ( 'NONE',  ( -14.97647472619899389, 23.30951416574269075, 26.02091320914878025 ) ) ;
#17451=CARTESIAN_POINT ( 'NONE',  ( -6.950374756619247307, 40.35378499907601935, 26.09010956794245217 ) ) ;
#17455=CARTESIAN_POINT ( 'NONE',  ( 27.95245687107222921, 61.41406250000000711, -2.463307335887066074E-13 ) ) ;
#17460=CARTESIAN_POINT ( 'NONE',  ( 30.02300923189239512, 30.47656250000000355, -2.619432448724977703E-13 ) ) ;
#17461=CARTESIAN_POINT ( 'NONE',  ( 28.02196122052045268, 31.77121500092397000, -7.468012846824774620 ) ) ;
#17470=CARTESIAN_POINT ( 'NONE',  ( -26.00068869287368756, 15.29427083333332504, -15.01150461594595775 ) ) ;
#17473=CARTESIAN_POINT ( 'NONE',  ( 28.01184896238290278, 33.77083333333333570, -7.505752307973347470 ) ) ;
#17477=CARTESIAN_POINT ( 'NONE',  ( -7.025853678916861966, 45.22357666574267654, -26.06988505166722803 ) ) ;
#17484=CARTESIAN_POINT ( 'NONE',  ( 19.11951029504763611, 45.23475666759063785, -19.06425588902591173 ) ) ;
#17491=CARTESIAN_POINT ( 'NONE',  ( -28.00173670424535644, 61.55170166574269786, 7.543491769121936308 ) ) ;
#17495=CARTESIAN_POINT ( 'NONE',  ( -19.09188309203694445, 39.49999999999999289, -19.09188309203661049 ) ) ;
#17498=CARTESIAN_POINT ( 'NONE',  ( -28.01184896238290278, 35.48958333333332860, 7.505752307973363457 ) ) ;
#17501=CARTESIAN_POINT ( 'NONE',  ( 14.97647472619947351, 56.54986083425731636, 26.02091320914850314 ) ) ;
#17502=CARTESIAN_POINT ( 'NONE',  ( 6.950374756619721595, 63.56809000092398065, 26.09010956794232428 ) ) ;
#17504=CARTESIAN_POINT ( 'NONE',  ( 25.98046417659831775, 18.43972249907602290, -15.04653450569338879 ) ) ;
#17525=CARTESIAN_POINT ( 'NONE',  ( -26.09010956794232428, 19.73996500092397355, 6.950374756619732253 ) ) ;
#17529=CARTESIAN_POINT ( 'NONE',  ( -0.04044903254990864921, 46.52381916759065206, 30.02300923189239867 ) ) ;
#17531=CARTESIAN_POINT ( 'NONE',  ( -20.47846945139866648, 37.20274333240935505, 20.53372385742108008 ) ) ;
#17534=CARTESIAN_POINT ( 'NONE',  ( -26.09010956794245217, 65.27565999907601224, -6.950374756619243755 ) ) ;
#17546=CARTESIAN_POINT ( 'NONE',  ( 15.01150461594596308, 43.65364583333332860, -26.00068869287367335 ) ) ;
#17560=CARTESIAN_POINT ( 'NONE',  ( -7.025853678916861966, 28.03607666574268364, -26.06988505166722803 ) ) ;
#17568=CARTESIAN_POINT ( 'NONE',  ( 24.20753774853756113, 54.82552083333331439, 13.97622843553589789 ) ) ;
#17573=CARTESIAN_POINT ( 'NONE',  ( 28.02196122052045268, 21.45871500092397355, -7.468012846824774620 ) ) ;
#17574=CARTESIAN_POINT ( 'NONE',  ( 2.740863092043355209E-13, 62.27343749999999289, 30.02300923189239512 ) ) ;
#17580=CARTESIAN_POINT ( 'NONE',  ( 13.97622843553633842, 65.42447916666665719, 24.20753774853730889 ) ) ;
#17585=CARTESIAN_POINT ( 'NONE',  ( -26.06988505166735237, 37.21392333425730214, -7.025853678916388567 ) ) ;
#17591=CARTESIAN_POINT ( 'NONE',  ( 30.02300923189239512, 40.78906249999998579, -2.619432448724977703E-13 ) ) ;
#17596=CARTESIAN_POINT ( 'NONE',  ( -15.04653450569338524, 48.51784749907601935, -25.98046417659831775 ) ) ;
#17598=CARTESIAN_POINT ( 'NONE',  ( 28.01184896238304134, 61.55729166666666430, 7.505752307972846538 ) ) ;
#17603=CARTESIAN_POINT ( 'NONE',  ( -2.428612866367529427E-13, 22.74218749999999645, -27.95245687107222921 ) ) ;
#17615=CARTESIAN_POINT ( 'NONE',  ( 6.950374756619257965, 35.19753499907601935, -26.09010956794244507 ) ) ;
#17620=CARTESIAN_POINT ( 'NONE',  ( -13.97622843553588901, 65.99739583333334281, 24.20753774853756823 ) ) ;
#17625=CARTESIAN_POINT ( 'NONE',  ( 15.01150461594643204, 34.48697916666667140, 26.00068869287340334 ) ) ;
#17626=CARTESIAN_POINT ( 'NONE',  ( 28.00173670424549499, 35.49517333425730214, 7.543491769121417612 ) ) ;
#17638=CARTESIAN_POINT ( 'NONE',  ( 28.00173670424549499, 62.99517333425730214, 7.543491769121417612 ) ) ;
#17641=CARTESIAN_POINT ( 'NONE',  ( -20.50609665440969209, 28.32812499999999645, 20.50609665441005092 ) ) ;
#17646=CARTESIAN_POINT ( 'NONE',  ( 0.04044903255044120238, 50.52305583240934794, 27.95245687107223276 ) ) ;
#17659=CARTESIAN_POINT ( 'NONE',  ( -28.00173670424535644, 64.98920166574268364, 7.543491769121936308 ) ) ;
#17663=CARTESIAN_POINT ( 'NONE',  ( -27.95245687107222921, 32.19531250000000000, 2.498001805406602216E-13 ) ) ;
#17667=CARTESIAN_POINT ( 'NONE',  ( -7.505752307972844761, 41.79166666666666430, 28.01184896238304134 ) ) ;
#17670=CARTESIAN_POINT ( 'NONE',  ( -20.53372385742071771, 57.26600666759063785, 20.47846945139902530 ) ) ;
#17671=CARTESIAN_POINT ( 'NONE',  ( 24.18731323226247554, 63.13840250092397355, 14.01125832528285997 ) ) ;
#17674=CARTESIAN_POINT ( 'NONE',  ( -30.02300923189239867, 17.00743083240935860, 0.04044903255044988294 ) ) ;
#17696=CARTESIAN_POINT ( 'NONE',  ( 24.18731323226247554, 18.45090250092397355, 14.01125832528285997 ) ) ;
#17701=CARTESIAN_POINT ( 'NONE',  ( 14.97647472619947351, 46.23736083425730925, 26.02091320914850314 ) ) ;
#17704=CARTESIAN_POINT ( 'NONE',  ( -25.98046417659831420, 40.78347249907601935, 15.04653450569339945 ) ) ;
#17708=CARTESIAN_POINT ( 'NONE',  ( -24.22776226481266448, 65.41888916574268364, -13.94119854578892514 ) ) ;
#17711=CARTESIAN_POINT ( 'NONE',  ( 15.01150461594596308, 16.15364583333333215, -26.00068869287367335 ) ) ;
#17717=CARTESIAN_POINT ( 'NONE',  ( -15.01150461594642138, 39.64322916666667140, -26.00068869287340334 ) ) ;
#17727=CARTESIAN_POINT ( 'NONE',  ( 26.00068869287341045, 16.44010416666666430, -15.01150461594642493 ) ) ;
#17732=CARTESIAN_POINT ( 'NONE',  ( -14.01125832528328985, 21.01784749907601579, -24.18731323226223040 ) ) ;
#17739=CARTESIAN_POINT ( 'NONE',  ( -27.95245687107222921, 49.38281249999997868, 2.498001805406602216E-13 ) ) ;
#17743=CARTESIAN_POINT ( 'NONE',  ( -27.95245687107223276, 28.75781249999999645, 2.498001805406602216E-13 ) ) ;
#17744=CARTESIAN_POINT ( 'NONE',  ( -15.04653450569291984, 22.74777750092397355, 25.98046417659859486 ) ) ;
#17745=CARTESIAN_POINT ( 'NONE',  ( 2.740863092043355209E-13, 58.83593750000000000, 30.02300923189239512 ) ) ;
#17756=CARTESIAN_POINT ( 'NONE',  ( 0.04044903254993986036, 44.80506916759064495, -27.95245687107223986 ) ) ;
#17760=CARTESIAN_POINT ( 'NONE',  ( 15.01150461594643204, 17.29947916666666430, 26.00068869287340334 ) ) ;
#17764=CARTESIAN_POINT ( 'NONE',  ( -26.00068869287340334, 35.34635416666666430, 15.01150461594643382 ) ) ;
#17770=CARTESIAN_POINT ( 'NONE',  ( -28.00173670424535644, 51.23920166574269786, 7.543491769121936308 ) ) ;
#17778=CARTESIAN_POINT ( 'NONE',  ( -6.988114217768288228, 22.59895833333332860, -26.07999730980477437 ) ) ;
#17790=CARTESIAN_POINT ( 'NONE',  ( -24.18731323226221974, 47.65847249907603356, 14.01125832528330406 ) ) ;
#17795=CARTESIAN_POINT ( 'NONE',  ( 6.988114217768294445, 65.56770833333332860, 26.07999730980477437 ) ) ;
#17800=CARTESIAN_POINT ( 'NONE',  ( 7.505752307972854531, 36.63541666666666430, -28.01184896238303423 ) ) ;
#17801=CARTESIAN_POINT ( 'NONE',  ( 28.02196122052045268, 35.20871500092396644, -7.468012846824774620 ) ) ;
#17812=CARTESIAN_POINT ( 'NONE',  ( -30.02300923189239867, 61.13319416759063785, -0.04044903254991731589 ) ) ;
#17815=CARTESIAN_POINT ( 'NONE',  ( 26.00068869287367690, 41.07552083333332149, 15.01150461594596486 ) ) ;
#17819=COLOUR_RGB ( '', 0.08235294, 0.09019608, 0.10196078) ;
#17821=CARTESIAN_POINT ( 'NONE',  ( 6.950374756619257965, 48.94753499907601935, -26.09010956794244507 ) ) ;
#17826=CARTESIAN_POINT ( 'NONE',  ( -13.97622843553632777, 12.14322916666666430, -24.20753774853731599 ) ) ;
#17834=CARTESIAN_POINT ( 'NONE',  ( -20.53372385742107653, 68.99961833240934084, -20.47846945139867003 ) ) ;
#17840=CARTESIAN_POINT ( 'NONE',  ( 24.20753774853731244, 33.62760416666665719, -13.97622843553632599 ) ) ;
#17844=CARTESIAN_POINT ( 'NONE',  ( -26.00068869287368756, 42.79427083333331439, -15.01150461594595775 ) ) ;
#17847=CARTESIAN_POINT ( 'NONE',  ( 28.02196122052045268, 62.70871500092398065, -7.468012846824774620 ) ) ;
#17848=CARTESIAN_POINT ( 'NONE',  ( -0.04044903254992426173, 63.71131916759064495, 27.95245687107223276 ) ) ;
#17851=CARTESIAN_POINT ( 'NONE',  ( -25.98046417659831420, 16.72097249907602290, 15.04653450569339945 ) ) ;
#17872=CARTESIAN_POINT ( 'NONE',  ( -24.18731323226248264, 23.60715250092398421, -14.01125832528284931 ) ) ;
#17877=CARTESIAN_POINT ( 'NONE',  ( 7.468012846824777284, 49.81809000092397355, 28.02196122052045268 ) ) ;
#17879=CARTESIAN_POINT ( 'NONE',  ( 7.543491769121922985, 33.19232666574268364, 28.00173670424535644 ) ) ;
#17885=CARTESIAN_POINT ( 'NONE',  ( -27.95245687107223986, 61.69493083240936926, 0.04044903255043252877 ) ) ;
#17894=CARTESIAN_POINT ( 'NONE',  ( 15.01150461594643204, 44.79947916666667140, 26.00068869287340334 ) ) ;
#17909=CARTESIAN_POINT ( 'NONE',  ( -7.025853678916861966, 24.59857666574268720, -26.06988505166722803 ) ) ;
#17918=CARTESIAN_POINT ( 'NONE',  ( 27.95245687107222921, 47.66406249999998579, -2.463307335887066074E-13 ) ) ;
#17923=CARTESIAN_POINT ( 'NONE',  ( -2.428612866367529427E-13, 29.61718749999999645, -27.95245687107223276 ) ) ;
#17924=CARTESIAN_POINT ( 'NONE',  ( 7.543491769121427382, 17.44829833425730925, -28.00173670424548433 ) ) ;
#17925=CARTESIAN_POINT ( 'NONE',  ( 30.02300923189239512, 61.41406250000000711, -2.619432448724977703E-13 ) ) ;
#17936=CARTESIAN_POINT ( 'NONE',  ( -6.950374756619716266, 41.22434000092397355, -26.09010956794232428 ) ) ;
#17940=CARTESIAN_POINT ( 'NONE',  ( 30.02300923189239512, 20.16406249999999645, -2.619432448724977703E-13 ) ) ;
#17944=CARTESIAN_POINT ( 'NONE',  ( -7.505752307972844761, 41.79166666666666430, 28.01184896238304134 ) ) ;
#17950=CARTESIAN_POINT ( 'NONE',  ( 14.97647472619900455, 55.96576416574269786, -26.02091320914876960 ) ) ;
#17957=CARTESIAN_POINT ( 'NONE',  ( -13.97622843553588901, 24.74739583333332504, 24.20753774853756823 ) ) ;
#17972=CARTESIAN_POINT ( 'NONE',  ( 14.01125832528286352, 10.71652750092397888, -24.18731323226246843 ) ) ;
#17977=CARTESIAN_POINT ( 'NONE',  ( -2.584737979205441561E-13, 46.80468750000000000, -30.02300923189239512 ) ) ;
#17990=CARTESIAN_POINT ( 'NONE',  ( 20.50609665441005092, 13.71874999999999467, 20.50609665440969209 ) ) ;
#17993=CARTESIAN_POINT ( 'NONE',  ( 20.50609665440969565, 40.35937499999999289, -20.50609665441004736 ) ) ;
#17999=CARTESIAN_POINT ( 'NONE',  ( -0.04044903255042732459, 52.24180583240936215, -27.95245687107223986 ) ) ;
#18011=CARTESIAN_POINT ( 'NONE',  ( 19.06425588902558133, 14.85899333240935505, -19.11951029504797006 ) ) ;
#18016=CARTESIAN_POINT ( 'NONE',  ( 19.09188309203661049, 40.35937499999999289, -19.09188309203694445 ) ) ;
#18019=CARTESIAN_POINT ( 'NONE',  ( 15.01150461594596308, 47.09114583333332860, -26.00068869287367335 ) ) ;
#18021=CARTESIAN_POINT ( 'NONE',  ( 0.04044903254992426173, 58.55506916759063785, -30.02300923189239867 ) ) ;
#18022=CARTESIAN_POINT ( 'NONE',  ( 19.06425588902592239, 59.84413166759065206, 19.11951029504763611 ) ) ;
#18025=CARTESIAN_POINT ( 'NONE',  ( 30.02300923189239867, 18.72618083240936215, -0.04044903255044467877 ) ) ;
#18030=CARTESIAN_POINT ( 'NONE',  ( 15.01150461594643204, 65.42447916666667140, 26.00068869287340334 ) ) ;
#18044=CARTESIAN_POINT ( 'NONE',  ( -0.04044903254992426173, 29.33631916759064850, 27.95245687107223276 ) ) ;
#18050=CARTESIAN_POINT ( 'NONE',  ( -28.00173670424535644, 44.36420166574269075, 7.543491769121936308 ) ) ;
#18053=CARTESIAN_POINT ( 'NONE',  ( 19.11951029504797006, 63.84336833240935505, 19.06425588902558133 ) ) ;
#18055=CARTESIAN_POINT ( 'NONE',  ( -7.505752307973343918, 19.16145833333332860, -28.01184896238290989 ) ) ;
#18061=CARTESIAN_POINT ( 'NONE',  ( -28.01184896238304134, 46.08854166666666430, -7.505752307972844761 ) ) ;
#18062=CARTESIAN_POINT ( 'NONE',  ( 20.50609665441005092, 58.40625000000000711, 20.50609665440969209 ) ) ;
#18075=CARTESIAN_POINT ( 'NONE',  ( -19.06425588902558133, 30.32774333240935150, 19.11951029504797006 ) ) ;
#18084=CARTESIAN_POINT ( 'NONE',  ( 27.95245687107222921, 51.10156249999998579, -2.463307335887066074E-13 ) ) ;
#18088=CARTESIAN_POINT ( 'NONE',  ( -24.20753774853756823, 42.79427083333332149, -13.97622843553588723 ) ) ;
#18090=CARTESIAN_POINT ( 'NONE',  ( -30.02300923189239867, 19.88319416759064495, -0.04044903254991731589 ) ) ;
#18091=CARTESIAN_POINT ( 'NONE',  ( -30.02300923189239512, 66.57031250000000000, 2.654126918244515359E-13 ) ) ;
#18100=CARTESIAN_POINT ( 'NONE',  ( 26.09010956794232428, 38.64621500092395934, -6.950374756619718042 ) ) ;
#18104=CARTESIAN_POINT ( 'NONE',  ( 26.00068869287340334, 16.44010416666666430, -15.01150461594642316 ) ) ;
#18108=CARTESIAN_POINT ( 'NONE',  ( -28.01184896238290278, 35.48958333333332860, 7.505752307973363457 ) ) ;
#18115=CARTESIAN_POINT ( 'NONE',  ( 20.47846945139867003, 62.98399333240935505, -20.53372385742107653 ) ) ;
#18117=CARTESIAN_POINT ( 'NONE',  ( -26.00068869287368756, 63.41927083333333570, -15.01150461594595775 ) ) ;
#18120=CARTESIAN_POINT ( 'NONE',  ( -2.428612866367529427E-13, 63.99218749999997868, -27.95245687107223276 ) ) ;
#18125=CARTESIAN_POINT ( 'NONE',  ( 24.20753774853756113, 23.88802083333331794, 13.97622843553589789 ) ) ;
#18133=CARTESIAN_POINT ( 'NONE',  ( -7.025853678916393008, 50.10454833425731636, 26.06988505166735592 ) ) ;
#18144=CARTESIAN_POINT ( 'NONE',  ( -27.95245687107223986, 13.00819416759064318, -0.04044903254993292840 ) ) ;
#18148=CARTESIAN_POINT ( 'NONE',  ( 2.740863092043355209E-13, 38.21093750000000000, 30.02300923189239512 ) ) ;
#18151=DIRECTION ( 'NONE',  ( -0.7069718413157914938, -0.01953538259431466736, 0.7069718413158002646 ) ) ;
#18159=CARTESIAN_POINT ( 'NONE',  ( -20.50609665441004736, 11.99999999999999645, -20.50609665440969565 ) ) ;
#18161=CARTESIAN_POINT ( 'NONE',  ( -15.01150461594642316, 36.20572916666665719, -26.00068869287341045 ) ) ;
#18167=CARTESIAN_POINT ( 'NONE',  ( 26.06988505166722803, 49.52045166574269075, -7.025853678916862854 ) ) ;
#18181=CARTESIAN_POINT ( 'NONE',  ( 6.950374756619257965, 21.44753499907601579, -26.09010956794244507 ) ) ;
#18186=CARTESIAN_POINT ( 'NONE',  ( 24.20753774853756113, 41.07552083333331439, 13.97622843553589789 ) ) ;
#18190=CARTESIAN_POINT ( 'NONE',  ( -7.505752307972844761, 45.22916666666665719, 28.01184896238304134 ) ) ;
#18192=CARTESIAN_POINT ( 'NONE',  ( 28.01184896238290278, 13.14583333333332860, -7.505752307973347470 ) ) ;
#18193=CARTESIAN_POINT ( 'NONE',  ( 20.47846945139902530, 18.59413166759064140, 20.53372385742071771 ) ) ;
#18215=CARTESIAN_POINT ( 'NONE',  ( 24.18731323226247554, 28.76340250092398065, 14.01125832528285997 ) ) ;
#18223=CARTESIAN_POINT ( 'NONE',  ( -7.468012846824272799, 50.66628499907601935, 28.02196122052058413 ) ) ;
#18226=CARTESIAN_POINT ( 'NONE',  ( 6.988114217768294445, 14.00520833333333215, 26.07999730980477437 ) ) ;
#18229=CARTESIAN_POINT ( 'NONE',  ( -26.00068869287368756, 22.16927083333332504, -15.01150461594595775 ) ) ;
#18233=CARTESIAN_POINT ( 'NONE',  ( -7.543491769121417612, 43.22954833425730925, 28.00173670424549499 ) ) ;
#18235=CARTESIAN_POINT ( 'NONE',  ( -28.01184896238304134, 39.21354166666666430, -7.505752307972844761 ) ) ;
#18236=CARTESIAN_POINT ( 'NONE',  ( -26.00068869287340334, 62.84635416666667851, 15.01150461594643382 ) ) ;
#18245=CARTESIAN_POINT ( 'NONE',  ( -26.00068869287368756, 18.73177083333332504, -15.01150461594595775 ) ) ;
#18250=CARTESIAN_POINT ( 'NONE',  ( 26.09010956794244507, 36.05690999907600514, 6.950374756619249084 ) ) ;
#18258=CARTESIAN_POINT ( 'NONE',  ( -13.97622843553588901, 59.12239583333333570, 24.20753774853756823 ) ) ;
#18262=CARTESIAN_POINT ( 'NONE',  ( 19.09188309203661049, 36.92187499999999289, -19.09188309203694445 ) ) ;
#18263=CARTESIAN_POINT ( 'NONE',  ( 20.47846945139902530, 32.34413166759064495, 20.53372385742071771 ) ) ;
#18264=CARTESIAN_POINT ( 'NONE',  ( 20.47846945139867003, 18.29649333240935150, -20.53372385742107653 ) ) ;
#18275=CARTESIAN_POINT ( 'NONE',  ( -27.95245687107223986, 40.50819416759064495, -0.04044903254993292840 ) ) ;
#18281=CARTESIAN_POINT ( 'NONE',  ( -30.02300923189239512, 18.44531249999999645, 2.654126918244515359E-13 ) ) ;
#18285=CARTESIAN_POINT ( 'NONE',  ( 30.02300923189239512, 47.66406249999998579, -2.619432448724977703E-13 ) ) ;
#18290=CARTESIAN_POINT ( 'NONE',  ( 20.47846945139867003, 59.54649333240936215, -20.53372385742107653 ) ) ;
#18295=CARTESIAN_POINT ( 'NONE',  ( 19.09188309203694800, 58.40625000000000711, 19.09188309203660694 ) ) ;
#18298=CARTESIAN_POINT ( 'NONE',  ( 19.09188309203661049, 33.48437500000000000, -19.09188309203694445 ) ) ;
#18304=CARTESIAN_POINT ( 'NONE',  ( 27.95245687107223986, 49.10194416759064495, 0.04044903254993640479 ) ) ;
#18305=CIRCLE ( 'NONE', #3484, 0.9999999999999988898 ) ;
#18316=CARTESIAN_POINT ( 'NONE',  ( -6.950374756619716266, 13.72434000092397532, -26.09010956794232428 ) ) ;
#18320=CARTESIAN_POINT ( 'NONE',  ( 20.50609665440969565, 40.35937499999999289, -20.50609665441004736 ) ) ;
#18324=CARTESIAN_POINT ( 'NONE',  ( -2.584737979205441561E-13, 22.74218749999999645, -30.02300923189239512 ) ) ;
#18331=CARTESIAN_POINT ( 'NONE',  ( -14.97647472619899389, 33.62201416574269075, 26.02091320914878025 ) ) ;
#18333=CARTESIAN_POINT ( 'NONE',  ( 2.740863092043355209E-13, 41.64843749999999289, 30.02300923189239867 ) ) ;
#18338=CARTESIAN_POINT ( 'NONE',  ( 0.04044903255044120238, 53.96055583240936926, 27.95245687107223276 ) ) ;
#18343=CARTESIAN_POINT ( 'NONE',  ( 24.20753774853731244, 16.44010416666666430, -13.97622843553633132 ) ) ;
#18345=( GEOMETRIC_REPRESENTATION_CONTEXT ( 3 ) GLOBAL_UNCERTAINTY_ASSIGNED_CONTEXT ( ( #6159 ) ) GLOBAL_UNIT_ASSIGNED_CONTEXT ( ( #146, #20780, #33809 ) ) REPRESENTATION_CONTEXT ( 'NONE', 'WORKASPACE' ) );
#18353=CARTESIAN_POINT ( 'NONE',  ( 26.09010956794244507, 15.43190999907601935, 6.950374756619249084 ) ) ;
#18357=CARTESIAN_POINT ( 'NONE',  ( 6.988114217767829928, 46.94791666666666430, -26.07999730980489872 ) ) ;
#18362=CARTESIAN_POINT ( 'NONE',  ( 15.01150461594643204, 17.29947916666666430, 26.00068869287340334 ) ) ;
#18363=CARTESIAN_POINT ( 'NONE',  ( 20.53372385742072481, 10.85975666759064318, -20.47846945139902175 ) ) ;
#18382=CARTESIAN_POINT ( 'NONE',  ( -7.025853678916393008, 26.04204833425729859, 26.06988505166735592 ) ) ;
#18389=CARTESIAN_POINT ( 'NONE',  ( -30.02300923189239867, 47.94493083240935505, 0.04044903255044988294 ) ) ;
#18393=CARTESIAN_POINT ( 'NONE',  ( 24.20753774853731244, 19.87760416666666430, -13.97622843553632599 ) ) ;
#18396=CARTESIAN_POINT ( 'NONE',  ( -7.505752307972844761, 24.60416666666666430, 28.01184896238304134 ) ) ;
#18400=CARTESIAN_POINT ( 'NONE',  ( -7.468012846824771955, 37.78684000092396644, -28.02196122052045624 ) ) ;
#18403=CARTESIAN_POINT ( 'NONE',  ( -26.00068869287368756, 56.54427083333332149, -15.01150461594595775 ) ) ;
#18414=CARTESIAN_POINT ( 'NONE',  ( -26.00068869287340334, 25.03385416666666430, 15.01150461594643559 ) ) ;
#18421=CARTESIAN_POINT ( 'NONE',  ( 6.950374756619257965, 31.76003499907602290, -26.09010956794244507 ) ) ;
#18428=CARTESIAN_POINT ( 'NONE',  ( -26.07999730980490583, 56.40104166666666430, -6.988114217767815717 ) ) ;
#18433=CARTESIAN_POINT ( 'NONE',  ( 19.09188309203694800, 37.78124999999999289, 19.09188309203660694 ) ) ;
#18434=CARTESIAN_POINT ( 'NONE',  ( -28.00173670424549499, 26.90142333425731280, -7.543491769121417612 ) ) ;
#18435=CARTESIAN_POINT ( 'NONE',  ( -7.468012846824272799, 16.29128499907601579, 28.02196122052058413 ) ) ;
#18439=CARTESIAN_POINT ( 'NONE',  ( -7.025853678916861966, 48.66107666574268364, -26.06988505166722803 ) ) ;
#18445=CARTESIAN_POINT ( 'NONE',  ( 24.22776226481241224, 41.94048583425730925, -13.94119854578936923 ) ) ;
#18449=CARTESIAN_POINT ( 'NONE',  ( 20.50609665441005092, 13.71874999999999467, 20.50609665440969209 ) ) ;
#18453=CARTESIAN_POINT ( 'NONE',  ( -2.584737979205441561E-13, 50.24218750000000711, -30.02300923189239512 ) ) ;
#18458=CARTESIAN_POINT ( 'NONE',  ( 25.98046417659831775, 63.12722249907601224, -15.04653450569338879 ) ) ;
#18462=CARTESIAN_POINT ( 'NONE',  ( 6.988114217768294445, 58.69270833333332860, 26.07999730980477437 ) ) ;
#18465=CARTESIAN_POINT ( 'NONE',  ( 6.988114217767829928, 29.76041666666666430, -26.07999730980489872 ) ) ;
#18472=CARTESIAN_POINT ( 'NONE',  ( 24.18731323226247554, 56.26340250092398065, 14.01125832528285997 ) ) ;
#18484=CARTESIAN_POINT ( 'NONE',  ( 26.06988505166735592, 18.30767333425730214, 7.025853678916393896 ) ) ;
#18490=CARTESIAN_POINT ( 'NONE',  ( 20.50609665440969565, 43.79687500000000000, -20.50609665441004736 ) ) ;
#18494=CARTESIAN_POINT ( 'NONE',  ( 15.01150461594596308, 23.02864583333332149, -26.00068869287367335 ) ) ;
#18500=CARTESIAN_POINT ( 'NONE',  ( 28.02196122052058413, 36.05690999907600514, 7.468012846824272799 ) ) ;
#18502=CARTESIAN_POINT ( 'NONE',  ( 28.01184896238290278, 37.20833333333332860, -7.505752307973347470 ) ) ;
#18508=CARTESIAN_POINT ( 'NONE',  ( -27.95245687107223986, 58.25743083240935505, 0.04044903255043252877 ) ) ;
#18521=CARTESIAN_POINT ( 'NONE',  ( 26.09010956794244507, 18.86940999907601935, 6.950374756619249084 ) ) ;
#18525=CARTESIAN_POINT ( 'NONE',  ( 24.20753774853731244, 47.37760416666666430, -13.97622843553632599 ) ) ;
#18529=CARTESIAN_POINT ( 'NONE',  ( 7.505752307973351023, 14.00520833333333215, 28.01184896238290278 ) ) ;
#18530=CARTESIAN_POINT ( 'NONE',  ( -0.04044903254990864921, 12.14881916759064140, 30.02300923189239867 ) ) ;
#18550=CARTESIAN_POINT ( 'NONE',  ( -26.09010956794232428, 26.61496500092397355, 6.950374756619732253 ) ) ;
#18554=ADVANCED_BREP_SHAPE_REPRESENTATION ( '', ( #32186, #1376 ), #13943 ) ;
#18558=CARTESIAN_POINT ( 'NONE',  ( -7.468012846824272799, 47.22878499907602645, 28.02196122052058413 ) ) ;
#18563=CARTESIAN_POINT ( 'NONE',  ( 27.95245687107222921, 16.72656249999999645, -2.463307335887066074E-13 ) ) ;
#18566=CARTESIAN_POINT ( 'NONE',  ( 20.50609665440969565, 19.73437500000000000, -20.50609665441004736 ) ) ;
#18572=CARTESIAN_POINT ( 'NONE',  ( -15.04653450569291984, 36.49777750092397355, 25.98046417659859486 ) ) ;
#18574=CARTESIAN_POINT ( 'NONE',  ( -15.01150461594595775, 52.24739583333332860, 26.00068869287368756 ) ) ;
#18584=CARTESIAN_POINT ( 'NONE',  ( -7.505752307973343918, 19.16145833333332860, -28.01184896238290989 ) ) ;
#18589=CARTESIAN_POINT ( 'NONE',  ( -14.01125832528328985, 34.76784749907601935, -24.18731323226223040 ) ) ;
#18596=CARTESIAN_POINT ( 'NONE',  ( 13.97622843553589966, 60.84114583333332860, -24.20753774853756113 ) ) ;
#18600=CARTESIAN_POINT ( 'NONE',  ( 6.988114217767829928, 36.63541666666666430, -26.07999730980489872 ) ) ;
#18601=CARTESIAN_POINT ( 'NONE',  ( -14.97647472619946285, 27.33111083425731280, -26.02091320914851025 ) ) ;
#18603=CARTESIAN_POINT ( 'NONE',  ( 14.97647472619900455, 14.71576416574268720, -26.02091320914876960 ) ) ;
#18607=CARTESIAN_POINT ( 'NONE',  ( -26.06988505166722803, 44.36420166574269075, 7.025853678916877953 ) ) ;
#18614=CARTESIAN_POINT ( 'NONE',  ( 24.22776226481241224, 48.81548583425731636, -13.94119854578936923 ) ) ;
#18619=CARTESIAN_POINT ( 'NONE',  ( -20.50609665441004736, 29.18749999999999645, -20.50609665440969565 ) ) ;
#18624=CARTESIAN_POINT ( 'NONE',  ( 20.50609665441005092, 48.09375000000000000, 20.50609665440969209 ) ) ;
#18630=CARTESIAN_POINT ( 'NONE',  ( -14.97647472619899389, 64.55951416574268364, 26.02091320914878025 ) ) ;
#18635=CARTESIAN_POINT ( 'NONE',  ( -26.07999730980490583, 59.83854166666666430, -6.988114217767815717 ) ) ;
#18638=CARTESIAN_POINT ( 'NONE',  ( -6.988114217767819270, 34.91666666666666430, 26.07999730980490583 ) ) ;
#18643=CARTESIAN_POINT ( 'NONE',  ( 6.950374756619721595, 60.13059000092398065, 26.09010956794232428 ) ) ;
#18654=CARTESIAN_POINT ( 'NONE',  ( 27.95245687107223986, 14.72694416759064318, 0.04044903254993640479 ) ) ;
#18659=CARTESIAN_POINT ( 'NONE',  ( 15.01150461594596308, 40.21614583333332860, -26.00068869287367335 ) ) ;
#18663=CARTESIAN_POINT ( 'NONE',  ( -26.00068869287368756, 18.73177083333332149, -15.01150461594595775 ) ) ;
#18669=CARTESIAN_POINT ( 'NONE',  ( -20.47846945139866648, 30.32774333240935150, 20.53372385742108008 ) ) ;
#18671=CARTESIAN_POINT ( 'NONE',  ( 15.01150461594643382, 44.79947916666667140, 26.00068869287340334 ) ) ;
#18677=CARTESIAN_POINT ( 'NONE',  ( -19.11951029504797006, 62.12461833240934794, -19.06425588902558133 ) ) ;
#18684=CARTESIAN_POINT ( 'NONE',  ( 19.09188309203661049, 23.17187499999999289, -19.09188309203694445 ) ) ;
#18691=CARTESIAN_POINT ( 'NONE',  ( 6.950374756619257965, 14.57253499907601935, -26.09010956794244507 ) ) ;
#18694=CARTESIAN_POINT ( 'NONE',  ( -2.428612866367529427E-13, 39.92968750000000000, -27.95245687107222921 ) ) ;
#18699=CARTESIAN_POINT ( 'NONE',  ( -28.01184896238304134, 18.58854166666666430, -7.505752307972844761 ) ) ;
#18700=CARTESIAN_POINT ( 'NONE',  ( 0.04044903254992426173, 13.86756916759064318, -30.02300923189239867 ) ) ;
#18722=CARTESIAN_POINT ( 'NONE',  ( 7.025853678916403666, 34.63579833425730925, -26.06988505166735237 ) ) ;
#18729=CARTESIAN_POINT ( 'NONE',  ( -28.02196122052058413, 44.65065999907601935, -7.468012846824272799 ) ) ;
#18732=CARTESIAN_POINT ( 'NONE',  ( 26.07999730980477437, 20.02083333333332860, -6.988114217768290004 ) ) ;
#18734=CARTESIAN_POINT ( 'NONE',  ( 28.01184896238304134, 23.74479166666666430, 7.505752307972846538 ) ) ;
#18738=CARTESIAN_POINT ( 'NONE',  ( -30.02300923189239867, 37.07069416759063785, -0.04044903254991731589 ) ) ;
#18740=CARTESIAN_POINT ( 'NONE',  ( -20.50609665440969209, 55.82812499999999289, 20.50609665441005092 ) ) ;
#18750=CARTESIAN_POINT ( 'NONE',  ( 20.50609665441005092, 20.59374999999999645, 20.50609665440969209 ) ) ;
#18761=CARTESIAN_POINT ( 'NONE',  ( 27.95245687107222921, 61.41406250000000711, -2.463307335887066074E-13 ) ) ;
#18765=CARTESIAN_POINT ( 'NONE',  ( -13.97622843553632777, 36.20572916666665719, -24.20753774853731599 ) ) ;
#18766=CARTESIAN_POINT ( 'NONE',  ( 25.98046417659858420, 32.20090250092397355, 15.04653450569292872 ) ) ;
#18767=CARTESIAN_POINT ( 'NONE',  ( 7.543491769121922985, 19.44232666574268364, 28.00173670424535644 ) ) ;
#18771=CARTESIAN_POINT ( 'NONE',  ( -24.22776226481266448, 44.79388916574269075, -13.94119854578892514 ) ) ;
#18777=CARTESIAN_POINT ( 'NONE',  ( 19.11951029504763611, 52.10975666759065206, -19.06425588902591173 ) ) ;
#18781=CARTESIAN_POINT ( 'NONE',  ( -30.02300923189239512, 28.75781249999999645, 2.654126918244515359E-13 ) ) ;
#18786=CARTESIAN_POINT ( 'NONE',  ( 15.01150461594643204, 48.23697916666665719, 26.00068869287340334 ) ) ;
#18793=CARTESIAN_POINT ( 'NONE',  ( -26.02091320914878025, 58.54388916574269075, -14.97647472619899389 ) ) ;
#18797=CARTESIAN_POINT ( 'NONE',  ( 19.09188309203694800, 61.84374999999998579, 19.09188309203660694 ) ) ;
#18800=CARTESIAN_POINT ( 'NONE',  ( 13.97622843553589966, 29.90364583333332504, -24.20753774853756113 ) ) ;
#18805=CARTESIAN_POINT ( 'NONE',  ( -19.11951029504763611, 57.26600666759063785, 19.06425588902592239 ) ) ;
#18818=CARTESIAN_POINT ( 'NONE',  ( -24.22776226481240514, 19.59673583425730925, 13.94119854578937812 ) ) ;
#18824=CARTESIAN_POINT ( 'NONE',  ( 7.505752307973351023, 55.25520833333333570, 28.01184896238290278 ) ) ;
#18828=CARTESIAN_POINT ( 'NONE',  ( 7.505752307972854531, 19.44791666666666075, -28.01184896238303423 ) ) ;
#18833=CARTESIAN_POINT ( 'NONE',  ( -26.02091320914878025, 34.48138916574268364, -14.97647472619899389 ) ) ;
#18835=CARTESIAN_POINT ( 'NONE',  ( 15.01150461594596486, 47.09114583333332860, -26.00068869287367690 ) ) ;
#18839=CARTESIAN_POINT ( 'NONE',  ( -0.04044903255042732459, 59.11680583240937636, -27.95245687107223986 ) ) ;
#18845=CARTESIAN_POINT ( 'NONE',  ( 13.97622843553589966, 26.46614583333332504, -24.20753774853756113 ) ) ;
#18852=CARTESIAN_POINT ( 'NONE',  ( 27.95245687107223276, 25.60118083240935860, -0.04044903255042905932 ) ) ;
#18855=CARTESIAN_POINT ( 'NONE',  ( -19.09188309203660694, 52.39062499999999289, 19.09188309203694800 ) ) ;
#18860=CARTESIAN_POINT ( 'NONE',  ( -7.505752307972844761, 17.72916666666666430, 28.01184896238304134 ) ) ;
#18861=CARTESIAN_POINT ( 'NONE',  ( -20.47846945139902175, 13.43788166759064140, -20.53372385742072481 ) ) ;
#18870=SHAPE_REPRESENTATION_RELATIONSHIP ( 'NONE' , 'NONE' ,  #8075, #18554 ) ;
#18881=CARTESIAN_POINT ( 'NONE',  ( -6.950374756619716266, 37.78684000092396644, -26.09010956794232428 ) ) ;
#18891=CARTESIAN_POINT ( 'NONE',  ( -28.02196122052058413, 51.52565999907602645, -7.468012846824272799 ) ) ;
#18895=CARTESIAN_POINT ( 'NONE',  ( 6.988114217767829928, 16.01041666666666075, -26.07999730980489872 ) ) ;
#18898=CARTESIAN_POINT ( 'NONE',  ( -20.50609665440969209, 31.76562499999999289, 20.50609665441005092 ) ) ;
#18902=CARTESIAN_POINT ( 'NONE',  ( 26.02091320914851025, 38.50298583425730925, -14.97647472619946463 ) ) ;
#18904=CARTESIAN_POINT ( 'NONE',  ( -15.01150461594642138, 53.39322916666665009, -26.00068869287340334 ) ) ;
#18915=CARTESIAN_POINT ( 'NONE',  ( 28.01184896238290278, 20.02083333333332860, -7.505752307973347470 ) ) ;
#18927=CARTESIAN_POINT ( 'NONE',  ( -13.97622843553632421, 63.70572916666667140, -24.20753774853731599 ) ) ;
#18933=CARTESIAN_POINT ( 'NONE',  ( -24.20753774853730889, 52.53385416666666430, 13.97622843553634020 ) ) ;
#18934=CARTESIAN_POINT ( 'NONE',  ( -14.97647472619946285, 34.20611083425730925, -26.02091320914851025 ) ) ;
#18936=CARTESIAN_POINT ( 'NONE',  ( -20.53372385742107653, 20.87461833240935505, -20.47846945139867003 ) ) ;
#18940=CARTESIAN_POINT ( 'NONE',  ( 0.04044903255044120238, 50.52305583240934794, 27.95245687107223276 ) ) ;
#18946=CARTESIAN_POINT ( 'NONE',  ( 6.950374756619721595, 53.25559000092396644, 26.09010956794232428 ) ) ;
#18950=CARTESIAN_POINT ( 'NONE',  ( -28.01184896238304134, 22.02604166666666430, -7.505752307972844761 ) ) ;
#18954=CARTESIAN_POINT ( 'NONE',  ( 20.50609665440969565, 50.67187500000000000, -20.50609665441004736 ) ) ;
#18961=CARTESIAN_POINT ( 'NONE',  ( 27.95245687107223276, 18.72618083240936215, -0.04044903255042905932 ) ) ;
#18968=CARTESIAN_POINT ( 'NONE',  ( -26.07999730980477437, 28.61458333333333215, 6.988114217768305103 ) ) ;
#18973=CARTESIAN_POINT ( 'NONE',  ( -26.09010956794232428, 60.98996500092398065, 6.950374756619732253 ) ) ;
#18986=CARTESIAN_POINT ( 'NONE',  ( 19.11951029504763611, 28.04725666759063429, -19.06425588902591173 ) ) ;
#18991=CARTESIAN_POINT ( 'NONE',  ( 26.00068869287340334, 50.81510416666667140, -15.01150461594642316 ) ) ;
#18995=CARTESIAN_POINT ( 'NONE',  ( -20.50609665441004736, 22.31250000000000000, -20.50609665440969565 ) ) ;
#19001=CARTESIAN_POINT ( 'NONE',  ( -0.04044903255044120238, 38.49180583240935505, -30.02300923189239867 ) ) ;
#19003=CARTESIAN_POINT ( 'NONE',  ( 15.01150461594643382, 48.23697916666665009, 26.00068869287340334 ) ) ;
#19006=CARTESIAN_POINT ( 'NONE',  ( -26.06988505166722803, 61.55170166574269786, 7.025853678916877953 ) ) ;
#19013=CARTESIAN_POINT ( 'NONE',  ( 27.95245687107223276, 23.60156250000000000, -2.463307335887066074E-13 ) ) ;
#19023=CARTESIAN_POINT ( 'NONE',  ( -27.95245687107223986, 27.31993083240935505, 0.04044903255043252877 ) ) ;
#19025=CARTESIAN_POINT ( 'NONE',  ( -6.988114217768288228, 50.09895833333332860, -26.07999730980477437 ) ) ;
#19031=CARTESIAN_POINT ( 'NONE',  ( 26.00068869287367335, 27.32552083333332860, 15.01150461594596308 ) ) ;
#19032=CARTESIAN_POINT ( 'NONE',  ( -26.02091320914849959, 19.59673583425730925, 14.97647472619947528 ) ) ;
#19051=CARTESIAN_POINT ( 'NONE',  ( 7.025853678916403666, 38.07329833425730925, -26.06988505166735237 ) ) ;
#19058=CARTESIAN_POINT ( 'NONE',  ( 20.47846945139867003, 59.54649333240936215, -20.53372385742107653 ) ) ;
#19061=CARTESIAN_POINT ( 'NONE',  ( -26.07999730980477437, 25.17708333333332860, 6.988114217768305103 ) ) ;
#19065=CARTESIAN_POINT ( 'NONE',  ( 20.50609665440969565, 33.48437500000000000, -20.50609665441004736 ) ) ;
#19068=CARTESIAN_POINT ( 'NONE',  ( 7.468012846824777284, 53.25559000092396644, 28.02196122052045268 ) ) ;
#19070=CARTESIAN_POINT ( 'NONE',  ( 28.01184896238290278, 50.95833333333332860, -7.505752307973347470 ) ) ;
#19091=CARTESIAN_POINT ( 'NONE',  ( -19.09188309203660694, 66.14062500000000000, 19.09188309203694800 ) ) ;
#19096=CARTESIAN_POINT ( 'NONE',  ( 19.09188309203694800, 51.53124999999999289, 19.09188309203660694 ) ) ;
#19097=CARTESIAN_POINT ( 'NONE',  ( -20.47846945139902175, 40.93788166759063785, -20.53372385742072481 ) ) ;
#19098=CARTESIAN_POINT ( 'NONE',  ( -15.04653450569338524, 27.89284749907601935, -25.98046417659831775 ) ) ;
#19101=CARTESIAN_POINT ( 'NONE',  ( 26.09010956794244507, 53.24440999907603356, 6.950374756619249084 ) ) ;
#19108=CARTESIAN_POINT ( 'NONE',  ( -7.025853678916393008, 53.54204833425730925, 26.06988505166735592 ) ) ;
#19112=CARTESIAN_POINT ( 'NONE',  ( 15.01150461594643204, 24.17447916666666785, 26.00068869287340334 ) ) ;
#19117=CARTESIAN_POINT ( 'NONE',  ( 15.01150461594643204, 61.98697916666665009, 26.00068869287340334 ) ) ;
#19124=CARTESIAN_POINT ( 'NONE',  ( 13.94119854578893580, 14.71576416574268720, -24.22776226481265383 ) ) ;
#19131=CARTESIAN_POINT ( 'NONE',  ( -27.95245687107222921, 39.07031249999997868, 2.498001805406602216E-13 ) ) ;
#19137=CARTESIAN_POINT ( 'NONE',  ( 7.025853678916403666, 62.13579833425730925, -26.06988505166735237 ) ) ;
#19139=CARTESIAN_POINT ( 'NONE',  ( -26.00068869287340334, 52.53385416666666430, 15.01150461594643382 ) ) ;
#19150=CARTESIAN_POINT ( 'NONE',  ( 13.94119854578937812, 25.61236083425731636, 24.22776226481240514 ) ) ;
#19155=CARTESIAN_POINT ( 'NONE',  ( -28.01184896238304134, 52.96354166666666430, -7.505752307972844761 ) ) ;
#19159=CARTESIAN_POINT ( 'NONE',  ( 2.740863092043355209E-13, 34.77343750000000000, 30.02300923189239512 ) ) ;
#19167=CARTESIAN_POINT ( 'NONE',  ( 30.02300923189239867, 42.78868083240935505, -0.04044903255044467877 ) ) ;
#19169=CARTESIAN_POINT ( 'NONE',  ( 2.740863092043355209E-13, 48.52343749999999289, 30.02300923189239867 ) ) ;
#19172=CARTESIAN_POINT ( 'NONE',  ( -2.428612866367529427E-13, 15.86718749999999645, -27.95245687107222921 ) ) ;
#19178=CARTESIAN_POINT ( 'NONE',  ( -24.20753774853730889, 18.15885416666666075, 13.97622843553634020 ) ) ;
#19184=CARTESIAN_POINT ( 'NONE',  ( -7.025853678916861966, 28.03607666574268364, -26.06988505166722803 ) ) ;
#19188=CARTESIAN_POINT ( 'NONE',  ( 2.584737979205441561E-13, 51.96093750000000000, 27.95245687107222921 ) ) ;
#19192=CARTESIAN_POINT ( 'NONE',  ( -28.01184896238304134, 22.02604166666666430, -7.505752307972844761 ) ) ;
#19193=CARTESIAN_POINT ( 'NONE',  ( 7.468012846824777284, 25.75559000092397710, 28.02196122052045268 ) ) ;
#19201=CARTESIAN_POINT ( 'NONE',  ( 7.543491769121427382, 51.82329833425730925, -28.00173670424548433 ) ) ;
#19208=CARTESIAN_POINT ( 'NONE',  ( 13.94119854578893580, 38.77826416574269075, -24.22776226481265383 ) ) ;
#19216=CARTESIAN_POINT ( 'NONE',  ( 19.11951029504763611, 41.79725666759063785, -19.06425588902591173 ) ) ;
#19224=CARTESIAN_POINT ( 'NONE',  ( -14.97647472619899389, 57.68451416574269075, 26.02091320914878025 ) ) ;
#19227=CARTESIAN_POINT ( 'NONE',  ( 26.07999730980490227, 30.61979166666666075, 6.988114217767821046 ) ) ;
#19230=CARTESIAN_POINT ( 'NONE',  ( 30.02300923189239512, 30.47656250000000355, -2.619432448724977703E-13 ) ) ;
#19231=DIRECTION ( 'NONE',  ( -0.7071067811865526798, 0.000000000000000000, -0.7071067811865423547 ) ) ;
#19233=CARTESIAN_POINT ( 'NONE',  ( -0.04044903254990864921, 46.52381916759065206, 30.02300923189239867 ) ) ;
#19235=CARTESIAN_POINT ( 'NONE',  ( 26.00068869287340334, 57.69010416666667140, -15.01150461594642316 ) ) ;
#19253=CARTESIAN_POINT ( 'NONE',  ( 26.07999730980477437, 64.70833333333334281, -6.988114217768290004 ) ) ;
#19258=CARTESIAN_POINT ( 'NONE',  ( 27.95245687107223276, 47.66406249999999289, -2.463307335887066074E-13 ) ) ;
#19259=CARTESIAN_POINT ( 'NONE',  ( -20.47846945139902175, 37.50038166759063074, -20.53372385742072481 ) ) ;
#19260=CARTESIAN_POINT ( 'NONE',  ( -30.02300923189239867, 27.31993083240935505, 0.04044903255044988294 ) ) ;
#19264=CARTESIAN_POINT ( 'NONE',  ( 19.06425588902558133, 59.54649333240936215, -19.11951029504797006 ) ) ;
#19271=CARTESIAN_POINT ( 'NONE',  ( 7.025853678916403666, 51.82329833425730925, -26.06988505166735237 ) ) ;
#19275=CARTESIAN_POINT ( 'NONE',  ( 7.505752307972854531, 26.32291666666666075, -28.01184896238303423 ) ) ;
#19279=CARTESIAN_POINT ( 'NONE',  ( 30.02300923189239512, 61.41406250000000711, -2.619432448724977703E-13 ) ) ;
#19285=CARTESIAN_POINT ( 'NONE',  ( -7.468012846824272799, 67.85378499907602645, 28.02196122052058413 ) ) ;
#19293=CARTESIAN_POINT ( 'NONE',  ( 19.09188309203694800, 44.65624999999999289, 19.09188309203660694 ) ) ;
#19299=CARTESIAN_POINT ( 'NONE',  ( -19.11951029504763611, 64.14100666759063074, 19.06425588902592239 ) ) ;
#19300=CARTESIAN_POINT ( 'NONE',  ( -26.00068869287368756, 53.10677083333331439, -15.01150461594595775 ) ) ;
#19314=CARTESIAN_POINT ( 'NONE',  ( -19.06425588902591173, 27.18788166759063785, -19.11951029504763611 ) ) ;
#19319=CARTESIAN_POINT ( 'NONE',  ( -15.01150461594642138, 49.95572916666665009, -26.00068869287340334 ) ) ;
#19323=CARTESIAN_POINT ( 'NONE',  ( -26.00068869287368756, 29.04427083333332504, -15.01150461594595775 ) ) ;
#19328=CARTESIAN_POINT ( 'NONE',  ( 0.04044903255045854962, 47.08555583240935505, 30.02300923189239867 ) ) ;
#19330=CARTESIAN_POINT ( 'NONE',  ( 7.505752307972854531, 50.38541666666666430, -28.01184896238303423 ) ) ;
#19333=CARTESIAN_POINT ( 'NONE',  ( 27.95245687107222921, 13.28906249999999289, -2.463307335887066074E-13 ) ) ;
#19341=CARTESIAN_POINT ( 'NONE',  ( -24.20753774853756823, 18.73177083333332504, -13.97622843553588723 ) ) ;
#19349=CARTESIAN_POINT ( 'NONE',  ( -28.02196122052058413, 27.46315999907601935, -7.468012846824272799 ) ) ;
#19351=CARTESIAN_POINT ( 'NONE',  ( 7.025853678916867295, 26.31732666574268364, 26.06988505166722803 ) ) ;
#19355=CARTESIAN_POINT ( 'NONE',  ( -27.95245687107222921, 56.25781249999997868, 2.498001805406602216E-13 ) ) ;
#19360=CARTESIAN_POINT ( 'NONE',  ( -28.01184896238290278, 25.17708333333332860, 7.505752307973363457 ) ) ;
#19361=CARTESIAN_POINT ( 'NONE',  ( -30.02300923189239867, 23.32069416759064140, -0.04044903254991731589 ) ) ;
#19371=CARTESIAN_POINT ( 'NONE',  ( 7.543491769121427382, 55.26079833425730214, -28.00173670424548433 ) ) ;
#19376=CARTESIAN_POINT ( 'NONE',  ( 26.06988505166722803, 42.64545166574268364, -7.025853678916862854 ) ) ;
#19382=CARTESIAN_POINT ( 'NONE',  ( 13.94119854578937812, 39.36236083425731636, 24.22776226481240514 ) ) ;
#19390=CARTESIAN_POINT ( 'NONE',  ( -14.97647472619899389, 54.24701416574269075, 26.02091320914878025 ) ) ;
#19394=CARTESIAN_POINT ( 'NONE',  ( 19.09188309203694800, 24.03124999999999645, 19.09188309203660694 ) ) ;
#19396=CARTESIAN_POINT ( 'NONE',  ( -20.50609665441004736, 29.18749999999999645, -20.50609665440969565 ) ) ;
#19399=CARTESIAN_POINT ( 'NONE',  ( 7.468012846824777284, 49.81809000092397355, 28.02196122052045268 ) ) ;
#19402=CARTESIAN_POINT ( 'NONE',  ( 28.01184896238304134, 58.11979166666665719, 7.505752307972846538 ) ) ;
#19408=CLOSED_SHELL ( 'NONE', ( #2093, #3381, #21216, #8304 ) ) ;
#19421=CARTESIAN_POINT ( 'NONE',  ( -13.94119854578936923, 10.14361083425730925, -24.22776226481241224 ) ) ;
#19426=CARTESIAN_POINT ( 'NONE',  ( -26.07999730980477437, 49.23958333333332860, 6.988114217768305103 ) ) ;
#19427=CARTESIAN_POINT ( 'NONE',  ( -25.98046417659859486, 37.35715250092397355, -15.04653450569291628 ) ) ;
#19428=CARTESIAN_POINT ( 'NONE',  ( 28.02196122052058413, 29.18190999907601579, 7.468012846824272799 ) ) ;
#19432=CARTESIAN_POINT ( 'NONE',  ( -26.06988505166722803, 58.11420166574269075, 7.025853678916877953 ) ) ;
#19444=CARTESIAN_POINT ( 'NONE',  ( -7.505752307973343918, 36.34895833333333570, -28.01184896238290989 ) ) ;
#19448=CARTESIAN_POINT ( 'NONE',  ( -7.505752307973343918, 53.53645833333332860, -28.01184896238290989 ) ) ;
#19455=CARTESIAN_POINT ( 'NONE',  ( 6.950374756619257965, 14.57253499907601935, -26.09010956794244507 ) ) ;
#19463=CARTESIAN_POINT ( 'NONE',  ( -24.20753774853730889, 38.78385416666665719, 13.97622843553633842 ) ) ;
#19469=CARTESIAN_POINT ( 'NONE',  ( 26.02091320914851025, 14.44048583425730925, -14.97647472619946463 ) ) ;
#19470=CARTESIAN_POINT ( 'NONE',  ( -7.505752307973343918, 56.97395833333333570, -28.01184896238290989 ) ) ;
#19481=CARTESIAN_POINT ( 'NONE',  ( -19.11951029504763611, 22.89100666759064495, 19.06425588902592239 ) ) ;
#19486=CARTESIAN_POINT ( 'NONE',  ( -28.01184896238290278, 56.11458333333332860, 7.505752307973363457 ) ) ;
#19490=CARTESIAN_POINT ( 'NONE',  ( 7.505752307972854531, 29.76041666666666430, -28.01184896238303423 ) ) ;
#19496=CARTESIAN_POINT ( 'NONE',  ( -25.98046417659831420, 40.78347249907601935, 15.04653450569339945 ) ) ;
#19498=CARTESIAN_POINT ( 'NONE',  ( 30.02300923189239867, 57.97656249999998579, -2.619432448724978208E-13 ) ) ;
#19502=CARTESIAN_POINT ( 'NONE',  ( 6.988114217768294445, 14.00520833333333215, 26.07999730980477437 ) ) ;
#19509=CARTESIAN_POINT ( 'NONE',  ( -26.07999730980477437, 32.05208333333332860, 6.988114217768305103 ) ) ;
#19513=CARTESIAN_POINT ( 'NONE',  ( 20.53372385742108008, 29.46836833240935505, 20.47846945139866648 ) ) ;
#19515=CARTESIAN_POINT ( 'NONE',  ( 6.950374756619257965, 31.76003499907602290, -26.09010956794244507 ) ) ;
#19519=CARTESIAN_POINT ( 'NONE',  ( 27.95245687107222921, 54.53906249999998579, -2.463307335887066074E-13 ) ) ;
#19524=CARTESIAN_POINT ( 'NONE',  ( 20.50609665441005092, 24.03124999999999645, 20.50609665440969209 ) ) ;
#19525=CARTESIAN_POINT ( 'NONE',  ( -14.97647472619946285, 23.89361083425731280, -26.02091320914851025 ) ) ;
#19535=CARTESIAN_POINT ( 'NONE',  ( 20.53372385742072481, 55.54725666759064495, -20.47846945139902175 ) ) ;
#19538=CARTESIAN_POINT ( 'NONE',  ( -7.505752307972844761, 34.91666666666666430, 28.01184896238304134 ) ) ;
#19543=CARTESIAN_POINT ( 'NONE',  ( 0.04044903255044120238, 47.08555583240935505, 27.95245687107223276 ) ) ;
#19549=CARTESIAN_POINT ( 'NONE',  ( -24.18731323226248264, 37.35715250092397355, -14.01125832528284931 ) ) ;
#19557=CARTESIAN_POINT ( 'NONE',  ( -15.04653450569338524, 51.95534749907602645, -25.98046417659831775 ) ) ;
#19561=CARTESIAN_POINT ( 'NONE',  ( 19.09188309203694800, 27.46875000000000000, 19.09188309203660694 ) ) ;
#19564=CARTESIAN_POINT ( 'NONE',  ( 26.00068869287367335, 27.32552083333332860, 15.01150461594596308 ) ) ;
#19567=CARTESIAN_POINT ( 'NONE',  ( -7.543491769121417612, 46.66704833425730925, 28.00173670424549499 ) ) ;
#19570=CARTESIAN_POINT ( 'NONE',  ( 26.00068869287340334, 61.12760416666665719, -15.01150461594642316 ) ) ;
#19588=CARTESIAN_POINT ( 'NONE',  ( 19.11951029504763611, 10.85975666759064318, -19.06425588902591173 ) ) ;
#19593=CARTESIAN_POINT ( 'NONE',  ( -27.95245687107223276, 49.38281249999999289, 2.498001805406602216E-13 ) ) ;
#19594=CARTESIAN_POINT ( 'NONE',  ( 7.468012846824777284, 39.50559000092398065, 28.02196122052045268 ) ) ;
#19595=CARTESIAN_POINT ( 'NONE',  ( -7.543491769121917656, 31.47357666574268364, -28.00173670424536354 ) ) ;
#19599=CARTESIAN_POINT ( 'NONE',  ( 19.06425588902558133, 56.10899333240935505, -19.11951029504797006 ) ) ;
#19607=CARTESIAN_POINT ( 'NONE',  ( -15.01150461594595775, 38.49739583333332860, 26.00068869287368756 ) ) ;
#19612=CARTESIAN_POINT ( 'NONE',  ( -26.00068869287340334, 59.40885416666666430, 15.01150461594643382 ) ) ;
#19619=CARTESIAN_POINT ( 'NONE',  ( -7.025853678916861966, 14.28607666574268720, -26.06988505166722803 ) ) ;
#19628=CARTESIAN_POINT ( 'NONE',  ( -6.988114217767819270, 41.79166666666666430, 26.07999730980490583 ) ) ;
#19633=CARTESIAN_POINT ( 'NONE',  ( -20.47846945139902175, 10.00038166759064140, -20.53372385742072481 ) ) ;
#19635=CARTESIAN_POINT ( 'NONE',  ( -28.01184896238290278, 52.67708333333333570, 7.505752307973363457 ) ) ;
#19647=CARTESIAN_POINT ( 'NONE',  ( -13.94119854578936923, 30.76861083425731280, -24.22776226481241224 ) ) ;
#19652=CARTESIAN_POINT ( 'NONE',  ( -28.01184896238304134, 56.40104166666666430, -7.505752307972844761 ) ) ;
#19656=CARTESIAN_POINT ( 'NONE',  ( 28.01184896238290278, 33.77083333333333570, -7.505752307973347470 ) ) ;
#19661=CARTESIAN_POINT ( 'NONE',  ( -0.04044903255044120238, 45.36680583240934794, -30.02300923189239867 ) ) ;
#19663=CARTESIAN_POINT ( 'NONE',  ( 15.01150461594596486, 60.84114583333332860, -26.00068869287367690 ) ) ;
#19667=CARTESIAN_POINT ( 'NONE',  ( 13.97622843553633665, 13.86197916666666430, 24.20753774853730889 ) ) ;
#19673=CARTESIAN_POINT ( 'NONE',  ( -19.09188309203694445, 36.06250000000000000, -19.09188309203661049 ) ) ;
#19678=CARTESIAN_POINT ( 'NONE',  ( -20.53372385742107653, 24.31211833240934794, -20.47846945139867003 ) ) ;
#19680=CARTESIAN_POINT ( 'NONE',  ( 7.025853678916867295, 33.19232666574268364, 26.06988505166722803 ) ) ;
#19684=CARTESIAN_POINT ( 'NONE',  ( -13.94119854578936923, 10.14361083425730925, -24.22776226481241224 ) ) ;
#19689=CARTESIAN_POINT ( 'NONE',  ( 20.50609665441005092, 20.59374999999999645, 20.50609665440969209 ) ) ;
#19690=CARTESIAN_POINT ( 'NONE',  ( 15.04653450569292872, 27.90402750092397355, -25.98046417659857710 ) ) ;
#19700=CARTESIAN_POINT ( 'NONE',  ( -7.543491769121417612, 53.54204833425730925, 28.00173670424549499 ) ) ;
#19703=CARTESIAN_POINT ( 'NONE',  ( -7.505752307973343918, 29.47395833333332860, -28.01184896238290989 ) ) ;
#19707=CARTESIAN_POINT ( 'NONE',  ( 24.22776226481265383, 39.63763916574268364, 13.94119854578893580 ) ) ;
#19713=CARTESIAN_POINT ( 'NONE',  ( 24.22776226481241224, 52.25298583425730925, -13.94119854578936923 ) ) ;
#19720=CARTESIAN_POINT ( 'NONE',  ( 20.47846945139867003, 66.42149333240935505, -20.53372385742107653 ) ) ;
#19725=CARTESIAN_POINT ( 'NONE',  ( -24.20753774853756823, 25.60677083333332149, -13.97622843553588723 ) ) ;
#19730=CARTESIAN_POINT ( 'NONE',  ( 26.00068869287340334, 43.94010416666665719, -15.01150461594642316 ) ) ;
#19733=CARTESIAN_POINT ( 'NONE',  ( -25.98046417659859486, 51.10715250092397355, -15.04653450569291628 ) ) ;
#19735=CARTESIAN_POINT ( 'NONE',  ( 28.01184896238304134, 61.55729166666666430, 7.505752307972846538 ) ) ;
#19753=CARTESIAN_POINT ( 'NONE',  ( 19.11951029504763611, 21.17225666759064850, -19.06425588902591173 ) ) ;
#19758=CARTESIAN_POINT ( 'NONE',  ( 2.584737979205442066E-13, 55.39843749999999289, 27.95245687107223276 ) ) ;
#19759=CARTESIAN_POINT ( 'NONE',  ( 28.02196122052045268, 38.64621500092395934, -7.468012846824774620 ) ) ;
#19760=CARTESIAN_POINT ( 'NONE',  ( 7.468012846824281681, 42.07253499907601935, -28.02196122052058058 ) ) ;
#19763=CARTESIAN_POINT ( 'NONE',  ( 19.11951029504797006, 53.53086833240935505, 19.06425588902558133 ) ) ;
#19771=CARTESIAN_POINT ( 'NONE',  ( 26.00068869287367335, 34.20052083333332860, 15.01150461594596308 ) ) ;
#19776=CARTESIAN_POINT ( 'NONE',  ( -20.50609665441004736, 56.68749999999998579, -20.50609665440969565 ) ) ;
#19783=CARTESIAN_POINT ( 'NONE',  ( -6.950374756619247307, 23.16628499907601579, 26.09010956794245217 ) ) ;
#19792=CARTESIAN_POINT ( 'NONE',  ( -6.988114217767819270, 45.22916666666665719, 26.07999730980490583 ) ) ;
#19797=CARTESIAN_POINT ( 'NONE',  ( 28.02196122052045268, 14.58371500092397710, -7.468012846824774620 ) ) ;
#19798=CARTESIAN_POINT ( 'NONE',  ( 28.01184896238304134, 51.24479166666666430, 7.505752307972846538 ) ) ;
#19810=CARTESIAN_POINT ( 'NONE',  ( -14.01125832528285109, 36.49777750092397355, 24.18731323226248264 ) ) ;
#19815=CARTESIAN_POINT ( 'NONE',  ( -30.02300923189239512, 59.69531250000000711, 2.654126918244515359E-13 ) ) ;
#19819=CARTESIAN_POINT ( 'NONE',  ( 15.01150461594643204, 34.48697916666667140, 26.00068869287340334 ) ) ;
#19824=CARTESIAN_POINT ( 'NONE',  ( -30.02300923189239867, 41.06993083240934794, 0.04044903255044988294 ) ) ;
#19826=CARTESIAN_POINT ( 'NONE',  ( -28.01184896238304134, 56.40104166666666430, -7.505752307972844761 ) ) ;
#19830=CARTESIAN_POINT ( 'NONE',  ( -19.11951029504797006, 68.99961833240934084, -19.06425588902558133 ) ) ;
#19840=CARTESIAN_POINT ( 'NONE',  ( -28.00173670424535644, 23.73920166574268364, 7.543491769121936308 ) ) ;
#19842=CARTESIAN_POINT ( 'NONE',  ( 27.95245687107223276, 35.91368083240935505, -0.04044903255042905932 ) ) ;
#19847=CARTESIAN_POINT ( 'NONE',  ( -6.988114217767819270, 65.85416666666665719, 26.07999730980490583 ) ) ;
#19852=CARTESIAN_POINT ( 'NONE',  ( 20.50609665441005092, 37.78124999999999289, 20.50609665440969209 ) ) ;
#19853=CARTESIAN_POINT ( 'NONE',  ( -20.53372385742071771, 29.76600666759063429, 20.47846945139902530 ) ) ;
#19864=CARTESIAN_POINT ( 'NONE',  ( 7.468012846824777284, 56.69309000092396644, 28.02196122052045268 ) ) ;
#19867=CARTESIAN_POINT ( 'NONE',  ( 26.00068869287367690, 27.32552083333333215, 15.01150461594596486 ) ) ;
#19873=CARTESIAN_POINT ( 'NONE',  ( -24.22776226481266448, 44.79388916574269075, -13.94119854578892514 ) ) ;
#19879=CARTESIAN_POINT ( 'NONE',  ( -7.025853678916393008, 46.66704833425730925, 26.06988505166735592 ) ) ;
#19886=CARTESIAN_POINT ( 'NONE',  ( 25.98046417659831775, 66.56472249907604066, -15.04653450569338879 ) ) ;
#19892=CARTESIAN_POINT ( 'NONE',  ( -13.97622843553588901, 38.49739583333332860, 24.20753774853756823 ) ) ;
#19896=CARTESIAN_POINT ( 'NONE',  ( -2.584737979205441561E-13, 39.92968750000000000, -30.02300923189239512 ) ) ;
#19898=DIRECTION ( 'NONE',  ( -0.7069718413157914938, -0.01953538259431466736, 0.7069718413158002646 ) ) ;
#19900=CARTESIAN_POINT ( 'NONE',  ( 28.00173670424549499, 59.55767333425731636, 7.543491769121417612 ) ) ;
#19901=CARTESIAN_POINT ( 'NONE',  ( -6.950374756619716266, 58.41184000092398065, -26.09010956794232428 ) ) ;
#19903=CARTESIAN_POINT ( 'NONE',  ( -20.50609665440969209, 66.14062500000000000, 20.50609665441005092 ) ) ;
#19925=CARTESIAN_POINT ( 'NONE',  ( 19.06425588902592239, 18.59413166759064140, 19.11951029504763611 ) ) ;
#19930=CARTESIAN_POINT ( 'NONE',  ( 20.47846945139902530, 46.09413166759064495, 20.53372385742071771 ) ) ;
#19931=CARTESIAN_POINT ( 'NONE',  ( -20.53372385742107653, 34.62461833240934794, -20.47846945139867003 ) ) ;
#19934=CARTESIAN_POINT ( 'NONE',  ( -24.22776226481266448, 61.98138916574268364, -13.94119854578892514 ) ) ;
#19937=CARTESIAN_POINT ( 'NONE',  ( 7.505752307972854531, 12.57291666666666252, -28.01184896238303423 ) ) ;
#19945=CARTESIAN_POINT ( 'NONE',  ( -26.00068869287340334, 31.90885416666666430, 15.01150461594643382 ) ) ;
#19960=CARTESIAN_POINT ( 'NONE',  ( -0.04044903255042732459, 28.17930583240935860, -27.95245687107223986 ) ) ;
#19969=CARTESIAN_POINT ( 'NONE',  ( -26.07999730980477437, 49.23958333333332860, 6.988114217768305103 ) ) ;
#19974=CARTESIAN_POINT ( 'NONE',  ( -20.53372385742071771, 16.01600666759064140, 20.47846945139902530 ) ) ;
#19975=CARTESIAN_POINT ( 'NONE',  ( -7.505752307972844761, 58.97916666666666430, 28.01184896238304134 ) ) ;
#19981=CARTESIAN_POINT ( 'NONE',  ( -24.20753774853756823, 66.85677083333332860, -13.97622843553588723 ) ) ;
#19986=CARTESIAN_POINT ( 'NONE',  ( 19.06425588902592239, 32.34413166759064495, 19.11951029504763611 ) ) ;
#19992=CARTESIAN_POINT ( 'NONE',  ( -20.50609665441004736, 60.12500000000000000, -20.50609665440969565 ) ) ;
#19995=CARTESIAN_POINT ( 'NONE',  ( 20.50609665440969565, 40.35937499999999289, -20.50609665441004736 ) ) ;
#20001=CARTESIAN_POINT ( 'NONE',  ( -25.98046417659831420, 54.53347249907601935, 15.04653450569339945 ) ) ;
#20003=CARTESIAN_POINT ( 'NONE',  ( -26.00068869287368756, 56.54427083333332860, -15.01150461594595775 ) ) ;
#20008=CARTESIAN_POINT ( 'NONE',  ( -19.09188309203660694, 21.45312499999999645, 19.09188309203694800 ) ) ;
#20019=CARTESIAN_POINT ( 'NONE',  ( -20.53372385742107653, 27.74961833240935505, -20.47846945139867003 ) ) ;
#20021=CARTESIAN_POINT ( 'NONE',  ( 26.06988505166722803, 39.20795166574269075, -7.025853678916862854 ) ) ;
#20025=CARTESIAN_POINT ( 'NONE',  ( 19.09188309203694800, 61.84374999999998579, 19.09188309203660694 ) ) ;
#20030=CARTESIAN_POINT ( 'NONE',  ( -28.01184896238304134, 35.77604166666666430, -7.505752307972844761 ) ) ;
#20031=CARTESIAN_POINT ( 'NONE',  ( 14.97647472619947351, 29.04986083425730570, 26.02091320914850314 ) ) ;
#20041=CARTESIAN_POINT ( 'NONE',  ( -26.02091320914849959, 64.28423583425730214, 14.97647472619947528 ) ) ;
#20044=CARTESIAN_POINT ( 'NONE',  ( 30.02300923189239867, 30.47656250000000355, -2.619432448724978208E-13 ) ) ;
#20048=CARTESIAN_POINT ( 'NONE',  ( 19.11951029504797006, 39.78086833240934794, 19.06425588902558133 ) ) ;
#20057=CARTESIAN_POINT ( 'NONE',  ( 0.04044903254993986036, 44.80506916759064495, -27.95245687107223986 ) ) ;
#20065=CARTESIAN_POINT ( 'NONE',  ( 25.98046417659831775, 63.12722249907601224, -15.04653450569338879 ) ) ;
#20070=CARTESIAN_POINT ( 'NONE',  ( 6.988114217767829928, 36.63541666666666430, -26.07999730980489872 ) ) ;
#20074=CARTESIAN_POINT ( 'NONE',  ( 15.01150461594596308, 36.77864583333332860, -26.00068869287367335 ) ) ;
#20077=CARTESIAN_POINT ( 'NONE',  ( 20.53372385742072481, 58.98475666759065206, -20.47846945139902175 ) ) ;
#20078=CARTESIAN_POINT ( 'NONE',  ( 26.06988505166735592, 56.12017333425732346, 7.025853678916393896 ) ) ;
#20081=CARTESIAN_POINT ( 'NONE',  ( 20.47846945139867003, 18.29649333240935150, -20.53372385742107653 ) ) ;
#20100=CARTESIAN_POINT ( 'NONE',  ( -14.01125832528285109, 19.31027750092397710, 24.18731323226248264 ) ) ;
#20105=CARTESIAN_POINT ( 'NONE',  ( 28.00173670424549499, 49.24517333425730925, 7.543491769121417612 ) ) ;
#20107=CARTESIAN_POINT ( 'NONE',  ( -0.04044903255044120238, 35.05430583240935505, -30.02300923189239867 ) ) ;
#20111=CARTESIAN_POINT ( 'NONE',  ( 14.01125832528330051, 60.54909749907603356, 24.18731323226221974 ) ) ;
#20114=CARTESIAN_POINT ( 'NONE',  ( 26.00068869287367335, 13.57552083333332682, 15.01150461594596308 ) ) ;
#20122=CARTESIAN_POINT ( 'NONE',  ( 26.00068869287367335, 37.63802083333331439, 15.01150461594596308 ) ) ;
#20130=CARTESIAN_POINT ( 'NONE',  ( 7.505752307972854531, 12.57291666666666252, -28.01184896238303423 ) ) ;
#20135=CARTESIAN_POINT ( 'NONE',  ( 27.95245687107223276, 25.60118083240935860, -0.04044903255042905932 ) ) ;
#20144=CARTESIAN_POINT ( 'NONE',  ( 24.20753774853756113, 51.38802083333332149, 13.97622843553589789 ) ) ;
#20149=CARTESIAN_POINT ( 'NONE',  ( -7.468012846824771955, 17.16184000092397000, -28.02196122052045624 ) ) ;
#20150=CARTESIAN_POINT ( 'NONE',  ( 15.01150461594643204, 65.42447916666667140, 26.00068869287340334 ) ) ;
#20162=CARTESIAN_POINT ( 'NONE',  ( 24.18731323226247554, 28.76340250092398065, 14.01125832528285997 ) ) ;
#20170=CARTESIAN_POINT ( 'NONE',  ( -2.584737979205441561E-13, 43.36718749999999289, -30.02300923189239512 ) ) ;
#20174=CARTESIAN_POINT ( 'NONE',  ( 28.02196122052058413, 56.68190999907602645, 7.468012846824272799 ) ) ;
#20176=CARTESIAN_POINT ( 'NONE',  ( 26.00068869287341045, 54.25260416666666430, -15.01150461594642493 ) ) ;
#20181=CARTESIAN_POINT ( 'NONE',  ( 27.95245687107222921, 23.60156250000000000, -2.463307335887066074E-13 ) ) ;
#20195=CARTESIAN_POINT ( 'NONE',  ( 27.95245687107223276, 39.35118083240935505, -0.04044903255042905932 ) ) ;
#20199=CARTESIAN_POINT ( 'NONE',  ( 2.584737979205441561E-13, 65.71093749999997158, 27.95245687107222921 ) ) ;
#20207=CARTESIAN_POINT ( 'NONE',  ( -20.50609665440969209, 31.76562499999999289, 20.50609665441005092 ) ) ;
#20208=CARTESIAN_POINT ( 'NONE',  ( -14.97647472619946285, 34.20611083425730925, -26.02091320914851025 ) ) ;
#20218=CARTESIAN_POINT ( 'NONE',  ( 7.543491769121427382, 62.13579833425730925, -28.00173670424548433 ) ) ;
#20221=CARTESIAN_POINT ( 'NONE',  ( 15.01150461594643382, 34.48697916666666430, 26.00068869287340334 ) ) ;
#20226=CARTESIAN_POINT ( 'NONE',  ( -0.04044903255042732459, 48.80430583240936215, -27.95245687107223986 ) ) ;
#20233=CARTESIAN_POINT ( 'NONE',  ( -27.95245687107223986, 43.94569416759065206, -0.04044903254993292840 ) ) ;
#20240=CARTESIAN_POINT ( 'NONE',  ( -25.98046417659831420, 68.28347249907602645, 15.04653450569339945 ) ) ;
#20244=CARTESIAN_POINT ( 'NONE',  ( 13.97622843553633665, 34.48697916666667140, 24.20753774853730889 ) ) ;
#20247=CARTESIAN_POINT ( 'NONE',  ( 30.02300923189239512, 37.35156249999997868, -2.619432448724977703E-13 ) ) ;
#20250=CARTESIAN_POINT ( 'NONE',  ( 28.02196122052045268, 55.83371500092398065, -7.468012846824774620 ) ) ;
#20251=CARTESIAN_POINT ( 'NONE',  ( -24.18731323226248264, 57.98215250092397355, -14.01125832528284931 ) ) ;
#20253=CARTESIAN_POINT ( 'NONE',  ( -7.468012846824272799, 16.29128499907601579, 28.02196122052058413 ) ) ;
#20271=CARTESIAN_POINT ( 'NONE',  ( 6.950374756619721595, 22.31809000092397000, 26.09010956794232428 ) ) ;
#20276=CARTESIAN_POINT ( 'NONE',  ( -15.04653450569291984, 50.24777750092398065, 25.98046417659859486 ) ) ;
#20278=CARTESIAN_POINT ( 'NONE',  ( -0.04044903255044120238, 38.49180583240935505, -30.02300923189239867 ) ) ;
#20281=CARTESIAN_POINT ( 'NONE',  ( 0.04044903255044120238, 67.71055583240935505, 27.95245687107223276 ) ) ;
#20291=CARTESIAN_POINT ( 'NONE',  ( -15.01150461594642138, 43.08072916666666430, -26.00068869287340334 ) ) ;
#20299=CARTESIAN_POINT ( 'NONE',  ( 2.740863092043355209E-13, 14.14843749999999467, 30.02300923189239867 ) ) ;
#20303=CARTESIAN_POINT ( 'NONE',  ( 7.025853678916867295, 26.31732666574268364, 26.06988505166722803 ) ) ;
#20312=CARTESIAN_POINT ( 'NONE',  ( 6.988114217767829928, 46.94791666666666430, -26.07999730980489872 ) ) ;
#20317=CARTESIAN_POINT ( 'NONE',  ( 24.20753774853731244, 30.19010416666665719, -13.97622843553633132 ) ) ;
#20319=CARTESIAN_POINT ( 'NONE',  ( 28.00173670424549499, 25.18267333425730214, 7.543491769121417612 ) ) ;
#20320=CARTESIAN_POINT ( 'NONE',  ( -7.505752307973343918, 60.41145833333332149, -28.01184896238290989 ) ) ;
#20330=CARTESIAN_POINT ( 'NONE',  ( -19.06425588902591173, 34.06288166759063785, -19.11951029504763611 ) ) ;
#20334=CARTESIAN_POINT ( 'NONE',  ( -20.50609665441004736, 15.43749999999999645, -20.50609665440969565 ) ) ;
#20338=CARTESIAN_POINT ( 'NONE',  ( -2.584737979205441561E-13, 36.49218750000000000, -30.02300923189239512 ) ) ;
#20343=CARTESIAN_POINT ( 'NONE',  ( 7.468012846824281681, 48.94753499907601935, -28.02196122052058058 ) ) ;
#20345=CARTESIAN_POINT ( 'NONE',  ( 20.50609665441005092, 65.28125000000000000, 20.50609665440969209 ) ) ;
#20350=CARTESIAN_POINT ( 'NONE',  ( -26.07999730980477437, 25.17708333333332860, 6.988114217768305103 ) ) ;
#20365=CARTESIAN_POINT ( 'NONE',  ( -13.94119854578892514, 43.93451416574269075, 24.22776226481266448 ) ) ;
#20369=CARTESIAN_POINT ( 'NONE',  ( -24.20753774853730889, 66.28385416666662877, 13.97622843553633842 ) ) ;
#20374=CARTESIAN_POINT ( 'NONE',  ( 20.50609665441005092, 34.34374999999999289, 20.50609665440969209 ) ) ;
#20375=CARTESIAN_POINT ( 'NONE',  ( 25.98046417659858420, 32.20090250092397355, 15.04653450569292872 ) ) ;
#20385=CARTESIAN_POINT ( 'NONE',  ( -15.01150461594642138, 15.58072916666666607, -26.00068869287340334 ) ) ;
#20388=CARTESIAN_POINT ( 'NONE',  ( -20.50609665441004736, 36.06250000000000000, -20.50609665440969565 ) ) ;
#20394=CARTESIAN_POINT ( 'NONE',  ( -19.11951029504797006, 55.24961833240936926, -19.06425588902558133 ) ) ;
#20399=CARTESIAN_POINT ( 'NONE',  ( 6.988114217768294445, 14.00520833333333215, 26.07999730980477437 ) ) ;
#20406=CARTESIAN_POINT ( 'NONE',  ( 15.04653450569339945, 67.42409749907601224, 25.98046417659831775 ) ) ;
#20411=CARTESIAN_POINT ( 'NONE',  ( 13.97622843553589966, 33.34114583333332860, -24.20753774853756113 ) ) ;
#20414=CARTESIAN_POINT ( 'NONE',  ( -28.01184896238290278, 42.36458333333332860, 7.505752307973363457 ) ) ;
#20417=CARTESIAN_POINT ( 'NONE',  ( 30.02300923189239867, 62.85194416759064495, 0.04044903254992252006 ) ) ;
#20418=CARTESIAN_POINT ( 'NONE',  ( -6.950374756619716266, 61.84934000092397355, -26.09010956794232428 ) ) ;
#20420=EDGE_LOOP ( 'NONE', ( #13585, #6721, #22222, #28211 ) ) ;
#20422=CARTESIAN_POINT ( 'NONE',  ( -26.00068869287340334, 66.28385416666662877, 15.01150461594643382 ) ) ;
#20442=CARTESIAN_POINT ( 'NONE',  ( 24.22776226481241224, 24.75298583425730925, -13.94119854578936923 ) ) ;
#20448=CARTESIAN_POINT ( 'NONE',  ( -28.02196122052045268, 43.80246500092398776, 7.468012846824790607 ) ) ;
#20450=CARTESIAN_POINT ( 'NONE',  ( -7.543491769121917656, 34.91107666574267654, -28.00173670424536354 ) ) ;
#20454=CARTESIAN_POINT ( 'NONE',  ( 27.95245687107223276, 66.85118083240935505, -0.04044903255042905932 ) ) ;
#20463=CARTESIAN_POINT ( 'NONE',  ( 7.505752307973351023, 41.50520833333333570, 28.01184896238290278 ) ) ;
#20479=CARTESIAN_POINT ( 'NONE',  ( -19.11951029504797006, 27.74961833240935505, -19.06425588902558133 ) ) ;
#20487=CARTESIAN_POINT ( 'NONE',  ( -2.428612866367529427E-13, 53.67968750000000000, -27.95245687107222921 ) ) ;
#20491=CARTESIAN_POINT ( 'NONE',  ( -19.09188309203694445, 29.18749999999999645, -19.09188309203661049 ) ) ;
#20493=CARTESIAN_POINT ( 'NONE',  ( 30.02300923189239867, 21.60194416759064495, 0.04044903254992252006 ) ) ;
#20495=CARTESIAN_POINT ( 'NONE',  ( -7.543491769121917656, 14.28607666574268720, -28.00173670424536354 ) ) ;
#20508=CARTESIAN_POINT ( 'NONE',  ( 27.95245687107223986, 45.66444416759065916, 0.04044903254993640479 ) ) ;
#20512=CARTESIAN_POINT ( 'NONE',  ( 20.50609665440969565, 16.29687499999999645, -20.50609665441004736 ) ) ;
#20517=CARTESIAN_POINT ( 'NONE',  ( 20.50609665440969565, 36.92187499999999289, -20.50609665441004736 ) ) ;
#20524=CARTESIAN_POINT ( 'NONE',  ( -25.98046417659831420, 51.09597249907602645, 15.04653450569339945 ) ) ;
#20527=CARTESIAN_POINT ( 'NONE',  ( 26.00068869287341045, 64.56510416666667140, -15.01150461594642493 ) ) ;
#20532=CARTESIAN_POINT ( 'NONE',  ( 6.988114217767829928, 26.32291666666666075, -26.07999730980489872 ) ) ;
#20547=CARTESIAN_POINT ( 'NONE',  ( -26.09010956794232428, 16.30246500092397355, 6.950374756619732253 ) ) ;
#20552=CARTESIAN_POINT ( 'NONE',  ( 2.740863092043355209E-13, 31.33593749999999289, 30.02300923189239512 ) ) ;
#20564=CARTESIAN_POINT ( 'NONE',  ( 30.02300923189239867, 62.85194416759064495, 0.04044903254992252006 ) ) ;
#20567=CARTESIAN_POINT ( 'NONE',  ( -7.505752307972844761, 41.79166666666666430, 28.01184896238304134 ) ) ;
#20573=CARTESIAN_POINT ( 'NONE',  ( 14.01125832528330051, 57.11159749907603356, 24.18731323226221974 ) ) ;
#20578=CARTESIAN_POINT ( 'NONE',  ( -26.07999730980477437, 14.86458333333333037, 6.988114217768305103 ) ) ;
#20586=CARTESIAN_POINT ( 'NONE',  ( -19.06425588902558133, 20.01524333240935505, 19.11951029504797006 ) ) ;
#20591=CARTESIAN_POINT ( 'NONE',  ( -27.95245687107222921, 35.63281249999998579, 2.498001805406602216E-13 ) ) ;
#20594=CARTESIAN_POINT ( 'NONE',  ( 7.505752307973351023, 44.94270833333332860, 28.01184896238290278 ) ) ;
#20597=CARTESIAN_POINT ( 'NONE',  ( 26.02091320914851025, 59.12798583425730925, -14.97647472619946463 ) ) ;
#20598=CARTESIAN_POINT ( 'NONE',  ( -0.04044903254992426173, 60.27381916759065206, 27.95245687107223276 ) ) ;
#20602=CARTESIAN_POINT ( 'NONE',  ( 20.47846945139867003, 14.85899333240935505, -20.53372385742107653 ) ) ;
#20623=CARTESIAN_POINT ( 'NONE',  ( 26.09010956794232428, 28.33371500092397355, -6.950374756619718042 ) ) ;
#20629=CARTESIAN_POINT ( 'NONE',  ( -28.00173670424535644, 47.80170166574269786, 7.543491769121936308 ) ) ;
#20634=CARTESIAN_POINT ( 'NONE',  ( -6.950374756619247307, 60.97878499907603356, 26.09010956794245217 ) ) ;
#20643=CARTESIAN_POINT ( 'NONE',  ( 20.50609665441005092, 44.65624999999999289, 20.50609665440969209 ) ) ;
#20644=CARTESIAN_POINT ( 'NONE',  ( -26.00068869287368756, 63.41927083333333570, -15.01150461594595775 ) ) ;
#20656=CARTESIAN_POINT ( 'NONE',  ( -15.01150461594595775, 14.43489583333332860, 26.00068869287368756 ) ) ;
#20661=CARTESIAN_POINT ( 'NONE',  ( 19.11951029504797006, 32.90586833240934794, 19.06425588902558133 ) ) ;
#20670=CARTESIAN_POINT ( 'NONE',  ( 2.584737979205441561E-13, 48.52343750000000000, 27.95245687107222921 ) ) ;
#20675=CARTESIAN_POINT ( 'NONE',  ( 13.97622843553589966, 33.34114583333332860, -24.20753774853756113 ) ) ;
#20676=CARTESIAN_POINT ( 'NONE',  ( 7.543491769121427382, 24.32329833425730214, -28.00173670424548433 ) ) ;
#20677=CARTESIAN_POINT ( 'NONE',  ( -28.01184896238290278, 66.42708333333332860, 7.505752307973363457 ) ) ;
#20683=CARTESIAN_POINT ( 'NONE',  ( -26.07999730980490583, 66.71354166666665719, -6.988114217767815717 ) ) ;
#20687=CARTESIAN_POINT ( 'NONE',  ( 24.22776226481241224, 45.37798583425732346, -13.94119854578936923 ) ) ;
#20691=CARTESIAN_POINT ( 'NONE',  ( -30.02300923189239512, 15.00781249999999467, 2.654126918244515359E-13 ) ) ;
#20695=CARTESIAN_POINT ( 'NONE',  ( 7.505752307973351023, 41.50520833333333570, 28.01184896238290278 ) ) ;
#20700=CARTESIAN_POINT ( 'NONE',  ( -15.04653450569338524, 55.39284749907604066, -25.98046417659831775 ) ) ;
#20702=CARTESIAN_POINT ( 'NONE',  ( 7.505752307972854531, 64.13541666666667140, -28.01184896238303423 ) ) ;
#20708=CARTESIAN_POINT ( 'NONE',  ( -26.07999730980490583, 22.02604166666666430, -6.988114217767815717 ) ) ;
#20724=CARTESIAN_POINT ( 'NONE',  ( -7.025853678916393008, 12.29204833425730925, 26.06988505166735592 ) ) ;
#20729=CARTESIAN_POINT ( 'NONE',  ( -28.01184896238290278, 42.36458333333332860, 7.505752307973363457 ) ) ;
#20740=CARTESIAN_POINT ( 'NONE',  ( -7.505752307972844761, 14.29166666666666430, 28.01184896238304134 ) ) ;
#20742=CARTESIAN_POINT ( 'NONE',  ( -26.00068869287340334, 42.22135416666666430, 15.01150461594643559 ) ) ;
#20748=CARTESIAN_POINT ( 'NONE',  ( 24.18731323226221974, 56.25222249907602645, -14.01125832528328985 ) ) ;
#20760=CARTESIAN_POINT ( 'NONE',  ( -19.11951029504797006, 20.87461833240935505, -19.06425588902558133 ) ) ;
#20764=CARTESIAN_POINT ( 'NONE',  ( -2.428612866367529427E-13, 43.36718749999999289, -27.95245687107222921 ) ) ;
#20767=CARTESIAN_POINT ( 'NONE',  ( 28.01184896238290278, 47.52083333333332860, -7.505752307973347470 ) ) ;
#20769=CARTESIAN_POINT ( 'NONE',  ( -20.47846945139902175, 65.00038166759063074, -20.53372385742072481 ) ) ;
#20770=CARTESIAN_POINT ( 'NONE',  ( 30.02300923189239867, 18.16444416759064140, 0.04044903254992252006 ) ) ;
#20780=( NAMED_UNIT ( * ) PLANE_ANGLE_UNIT ( ) SI_UNIT ( $, .RADIAN. ) );
#20790=CARTESIAN_POINT ( 'NONE',  ( -27.95245687107223986, 26.75819416759064495, -0.04044903254993292840 ) ) ;
#20797=CARTESIAN_POINT ( 'NONE',  ( 26.02091320914876960, 49.95013916574269786, 14.97647472619900455 ) ) ;
#20801=CARTESIAN_POINT ( 'NONE',  ( -24.20753774853730889, 14.72135416666666607, 13.97622843553633842 ) ) ;
#20804=CARTESIAN_POINT ( 'NONE',  ( 7.505752307972854531, 19.44791666666666075, -28.01184896238303423 ) ) ;
#20810=CARTESIAN_POINT ( 'NONE',  ( 20.50609665440969565, 40.35937499999999289, -20.50609665441004736 ) ) ;
#20811=CARTESIAN_POINT ( 'NONE',  ( 2.740863092043355209E-13, 62.27343749999999289, 30.02300923189239512 ) ) ;
#20820=CARTESIAN_POINT ( 'NONE',  ( -20.50609665441004736, 11.99999999999999645, -20.50609665440969565 ) ) ;
#20826=CARTESIAN_POINT ( 'NONE',  ( 13.94119854578893580, 35.34076416574268364, -24.22776226481265383 ) ) ;
#20833=CARTESIAN_POINT ( 'NONE',  ( -6.988114217768288228, 60.41145833333332149, -26.07999730980477437 ) ) ;
#20837=CARTESIAN_POINT ( 'NONE',  ( 19.09188309203661049, 40.35937499999999289, -19.09188309203694445 ) ) ;
#20838=CARTESIAN_POINT ( 'NONE',  ( -7.468012846824771955, 34.34934000092397355, -28.02196122052045624 ) ) ;
#20839=CARTESIAN_POINT ( 'NONE',  ( -7.543491769121917656, 17.72357666574268720, -28.00173670424536354 ) ) ;
#20848=CARTESIAN_POINT ( 'NONE',  ( -24.22776226481240514, 40.22173583425730925, 13.94119854578937812 ) ) ;
#20852=CARTESIAN_POINT ( 'NONE',  ( 26.00068869287340334, 13.00260416666666430, -15.01150461594642316 ) ) ;
#20856=CARTESIAN_POINT ( 'NONE',  ( 7.505752307973351023, 48.38020833333332860, 28.01184896238290278 ) ) ;
#20861=CARTESIAN_POINT ( 'NONE',  ( -15.04653450569338524, 65.70534749907602645, -25.98046417659831775 ) ) ;
#20866=CARTESIAN_POINT ( 'NONE',  ( -26.07999730980490583, 56.40104166666666430, -6.988114217767815717 ) ) ;
#20869=CARTESIAN_POINT ( 'NONE',  ( -26.07999730980477437, 32.05208333333332860, 6.988114217768305103 ) ) ;
#20876=CARTESIAN_POINT ( 'NONE',  ( -19.11951029504763611, 50.39100666759063785, 19.06425588902592239 ) ) ;
#20886=CARTESIAN_POINT ( 'NONE',  ( 24.22776226481241224, 14.44048583425730925, -13.94119854578936923 ) ) ;
#20890=CARTESIAN_POINT ( 'NONE',  ( 26.00068869287340334, 40.50260416666666430, -15.01150461594642316 ) ) ;
#20901=CARTESIAN_POINT ( 'NONE',  ( 7.543491769121922985, 36.62982666574267654, 28.00173670424535644 ) ) ;
#20903=CARTESIAN_POINT ( 'NONE',  ( -2.584737979205442066E-13, 36.49218749999999289, -30.02300923189239867 ) ) ;
#20907=CARTESIAN_POINT ( 'NONE',  ( 6.950374756619257965, 55.82253499907601935, -26.09010956794244507 ) ) ;
#20922=CARTESIAN_POINT ( 'NONE',  ( -14.01125832528328985, 21.01784749907601579, -24.18731323226223040 ) ) ;
#20928=CARTESIAN_POINT ( 'NONE',  ( 26.07999730980477437, 40.64583333333332860, -6.988114217768290004 ) ) ;
#20932=CARTESIAN_POINT ( 'NONE',  ( -28.01184896238290278, 45.80208333333333570, 7.505752307973363457 ) ) ;
#20934=CARTESIAN_POINT ( 'NONE',  ( -15.01150461594595775, 14.43489583333332682, 26.00068869287368756 ) ) ;
#20935=CARTESIAN_POINT ( 'NONE',  ( -20.47846945139902175, 16.87538166759064140, -20.53372385742072481 ) ) ;
#20941=CARTESIAN_POINT ( 'NONE',  ( -26.00068869287340334, 62.84635416666667851, 15.01150461594643382 ) ) ;
#20945=PRESENTATION_STYLE_ASSIGNMENT (( #15964 ) ) ;
#20955=CARTESIAN_POINT ( 'NONE',  ( -27.95245687107223986, 33.63319416759063785, -0.04044903254993292840 ) ) ;
#20962=CARTESIAN_POINT ( 'NONE',  ( -14.97647472619899389, 47.37201416574269786, 26.02091320914878025 ) ) ;
#20965=CARTESIAN_POINT ( 'NONE',  ( -24.20753774853756823, 15.29427083333332504, -13.97622843553588723 ) ) ;
#20968=CARTESIAN_POINT ( 'NONE',  ( 28.01184896238290278, 23.45833333333333215, -7.505752307973347470 ) ) ;
#20972=CARTESIAN_POINT ( 'NONE',  ( -20.53372385742071771, 43.51600666759065206, 20.47846945139902530 ) ) ;
#20975=CARTESIAN_POINT ( 'NONE',  ( 20.50609665440969565, 47.23437499999999289, -20.50609665441004736 ) ) ;
#20986=CARTESIAN_POINT ( 'NONE',  ( 30.02300923189239867, 20.16406249999999645, -2.619432448724978208E-13 ) ) ;
#20992=CARTESIAN_POINT ( 'NONE',  ( 14.01125832528330051, 36.48659749907601935, 24.18731323226221974 ) ) ;
#20999=CARTESIAN_POINT ( 'NONE',  ( 6.988114217768294445, 62.13020833333334281, 26.07999730980477437 ) ) ;
#21003=CARTESIAN_POINT ( 'NONE',  ( 26.07999730980490227, 37.49479166666666430, 6.988114217767821046 ) ) ;
#21004=CARTESIAN_POINT ( 'NONE',  ( -30.02300923189239867, 26.75819416759064495, -0.04044903254991731589 ) ) ;
#21005=CARTESIAN_POINT ( 'NONE',  ( 7.468012846824281681, 21.44753499907601579, -28.02196122052058058 ) ) ;
#21009=CARTESIAN_POINT ( 'NONE',  ( 26.09010956794244507, 49.80690999907602645, 6.950374756619249084 ) ) ;
#21015=CARTESIAN_POINT ( 'NONE',  ( 14.01125832528286352, 41.65402750092398065, -24.18731323226246843 ) ) ;
#21020=CARTESIAN_POINT ( 'NONE',  ( 7.505752307973351023, 17.44270833333333215, 28.01184896238290278 ) ) ;
#21025=CARTESIAN_POINT ( 'NONE',  ( -28.01184896238290278, 49.23958333333332860, 7.505752307973363457 ) ) ;
#21031=CARTESIAN_POINT ( 'NONE',  ( -25.98046417659831420, 64.84597249907602645, 15.04653450569339945 ) ) ;
#21033=CARTESIAN_POINT ( 'NONE',  ( -20.50609665441004736, 63.56249999999999289, -20.50609665440969565 ) ) ;
#21036=CARTESIAN_POINT ( 'NONE',  ( 24.20753774853756113, 65.13802083333334281, 13.97622843553589789 ) ) ;
#21039=CARTESIAN_POINT ( 'NONE',  ( -26.07999730980477437, 35.48958333333332860, 6.988114217768305103 ) ) ;
#21045=CARTESIAN_POINT ( 'NONE',  ( -24.22776226481240514, 57.40923583425731636, 13.94119854578937812 ) ) ;
#21057=CARTESIAN_POINT ( 'NONE',  ( -24.18731323226248264, 13.29465250092397532, -14.01125832528284931 ) ) ;
#21061=CARTESIAN_POINT ( 'NONE',  ( -28.01184896238290278, 38.92708333333333570, 7.505752307973363457 ) ) ;
#21066=CARTESIAN_POINT ( 'NONE',  ( 15.01150461594596308, 19.59114583333332149, -26.00068869287367335 ) ) ;
#21072=CARTESIAN_POINT ( 'NONE',  ( -15.04653450569338524, 34.76784749907601935, -25.98046417659831775 ) ) ;
#21074=CARTESIAN_POINT ( 'NONE',  ( 30.02300923189239867, 40.78906249999999289, -2.619432448724978208E-13 ) ) ;
#21080=CARTESIAN_POINT ( 'NONE',  ( 24.18731323226221974, 59.68972249907602645, -14.01125832528328985 ) ) ;
#21086=CARTESIAN_POINT ( 'NONE',  ( 27.95245687107223276, 16.72656249999999645, -2.463307335887066074E-13 ) ) ;
#21095=CARTESIAN_POINT ( 'NONE',  ( 0.04044903255044120238, 16.14805583240936215, 27.95245687107223276 ) ) ;
#21099=CARTESIAN_POINT ( 'NONE',  ( 13.97622843553589966, 47.09114583333332860, -24.20753774853756113 ) ) ;
#21103=CARTESIAN_POINT ( 'NONE',  ( -26.02091320914849959, 64.28423583425730214, 14.97647472619947528 ) ) ;
#21104=CARTESIAN_POINT ( 'NONE',  ( -14.97647472619946285, 17.01861083425731280, -26.02091320914851025 ) ) ;
#21124=CARTESIAN_POINT ( 'NONE',  ( 26.06988505166735592, 32.05767333425730214, 7.025853678916393896 ) ) ;
#21132=CARTESIAN_POINT ( 'NONE',  ( -7.543491769121917656, 45.22357666574267654, -28.00173670424536354 ) ) ;
#21137=CARTESIAN_POINT ( 'NONE',  ( 19.09188309203661049, 16.29687499999999645, -19.09188309203694445 ) ) ;
#21140=CARTESIAN_POINT ( 'NONE',  ( 15.01150461594643204, 24.17447916666666785, 26.00068869287340334 ) ) ;
#21144=CARTESIAN_POINT ( 'NONE',  ( 26.02091320914851025, 41.94048583425730925, -14.97647472619946463 ) ) ;
#21146=CARTESIAN_POINT ( 'NONE',  ( -15.01150461594642138, 56.83072916666665009, -26.00068869287340334 ) ) ;
#21156=CARTESIAN_POINT ( 'NONE',  ( -30.02300923189239867, 18.44531249999999645, 2.654126918244514854E-13 ) ) ;
#21162=CARTESIAN_POINT ( 'NONE',  ( -13.94119854578892514, 37.05951416574268364, 24.22776226481266448 ) ) ;
#21169=CARTESIAN_POINT ( 'NONE',  ( -13.97622843553588901, 55.68489583333332860, 24.20753774853756823 ) ) ;
#21174=CARTESIAN_POINT ( 'NONE',  ( 6.988114217768294445, 41.50520833333333570, 26.07999730980477437 ) ) ;
#21175=CARTESIAN_POINT ( 'NONE',  ( 0.04044903254992426173, 34.49256916759064495, -30.02300923189239867 ) ) ;
#21176=CARTESIAN_POINT ( 'NONE',  ( 26.02091320914876960, 15.57513916574268720, 14.97647472619900455 ) ) ;
#21180=CARTESIAN_POINT ( 'NONE',  ( -26.09010956794245217, 44.65065999907601935, -6.950374756619243755 ) ) ;
#21186=CARTESIAN_POINT ( 'NONE',  ( 14.01125832528286352, 38.21652750092398065, -24.18731323226246843 ) ) ;
#21190=CARTESIAN_POINT ( 'NONE',  ( 2.740863092043355209E-13, 21.02343749999999645, 30.02300923189239512 ) ) ;
#21194=CARTESIAN_POINT ( 'NONE',  ( -20.50609665441004736, 53.25000000000000000, -20.50609665440969565 ) ) ;
#21199=CARTESIAN_POINT ( 'NONE',  ( 28.00173670424535644, 59.83295166574269075, -7.543491769121920321 ) ) ;
#21204=CARTESIAN_POINT ( 'NONE',  ( 13.97622843553633842, 58.54947916666666430, 24.20753774853730889 ) ) ;
#21207=CARTESIAN_POINT ( 'NONE',  ( -26.07999730980490583, 35.77604166666666430, -6.988114217767815717 ) ) ;
#21213=CARTESIAN_POINT ( 'NONE',  ( -27.95245687107223986, 57.69569416759065206, -0.04044903254993292840 ) ) ;
#21216=ADVANCED_FACE ( 'NONE', ( #4628 ), #22317, .F. ) ;
#21226=CARTESIAN_POINT ( 'NONE',  ( -13.94119854578936923, 13.58111083425730925, -24.22776226481241224 ) ) ;
#21232=CARTESIAN_POINT ( 'NONE',  ( 15.01150461594643204, 44.79947916666667140, 26.00068869287340334 ) ) ;
#21236=CARTESIAN_POINT ( 'NONE',  ( -26.00068869287340334, 18.15885416666666075, 15.01150461594643382 ) ) ;
#21242=CARTESIAN_POINT ( 'NONE',  ( -25.98046417659831420, 30.47097249907602290, 15.04653450569339945 ) ) ;
#21244=CARTESIAN_POINT ( 'NONE',  ( -15.01150461594642316, 53.39322916666665719, -26.00068869287341045 ) ) ;
#21250=CARTESIAN_POINT ( 'NONE',  ( -13.94119854578892514, 64.55951416574268364, 24.22776226481266448 ) ) ;
#21256=CARTESIAN_POINT ( 'NONE',  ( 19.09188309203661049, 19.73437500000000000, -19.09188309203694445 ) ) ;
#21263=CARTESIAN_POINT ( 'NONE',  ( 0.04044903255044120238, 23.02305583240935860, 27.95245687107223276 ) ) ;
#21269=CARTESIAN_POINT ( 'NONE',  ( 13.97622843553633665, 44.79947916666667140, 24.20753774853730889 ) ) ;
#21273=CARTESIAN_POINT ( 'NONE',  ( 28.01184896238304134, 13.43229166666666607, 7.505752307972846538 ) ) ;
#21274=CARTESIAN_POINT ( 'NONE',  ( -20.53372385742071771, 16.01600666759064140, 20.47846945139902530 ) ) ;
#21286=( NAMED_UNIT ( * ) PLANE_ANGLE_UNIT ( ) SI_UNIT ( $, .RADIAN. ) );
#21297=CARTESIAN_POINT ( 'NONE',  ( -7.025853678916393008, 32.91704833425729504, 26.06988505166735592 ) ) ;
#21304=CARTESIAN_POINT ( 'NONE',  ( 25.98046417659831775, 42.50222249907603356, -15.04653450569338879 ) ) ;
#21307=CARTESIAN_POINT ( 'NONE',  ( -19.09188309203660694, 18.01562499999999645, 19.09188309203694800 ) ) ;
#21309=CARTESIAN_POINT ( 'NONE',  ( -30.02300923189239512, 21.88281249999999645, 2.654126918244515359E-13 ) ) ;
#21313=CARTESIAN_POINT ( 'NONE',  ( -7.543491769121417612, 39.79204833425731636, 28.00173670424549499 ) ) ;
#21315=CARTESIAN_POINT ( 'NONE',  ( 28.01184896238290278, 54.39583333333332860, -7.505752307973347470 ) ) ;
#21324=CARTESIAN_POINT ( 'NONE',  ( 26.00068869287367690, 23.88802083333332504, 15.01150461594596486 ) ) ;
#21329=CARTESIAN_POINT ( 'NONE',  ( -7.025853678916861966, 38.34857666574267654, -26.06988505166722803 ) ) ;
#21336=CARTESIAN_POINT ( 'NONE',  ( 26.07999730980490227, 61.55729166666666430, 6.988114217767821046 ) ) ;
#21340=CARTESIAN_POINT ( 'NONE',  ( 26.07999730980490227, 44.36979166666666430, 6.988114217767821046 ) ) ;
#21341=CARTESIAN_POINT ( 'NONE',  ( 28.02196122052045268, 31.77121500092397000, -7.468012846824774620 ) ) ;
#21342=CARTESIAN_POINT ( 'NONE',  ( -14.97647472619899389, 23.30951416574269075, 26.02091320914878025 ) ) ;
#21347=CARTESIAN_POINT ( 'NONE',  ( -26.06988505166722803, 47.80170166574269786, 7.025853678916877953 ) ) ;
#21353=CARTESIAN_POINT ( 'NONE',  ( 24.18731323226247554, 49.38840250092398776, 14.01125832528285997 ) ) ;
#21357=CARTESIAN_POINT ( 'NONE',  ( -26.00068869287368756, 25.60677083333332149, -15.01150461594595775 ) ) ;
#21361=CARTESIAN_POINT ( 'NONE',  ( 7.505752307972854531, 46.94791666666666430, -28.01184896238303423 ) ) ;
#21366=CARTESIAN_POINT ( 'NONE',  ( -7.543491769121917656, 62.41107666574269075, -28.00173670424536354 ) ) ;
#21371=CARTESIAN_POINT ( 'NONE',  ( -6.988114217768288228, 56.97395833333333570, -26.07999730980477437 ) ) ;
#21374=CARTESIAN_POINT ( 'NONE',  ( 26.07999730980477437, 33.77083333333333570, -6.988114217768290004 ) ) ;
#21379=CARTESIAN_POINT ( 'NONE',  ( -24.18731323226248264, 57.98215250092397355, -14.01125832528284931 ) ) ;
#21390=CARTESIAN_POINT ( 'NONE',  ( -24.22776226481240514, 23.03423583425731280, 13.94119854578937812 ) ) ;
#21395=CARTESIAN_POINT ( 'NONE',  ( -7.505752307973343918, 46.66145833333332860, -28.01184896238290989 ) ) ;
#21399=CARTESIAN_POINT ( 'NONE',  ( 7.505752307973351023, 20.88020833333333215, 28.01184896238290278 ) ) ;
#21406=CARTESIAN_POINT ( 'NONE',  ( -25.98046417659831420, 33.90847249907601935, 15.04653450569339945 ) ) ;
#21408=CARTESIAN_POINT ( 'NONE',  ( 20.50609665441005092, 51.53124999999999289, 20.50609665440969209 ) ) ;
#21414=CARTESIAN_POINT ( 'NONE',  ( -19.11951029504797006, 58.68711833240935505, -19.06425588902558133 ) ) ;
#21421=CARTESIAN_POINT ( 'NONE',  ( 6.988114217767829928, 26.32291666666666075, -26.07999730980489872 ) ) ;
#21429=CARTESIAN_POINT ( 'NONE',  ( -0.04044903255042732459, 28.17930583240935860, -27.95245687107223986 ) ) ;
#21431=CARTESIAN_POINT ( 'NONE',  ( 26.07999730980490227, 58.11979166666665719, 6.988114217767821046 ) ) ;
#21435=CARTESIAN_POINT ( 'NONE',  ( -26.00068869287340334, 18.15885416666666075, 15.01150461594643382 ) ) ;
#21436=CARTESIAN_POINT ( 'NONE',  ( 20.47846945139902530, 11.71913166759064318, 20.53372385742071771 ) ) ;
#21457=CARTESIAN_POINT ( 'NONE',  ( 26.06988505166735592, 35.49517333425730214, 7.025853678916393896 ) ) ;
#21466=CARTESIAN_POINT ( 'NONE',  ( -26.02091320914878025, 55.10638916574269786, -14.97647472619899389 ) ) ;
#21469=CARTESIAN_POINT ( 'NONE',  ( 26.07999730980490227, 13.43229166666666607, 6.988114217767821046 ) ) ;
#21471=CARTESIAN_POINT ( 'NONE',  ( -26.00068869287368756, 32.48177083333332860, -15.01150461594595775 ) ) ;
#21474=CARTESIAN_POINT ( 'NONE',  ( 15.04653450569292872, 38.21652750092398065, -25.98046417659857710 ) ) ;
#21476=CARTESIAN_POINT ( 'NONE',  ( 20.50609665440969565, 54.10937499999999289, -20.50609665441004736 ) ) ;
#21477=CARTESIAN_POINT ( 'NONE',  ( -28.01184896238304134, 66.71354166666665719, -7.505752307972844761 ) ) ;
#21486=CARTESIAN_POINT ( 'NONE',  ( 15.01150461594643382, 17.29947916666666430, 26.00068869287340334 ) ) ;
#21497=CARTESIAN_POINT ( 'NONE',  ( 2.584737979205441561E-13, 58.83593750000000000, 27.95245687107222921 ) ) ;
#21501=CARTESIAN_POINT ( 'NONE',  ( -13.97622843553632777, 43.08072916666666430, -24.20753774853731599 ) ) ;
#21502=CARTESIAN_POINT ( 'NONE',  ( -20.53372385742071771, 33.20350666759063074, 20.47846945139902530 ) ) ;
#21503=CARTESIAN_POINT ( 'NONE',  ( 20.53372385742108008, 22.59336833240935505, 20.47846945139866648 ) ) ;
#21507=CARTESIAN_POINT ( 'NONE',  ( 24.18731323226221974, 49.37722249907602645, -14.01125832528328985 ) ) ;
#21514=CARTESIAN_POINT ( 'NONE',  ( -24.18731323226248264, 47.66965250092398065, -14.01125832528284931 ) ) ;
#21518=CARTESIAN_POINT ( 'NONE',  ( -2.584737979205441561E-13, 26.17968750000000000, -30.02300923189239512 ) ) ;
#21523=CARTESIAN_POINT ( 'NONE',  ( 7.505752307972854531, 50.38541666666666430, -28.01184896238303423 ) ) ;
#21529=CARTESIAN_POINT ( 'NONE',  ( 14.97647472619900455, 66.27826416574268364, -26.02091320914876960 ) ) ;
#21536=CARTESIAN_POINT ( 'NONE',  ( 24.20753774853756113, 34.20052083333332860, 13.97622843553589789 ) ) ;
#21541=CARTESIAN_POINT ( 'NONE',  ( -14.01125832528285109, 53.68527750092398065, 24.18731323226248264 ) ) ;
#21558=CARTESIAN_POINT ( 'NONE',  ( -24.18731323226248264, 23.60715250092398421, -14.01125832528284931 ) ) ;
#21563=CARTESIAN_POINT ( 'NONE',  ( 20.50609665441005092, 54.96875000000000000, 20.50609665440969209 ) ) ;
#21567=CARTESIAN_POINT ( 'NONE',  ( -20.50609665440969209, 24.89062500000000000, 20.50609665441005092 ) ) ;
#21573=CARTESIAN_POINT ( 'NONE',  ( 20.47846945139867003, 38.92149333240934794, -20.53372385742107653 ) ) ;
#21575=CARTESIAN_POINT ( 'NONE',  ( -15.01150461594642316, 49.95572916666665009, -26.00068869287341045 ) ) ;
#21579=CARTESIAN_POINT ( 'NONE',  ( -19.06425588902558133, 64.70274333240935505, 19.11951029504797006 ) ) ;
#21585=CARTESIAN_POINT ( 'NONE',  ( 6.988114217768294445, 24.31770833333332504, 26.07999730980477437 ) ) ;
#21592=CARTESIAN_POINT ( 'NONE',  ( -14.01125832528328985, 31.33034749907602290, -24.18731323226223040 ) ) ;
#21597=CARTESIAN_POINT ( 'NONE',  ( -6.988114217768288228, 53.53645833333332860, -26.07999730980477437 ) ) ;
#21602=CARTESIAN_POINT ( 'NONE',  ( 28.01184896238290278, 20.02083333333332860, -7.505752307973347470 ) ) ;
#21603=CARTESIAN_POINT ( 'NONE',  ( 0.04044903254992426173, 24.18006916759064140, -30.02300923189239867 ) ) ;
#21624=CARTESIAN_POINT ( 'NONE',  ( 26.06988505166735592, 38.93267333425729504, 7.025853678916393896 ) ) ;
#21631=CARTESIAN_POINT ( 'NONE',  ( 14.97647472619900455, 55.96576416574269786, -26.02091320914876960 ) ) ;
#21636=CARTESIAN_POINT ( 'NONE',  ( 24.20753774853756113, 27.32552083333332860, 13.97622843553589789 ) ) ;
#21639=CARTESIAN_POINT ( 'NONE',  ( -15.01150461594642138, 29.33072916666665719, -26.00068869287340334 ) ) ;
#21642=CARTESIAN_POINT ( 'NONE',  ( 25.98046417659858420, 42.51340250092398065, 15.04653450569292872 ) ) ;
#21644=CARTESIAN_POINT ( 'NONE',  ( -7.505752307973343918, 50.09895833333332860, -28.01184896238290989 ) ) ;
#21664=CARTESIAN_POINT ( 'NONE',  ( 26.06988505166735592, 14.87017333425730747, 7.025853678916393896 ) ) ;
#21669=CARTESIAN_POINT ( 'NONE',  ( -2.428612866367529427E-13, 53.67968750000000000, -27.95245687107223276 ) ) ;
#21670=CARTESIAN_POINT ( 'NONE',  ( 28.00173670424549499, 42.37017333425730925, 7.543491769121417612 ) ) ;
#21671=CARTESIAN_POINT ( 'NONE',  ( 20.53372385742108008, 32.90586833240934794, 20.47846945139866648 ) ) ;
#21675=CARTESIAN_POINT ( 'NONE',  ( -26.09010956794245217, 58.40065999907601935, -6.950374756619243755 ) ) ;
#21683=CARTESIAN_POINT ( 'NONE',  ( -6.950374756619716266, 48.09934000092398065, -26.09010956794232428 ) ) ;
#21687=CARTESIAN_POINT ( 'NONE',  ( 15.01150461594596308, 26.46614583333332149, -26.00068869287367335 ) ) ;
#21692=CARTESIAN_POINT ( 'NONE',  ( 20.50609665441005092, 61.84374999999998579, 20.50609665440969209 ) ) ;
#21700=CARTESIAN_POINT ( 'NONE',  ( 13.94119854578893580, 18.15326416574268720, -24.22776226481265383 ) ) ;
#21707=CARTESIAN_POINT ( 'NONE',  ( 26.07999730980477437, 37.20833333333332860, -6.988114217768290004 ) ) ;
#21713=CARTESIAN_POINT ( 'NONE',  ( -19.06425588902591173, 61.56288166759063074, -19.11951029504763611 ) ) ;
#21715=CARTESIAN_POINT ( 'NONE',  ( -20.50609665441004736, 49.81249999999999289, -20.50609665440969565 ) ) ;
#21728=CARTESIAN_POINT ( 'NONE',  ( -27.95245687107223986, 26.75819416759064495, -0.04044903254993292840 ) ) ;
#21733=CARTESIAN_POINT ( 'NONE',  ( -28.01184896238304134, 49.52604166666666430, -7.505752307972844761 ) ) ;
#21737=CARTESIAN_POINT ( 'NONE',  ( -7.505752307973343918, 26.03645833333333215, -28.01184896238290989 ) ) ;
#21743=CARTESIAN_POINT ( 'NONE',  ( 28.00173670424535644, 39.20795166574269075, -7.543491769121920321 ) ) ;
#21745=CARTESIAN_POINT ( 'NONE',  ( 2.740863092043355209E-13, 45.08593750000000000, 30.02300923189239867 ) ) ;
#21749=CARTESIAN_POINT ( 'NONE',  ( 14.01125832528330051, 63.98659749907601935, 24.18731323226221974 ) ) ;
#21756=CARTESIAN_POINT ( 'NONE',  ( -19.09188309203694445, 22.31250000000000000, -19.09188309203661049 ) ) ;
#21765=CARTESIAN_POINT ( 'NONE',  ( 26.06988505166722803, 28.89545166574268009, -7.025853678916862854 ) ) ;
#21769=CARTESIAN_POINT ( 'NONE',  ( 13.97622843553589966, 53.96614583333333570, -24.20753774853756113 ) ) ;
#21772=VERTEX_POINT ( 'NONE', #30317 ) ;
#21773=CARTESIAN_POINT ( 'NONE',  ( -30.02300923189239512, 21.88281249999999645, 2.654126918244515359E-13 ) ) ;
#21774=CARTESIAN_POINT ( 'NONE',  ( 28.02196122052045268, 24.89621500092397710, -7.468012846824774620 ) ) ;
#21791=CARTESIAN_POINT ( 'NONE',  ( 19.06425588902592239, 39.21913166759063785, 19.11951029504763611 ) ) ;
#21797=CARTESIAN_POINT ( 'NONE',  ( 25.98046417659831775, 56.25222249907602645, -15.04653450569338879 ) ) ;
#21801=CARTESIAN_POINT ( 'NONE',  ( -26.07999730980477437, 28.61458333333333215, 6.988114217768305103 ) ) ;
#21804=CARTESIAN_POINT ( 'NONE',  ( 20.50609665440969565, 30.04687500000000000, -20.50609665441004736 ) ) ;
#21807=CARTESIAN_POINT ( 'NONE',  ( -14.97647472619946285, 51.39361083425730925, -26.02091320914851025 ) ) ;
#21810=CARTESIAN_POINT ( 'NONE',  ( -26.00068869287340334, 59.40885416666666430, 15.01150461594643382 ) ) ;
#21818=DIRECTION ( 'NONE',  ( 1.000000000000000000, 0.000000000000000000, 0.000000000000000000 ) ) ;
#21823=CARTESIAN_POINT ( 'NONE',  ( -19.09188309203694445, 11.99999999999999645, -19.09188309203661049 ) ) ;
#21832=CARTESIAN_POINT ( 'NONE',  ( -27.95245687107223986, 13.00819416759064318, -0.04044903254993292840 ) ) ;
#21837=CARTESIAN_POINT ( 'NONE',  ( -2.428612866367529427E-13, 50.24218750000000711, -27.95245687107223276 ) ) ;
#21838=CARTESIAN_POINT ( 'NONE',  ( 20.53372385742072481, 38.35975666759064495, -20.47846945139902175 ) ) ;
#21839=CARTESIAN_POINT ( 'NONE',  ( -25.98046417659831420, 30.47097249907602290, 15.04653450569339945 ) ) ;
#21842=CARTESIAN_POINT ( 'NONE',  ( 24.22776226481265383, 56.82513916574268364, 13.94119854578893580 ) ) ;
#21848=CARTESIAN_POINT ( 'NONE',  ( -27.95245687107223986, 50.82069416759063785, -0.04044903254993292840 ) ) ;
#21852=CARTESIAN_POINT ( 'NONE',  ( 28.01184896238290278, 23.45833333333333215, -7.505752307973347470 ) ) ;
#21856=CARTESIAN_POINT ( 'NONE',  ( 28.01184896238290278, 57.83333333333333570, -7.505752307973347470 ) ) ;
#21863=CARTESIAN_POINT ( 'NONE',  ( -19.06425588902558133, 16.57774333240934794, 19.11951029504797006 ) ) ;
#21869=CARTESIAN_POINT ( 'NONE',  ( 6.988114217768294445, 41.50520833333333570, 26.07999730980477437 ) ) ;
#21875=CARTESIAN_POINT ( 'NONE',  ( 25.98046417659858420, 11.57590250092397355, 15.04653450569292872 ) ) ;
#21876=CARTESIAN_POINT ( 'NONE',  ( -2.584737979205441561E-13, 50.24218750000000711, -30.02300923189239512 ) ) ;
#21887=CARTESIAN_POINT ( 'NONE',  ( -26.09010956794232428, 23.17746500092398065, 6.950374756619732253 ) ) ;
#21892=CARTESIAN_POINT ( 'NONE',  ( 26.00068869287367335, 51.38802083333332149, 15.01150461594596308 ) ) ;
#21896=CARTESIAN_POINT ( 'NONE',  ( 7.505752307972854531, 26.32291666666666075, -28.01184896238303423 ) ) ;
#21901=CARTESIAN_POINT ( 'NONE',  ( 15.04653450569339945, 46.79909749907603356, 25.98046417659831775 ) ) ;
#21903=CARTESIAN_POINT ( 'NONE',  ( 7.505752307973351023, 44.94270833333332860, 28.01184896238290278 ) ) ;
#21907=CARTESIAN_POINT ( 'NONE',  ( 6.988114217767829928, 16.01041666666666075, -26.07999730980489872 ) ) ;
#21914=CARTESIAN_POINT ( 'NONE',  ( -26.07999730980490583, 18.58854166666666430, -6.988114217767815717 ) ) ;
#21921=CARTESIAN_POINT ( 'NONE',  ( 13.94119854578893580, 25.02826416574268720, -24.22776226481265383 ) ) ;
#21925=CARTESIAN_POINT ( 'NONE',  ( -19.09188309203660694, 55.82812499999999289, 19.09188309203694800 ) ) ;
#21930=CARTESIAN_POINT ( 'NONE',  ( -7.505752307972844761, 24.60416666666666430, 28.01184896238304134 ) ) ;
#21931=CARTESIAN_POINT ( 'NONE',  ( -28.02196122052045268, 23.17746500092398065, 7.468012846824790607 ) ) ;
#21941=CARTESIAN_POINT ( 'NONE',  ( -25.98046417659859486, 54.54465250092398776, -15.04653450569291628 ) ) ;
#21946=CARTESIAN_POINT ( 'NONE',  ( 24.18731323226221974, 39.06472249907601935, -14.01125832528328985 ) ) ;
#21953=CARTESIAN_POINT ( 'NONE',  ( -26.06988505166735237, 37.21392333425730214, -7.025853678916388567 ) ) ;
#21962=CARTESIAN_POINT ( 'NONE',  ( -0.04044903255044120238, 52.24180583240936215, -30.02300923189239867 ) ) ;
#21966=CARTESIAN_POINT ( 'NONE',  ( -2.428612866367529427E-13, 29.61718749999999645, -27.95245687107222921 ) ) ;
#21969=CARTESIAN_POINT ( 'NONE',  ( 15.01150461594596308, 33.34114583333332860, -26.00068869287367335 ) ) ;
#21972=CARTESIAN_POINT ( 'NONE',  ( -0.04044903254990864921, 49.96131916759065206, 30.02300923189239867 ) ) ;
#21974=CARTESIAN_POINT ( 'NONE',  ( -28.01184896238304134, 63.27604166666667140, -7.505752307972844761 ) ) ;
#21994=CARTESIAN_POINT ( 'NONE',  ( 24.20753774853756113, 65.13802083333334281, 13.97622843553589789 ) ) ;
#21999=CARTESIAN_POINT ( 'NONE',  ( 26.07999730980490227, 47.80729166666666430, 6.988114217767821046 ) ) ;
#22000=CARTESIAN_POINT ( 'NONE',  ( 15.04653450569292872, 34.77902750092397355, -25.98046417659857710 ) ) ;
#22001=CARTESIAN_POINT ( 'NONE',  ( 0.04044903255045854962, 26.46055583240935505, 30.02300923189239867 ) ) ;
#22005=CARTESIAN_POINT ( 'NONE',  ( 24.18731323226221974, 56.25222249907602645, -14.01125832528328985 ) ) ;
#22016=CARTESIAN_POINT ( 'NONE',  ( 26.00068869287340334, 37.06510416666666430, -15.01150461594642316 ) ) ;
#22021=CARTESIAN_POINT ( 'NONE',  ( -30.02300923189239512, 56.25781249999997868, 2.654126918244515359E-13 ) ) ;
#22028=CARTESIAN_POINT ( 'NONE',  ( -14.97647472619899389, 67.99701416574269786, 26.02091320914878025 ) ) ;
#22036=CARTESIAN_POINT ( 'NONE',  ( -26.07999730980477437, 42.36458333333332860, 6.988114217768305103 ) ) ;
#22042=CARTESIAN_POINT ( 'NONE',  ( -26.02091320914849959, 12.72173583425731458, 14.97647472619947528 ) ) ;
#22043=CARTESIAN_POINT ( 'NONE',  ( -20.50609665441004736, 53.25000000000000000, -20.50609665440969565 ) ) ;
#22055=CARTESIAN_POINT ( 'NONE',  ( 26.06988505166735592, 21.74517333425730925, 7.025853678916393896 ) ) ;
#22061=CARTESIAN_POINT ( 'NONE',  ( -2.584737979205441561E-13, 53.67968750000000000, -30.02300923189239512 ) ) ;
#22065=CARTESIAN_POINT ( 'NONE',  ( 26.00068869287340334, 26.75260416666666430, -15.01150461594642316 ) ) ;
#22070=CARTESIAN_POINT ( 'NONE',  ( 20.47846945139867003, 42.35899333240935505, -20.53372385742107653 ) ) ;
#22072=CARTESIAN_POINT ( 'NONE',  ( -30.02300923189239867, 56.25781249999999289, 2.654126918244514854E-13 ) ) ;
#22076=CARTESIAN_POINT ( 'NONE',  ( 2.584737979205441561E-13, 17.58593749999999645, 27.95245687107222921 ) ) ;
#22084=CARTESIAN_POINT ( 'NONE',  ( -6.988114217767819270, 34.91666666666666430, 26.07999730980490583 ) ) ;
#22090=CARTESIAN_POINT ( 'NONE',  ( -20.47846945139866648, 26.89024333240934439, 20.53372385742108008 ) ) ;
#22092=CARTESIAN_POINT ( 'NONE',  ( -6.950374756619247307, 30.04128499907601224, 26.09010956794245217 ) ) ;
#22096=CARTESIAN_POINT ( 'NONE',  ( 6.988114217767829928, 53.82291666666666430, -26.07999730980489872 ) ) ;
#22101=CARTESIAN_POINT ( 'NONE',  ( 7.505752307973351023, 27.75520833333332860, 28.01184896238290278 ) ) ;
#22102=CARTESIAN_POINT ( 'NONE',  ( 26.02091320914851025, 21.31548583425730925, -14.97647472619946463 ) ) ;
#22112=CARTESIAN_POINT ( 'NONE',  ( 20.47846945139902530, 56.40663166759065206, 20.53372385742071771 ) ) ;
#22115=CARTESIAN_POINT ( 'NONE',  ( -2.584737979205442066E-13, 22.74218749999999645, -30.02300923189239867 ) ) ;
#22120=CARTESIAN_POINT ( 'NONE',  ( -19.06425588902558133, 44.07774333240935505, 19.11951029504797006 ) ) ;
#22126=CARTESIAN_POINT ( 'NONE',  ( -26.09010956794232428, 40.36496500092396644, 6.950374756619732253 ) ) ;
#22134=CARTESIAN_POINT ( 'NONE',  ( -15.04653450569338524, 58.83034749907602645, -25.98046417659831775 ) ) ;
#22137=CARTESIAN_POINT ( 'NONE',  ( -6.988114217768288228, 26.03645833333333215, -26.07999730980477437 ) ) ;
#22139=CARTESIAN_POINT ( 'NONE',  ( 7.505752307972854531, 26.32291666666666075, -28.01184896238303423 ) ) ;
#22142=CARTESIAN_POINT ( 'NONE',  ( -26.02091320914849959, 50.53423583425731636, 14.97647472619947528 ) ) ;
#22145=CARTESIAN_POINT ( 'NONE',  ( 30.02300923189239512, 61.41406250000000711, -2.619432448724977703E-13 ) ) ;
#22166=CARTESIAN_POINT ( 'NONE',  ( -6.950374756619716266, 10.28684000092397532, -26.09010956794232428 ) ) ;
#22171=CARTESIAN_POINT ( 'NONE',  ( -6.988114217768288228, 46.66145833333332860, -26.07999730980477437 ) ) ;
#22172=CARTESIAN_POINT ( 'NONE',  ( -14.97647472619946285, 41.08111083425730214, -26.02091320914851025 ) ) ;
#22173=CARTESIAN_POINT ( 'NONE',  ( 28.00173670424535644, 28.89545166574268009, -7.543491769121920321 ) ) ;
#22176=CARTESIAN_POINT ( 'NONE',  ( -6.950374756619247307, 54.10378499907602645, 26.09010956794245217 ) ) ;
#22184=CARTESIAN_POINT ( 'NONE',  ( -2.584737979205441561E-13, 33.05468750000000000, -30.02300923189239512 ) ) ;
#22189=CARTESIAN_POINT ( 'NONE',  ( 20.50609665441005092, 54.96875000000000000, 20.50609665440969209 ) ) ;
#22196=CARTESIAN_POINT ( 'NONE',  ( 26.09010956794244507, 15.43190999907601935, 6.950374756619249084 ) ) ;
#22204=CARTESIAN_POINT ( 'NONE',  ( 13.97622843553633665, 37.92447916666666430, 24.20753774853730889 ) ) ;
#22209=CARTESIAN_POINT ( 'NONE',  ( -7.468012846824771955, 10.28684000092397532, -28.02196122052045624 ) ) ;
#22210=CARTESIAN_POINT ( 'NONE',  ( 15.01150461594596308, 50.52864583333333570, -26.00068869287367335 ) ) ;
#22221=CARTESIAN_POINT ( 'NONE',  ( 24.18731323226247554, 35.63840250092398065, 14.01125832528285997 ) ) ;
#22222=ORIENTED_EDGE ( 'NONE', *, *, #28799, .T. ) ;
#22226=CARTESIAN_POINT ( 'NONE',  ( -30.02300923189239512, 49.38281249999997868, 2.654126918244515359E-13 ) ) ;
#22232=CARTESIAN_POINT ( 'NONE',  ( -15.01150461594642138, 32.76822916666666430, -26.00068869287340334 ) ) ;
#22237=CARTESIAN_POINT ( 'NONE',  ( -28.02196122052058413, 44.65065999907601935, -7.468012846824272799 ) ) ;
#22239=CARTESIAN_POINT ( 'NONE',  ( 20.50609665440969565, 54.10937499999999289, -20.50609665441004736 ) ) ;
#22243=CARTESIAN_POINT ( 'NONE',  ( 13.97622843553589966, 12.71614583333333037, -24.20753774853756113 ) ) ;
#22251=CARTESIAN_POINT ( 'NONE',  ( -24.20753774853756823, 35.91927083333332860, -13.97622843553588723 ) ) ;
#22256=CARTESIAN_POINT ( 'NONE',  ( 20.53372385742108008, 22.59336833240935505, 20.47846945139866648 ) ) ;
#22258=CARTESIAN_POINT ( 'NONE',  ( 0.04044903255044120238, 40.21055583240935505, 27.95245687107223276 ) ) ;
#22262=CARTESIAN_POINT ( 'NONE',  ( 2.584737979205441561E-13, 58.83593750000000000, 27.95245687107222921 ) ) ;
#22267=CARTESIAN_POINT ( 'NONE',  ( -28.01184896238304134, 25.46354166666666430, -7.505752307972844761 ) ) ;
#22268=CARTESIAN_POINT ( 'NONE',  ( -7.543491769121417612, 26.04204833425729859, 28.00173670424549499 ) ) ;
#22277=CARTESIAN_POINT ( 'NONE',  ( -7.468012846824771955, 51.53684000092397355, -28.02196122052045624 ) ) ;
#22280=CARTESIAN_POINT ( 'NONE',  ( -15.01150461594642316, 29.33072916666665719, -26.00068869287341045 ) ) ;
#22285=CARTESIAN_POINT ( 'NONE',  ( -19.11951029504797006, 41.49961833240934794, -19.06425588902558133 ) ) ;
#22291=CARTESIAN_POINT ( 'NONE',  ( -13.94119854578936923, 47.95611083425732346, -24.22776226481241224 ) ) ;
#22298=CARTESIAN_POINT ( 'NONE',  ( -15.04653450569338524, 65.70534749907602645, -25.98046417659831775 ) ) ;
#22302=CARTESIAN_POINT ( 'NONE',  ( -6.988114217767819270, 24.60416666666666430, 26.07999730980490583 ) ) ;
#22305=CARTESIAN_POINT ( 'NONE',  ( -30.02300923189239512, 39.07031249999997868, 2.654126918244515359E-13 ) ) ;
#22308=CARTESIAN_POINT ( 'NONE',  ( -7.468012846824771955, 48.09934000092398065, -28.02196122052045624 ) ) ;
#22311=CARTESIAN_POINT ( 'NONE',  ( -20.50609665440969209, 62.70312500000000000, 20.50609665441005092 ) ) ;
#22317=PLANE ( 'NONE',  #600 ) ;
#22330=CARTESIAN_POINT ( 'NONE',  ( -7.025853678916393008, 15.72954833425730925, 26.06988505166735592 ) ) ;
#22335=CARTESIAN_POINT ( 'NONE',  ( 19.09188309203661049, 47.23437499999999289, -19.09188309203694445 ) ) ;
#22336=CARTESIAN_POINT ( 'NONE',  ( -26.02091320914849959, 36.78423583425730214, 14.97647472619947528 ) ) ;
#22337=CARTESIAN_POINT ( 'NONE',  ( 20.53372385742108008, 26.03086833240935860, 20.47846945139866648 ) ) ;
#22340=CARTESIAN_POINT ( 'NONE',  ( -27.95245687107223986, 51.38243083240936215, 0.04044903255043252877 ) ) ;
#22347=CARTESIAN_POINT ( 'NONE',  ( -26.00068869287368756, 35.91927083333332860, -15.01150461594595775 ) ) ;
#22351=CARTESIAN_POINT ( 'NONE',  ( 28.01184896238290278, 61.27083333333332860, -7.505752307973347470 ) ) ;
#22359=CARTESIAN_POINT ( 'NONE',  ( -13.94119854578892514, 19.87201416574269075, 24.22776226481266448 ) ) ;
#22367=CARTESIAN_POINT ( 'NONE',  ( 26.07999730980490227, 40.93229166666666430, 6.988114217767821046 ) ) ;
#22373=CARTESIAN_POINT ( 'NONE',  ( 7.543491769121427382, 14.01079833425730747, -28.00173670424548433 ) ) ;
#22374=CARTESIAN_POINT ( 'NONE',  ( 28.01184896238304134, 58.11979166666665719, 7.505752307972846538 ) ) ;
#22384=CARTESIAN_POINT ( 'NONE',  ( 14.01125832528286352, 34.77902750092397355, -24.18731323226246843 ) ) ;
#22389=CARTESIAN_POINT ( 'NONE',  ( 28.01184896238304134, 58.11979166666665719, 7.505752307972846538 ) ) ;
#22393=CARTESIAN_POINT ( 'NONE',  ( 20.50609665440969565, 26.60937499999999645, -20.50609665441004736 ) ) ;
#22399=CARTESIAN_POINT ( 'NONE',  ( -15.04653450569338524, 41.64284749907602645, -25.98046417659831775 ) ) ;
#22401=CARTESIAN_POINT ( 'NONE',  ( 20.50609665441005092, 54.96875000000000000, 20.50609665440969209 ) ) ;
#22404=CARTESIAN_POINT ( 'NONE',  ( 19.09188309203694800, 13.71874999999999467, 19.09188309203660694 ) ) ;
#22414=CARTESIAN_POINT ( 'NONE',  ( 0.04044903255045854962, 23.02305583240935860, 30.02300923189239867 ) ) ;
#22416=CARTESIAN_POINT ( 'NONE',  ( -6.950374756619247307, 36.91628499907601224, 26.09010956794245217 ) ) ;
#22419=CARTESIAN_POINT ( 'NONE',  ( 24.20753774853756113, 65.13802083333334281, 13.97622843553589789 ) ) ;
#22425=CARTESIAN_POINT ( 'NONE',  ( 26.00068869287340334, 30.19010416666665719, -15.01150461594642316 ) ) ;
#22426=CARTESIAN_POINT ( 'NONE',  ( -7.543491769121417612, 29.47954833425730570, 28.00173670424549499 ) ) ;
#22436=CARTESIAN_POINT ( 'NONE',  ( -14.97647472619946285, 58.26861083425732346, -26.02091320914851025 ) ) ;
#22439=CARTESIAN_POINT ( 'NONE',  ( -15.01150461594595775, 28.18489583333333215, 26.00068869287368756 ) ) ;
#22443=CARTESIAN_POINT ( 'NONE',  ( -24.18731323226221974, 44.22097249907603356, 14.01125832528330406 ) ) ;
#22449=CARTESIAN_POINT ( 'NONE',  ( 26.06988505166735592, 45.80767333425730925, 7.025853678916393896 ) ) ;
#22455=CARTESIAN_POINT ( 'NONE',  ( -7.468012846824272799, 64.41628499907602645, 28.02196122052058413 ) ) ;
#22459=CARTESIAN_POINT ( 'NONE',  ( -19.09188309203660694, 35.20312500000000000, 19.09188309203694800 ) ) ;
#22462=CARTESIAN_POINT ( 'NONE',  ( 28.01184896238304134, 37.49479166666666430, 7.505752307972846538 ) ) ;
#22466=CARTESIAN_POINT ( 'NONE',  ( 20.47846945139902530, 63.28163166759064495, 20.53372385742071771 ) ) ;
#22467=CARTESIAN_POINT ( 'NONE',  ( -14.01125832528285109, 63.99777750092396644, 24.18731323226248264 ) ) ;
#22471=CARTESIAN_POINT ( 'NONE',  ( -7.505752307973343918, 63.84895833333332860, -28.01184896238290989 ) ) ;
#22489=CARTESIAN_POINT ( 'NONE',  ( 24.22776226481241224, 21.31548583425730925, -13.94119854578936923 ) ) ;
#22495=CARTESIAN_POINT ( 'NONE',  ( 7.468012846824777284, 46.38059000092397355, 28.02196122052045268 ) ) ;
#22496=CARTESIAN_POINT ( 'NONE',  ( -14.97647472619899389, 37.05951416574268364, 26.02091320914878025 ) ) ;
#22500=CARTESIAN_POINT ( 'NONE',  ( -0.04044903255042732459, 65.99180583240935505, -27.95245687107223986 ) ) ;
#22502=CARTESIAN_POINT ( 'NONE',  ( 20.50609665440969565, 12.85937500000000000, -20.50609665441004736 ) ) ;
#22508=CARTESIAN_POINT ( 'NONE',  ( -30.02300923189239512, 35.63281249999998579, 2.654126918244515359E-13 ) ) ;
#22515=CARTESIAN_POINT ( 'NONE',  ( -20.50609665440969209, 62.70312500000000000, 20.50609665441005092 ) ) ;
#22523=CARTESIAN_POINT ( 'NONE',  ( -0.04044903255042732459, 21.30430583240935860, -27.95245687107223986 ) ) ;
#22532=CARTESIAN_POINT ( 'NONE',  ( -6.988114217768288228, 46.66145833333332860, -26.07999730980477437 ) ) ;
#22537=CARTESIAN_POINT ( 'NONE',  ( -7.025853678916393008, 63.85454833425732346, 26.06988505166735592 ) ) ;
#22538=CARTESIAN_POINT ( 'NONE',  ( 15.01150461594596308, 60.84114583333332860, -26.00068869287367335 ) ) ;
#22543=CARTESIAN_POINT ( 'NONE',  ( -19.09188309203660694, 66.14062500000000000, 19.09188309203694800 ) ) ;
#22547=CARTESIAN_POINT ( 'NONE',  ( -27.95245687107223986, 37.07069416759063785, -0.04044903254993292840 ) ) ;
#22552=CARTESIAN_POINT ( 'NONE',  ( 20.50609665440969565, 64.42187499999998579, -20.50609665441004736 ) ) ;
#22556=CARTESIAN_POINT ( 'NONE',  ( 7.505752307972854531, 36.63541666666666430, -28.01184896238303423 ) ) ;
#22562=CARTESIAN_POINT ( 'NONE',  ( 20.47846945139867003, 49.23399333240936215, -20.53372385742107653 ) ) ;
#22565=CARTESIAN_POINT ( 'NONE',  ( 7.505752307972854531, 53.82291666666666430, -28.01184896238303423 ) ) ;
#22571=CARTESIAN_POINT ( 'NONE',  ( -24.20753774853730889, 18.15885416666666075, 13.97622843553633842 ) ) ;
#22582=CARTESIAN_POINT ( 'NONE',  ( 28.00173670424535644, 22.02045166574269075, -7.543491769121920321 ) ) ;
#22584=CARTESIAN_POINT ( 'NONE',  ( 26.09010956794244507, 39.49440999907601224, 6.950374756619249084 ) ) ;
#22588=CARTESIAN_POINT ( 'NONE',  ( 19.09188309203661049, 60.98437499999999289, -19.09188309203694445 ) ) ;
#22594=CARTESIAN_POINT ( 'NONE',  ( -20.50609665440969209, 35.20312500000000000, 20.50609665441005092 ) ) ;
#22595=CARTESIAN_POINT ( 'NONE',  ( 30.02300923189239867, 35.35194416759064495, 0.04044903254992252006 ) ) ;
#22604=CARTESIAN_POINT ( 'NONE',  ( 7.505752307972854531, 12.57291666666666252, -28.01184896238303423 ) ) ;
#22607=CARTESIAN_POINT ( 'NONE',  ( -2.584737979205442066E-13, 26.17968750000000000, -30.02300923189239867 ) ) ;
#22613=CARTESIAN_POINT ( 'NONE',  ( 26.09010956794244507, 46.36940999907602645, 6.950374756619249084 ) ) ;
#22620=CARTESIAN_POINT ( 'NONE',  ( 24.18731323226247554, 52.82590250092398065, 14.01125832528285997 ) ) ;
#22628=CARTESIAN_POINT ( 'NONE',  ( 20.47846945139867003, 62.98399333240935505, -20.53372385742107653 ) ) ;
#22634=CARTESIAN_POINT ( 'NONE',  ( -13.97622843553588901, 35.05989583333332860, 24.20753774853756823 ) ) ;
#22638=CARTESIAN_POINT ( 'NONE',  ( 20.50609665441005092, 41.21875000000000000, 20.50609665440969209 ) ) ;
#22641=CARTESIAN_POINT ( 'NONE',  ( 26.02091320914851025, 55.69048583425730925, -14.97647472619946463 ) ) ;
#22642=CARTESIAN_POINT ( 'NONE',  ( -19.06425588902591173, 61.56288166759063074, -19.11951029504763611 ) ) ;
#22644=CARTESIAN_POINT ( 'NONE',  ( -14.97647472619899389, 16.43451416574268720, 26.02091320914878025 ) ) ;
#22663=CARTESIAN_POINT ( 'NONE',  ( 19.11951029504763611, 24.60975666759063785, -19.06425588902591173 ) ) ;
#22669=CARTESIAN_POINT ( 'NONE',  ( 26.02091320914851025, 48.81548583425731636, -14.97647472619946463 ) ) ;
#22671=CARTESIAN_POINT ( 'NONE',  ( 7.468012846824281681, 35.19753499907601935, -28.02196122052058058 ) ) ;
#22674=CARTESIAN_POINT ( 'NONE',  ( -13.94119854578892514, 67.99701416574269786, 24.22776226481266448 ) ) ;
#22677=CARTESIAN_POINT ( 'NONE',  ( 28.01184896238304134, 16.86979166666666075, 7.505752307972846538 ) ) ;
#22686=CARTESIAN_POINT ( 'NONE',  ( 20.50609665440969565, 30.04687500000000000, -20.50609665441004736 ) ) ;
#22694=CARTESIAN_POINT ( 'NONE',  ( 20.50609665441005092, 13.71874999999999467, 20.50609665440969209 ) ) ;
#22699=CARTESIAN_POINT ( 'NONE',  ( -13.94119854578892514, 23.30951416574269075, 24.22776226481266448 ) ) ;
#22709=CARTESIAN_POINT ( 'NONE',  ( -24.20753774853756823, 49.66927083333330728, -13.97622843553588723 ) ) ;
#22715=CARTESIAN_POINT ( 'NONE',  ( 28.00173670424549499, 21.74517333425730925, 7.543491769121417612 ) ) ;
#22717=CARTESIAN_POINT ( 'NONE',  ( 26.00068869287367335, 61.70052083333331439, 15.01150461594596308 ) ) ;
#22729=CARTESIAN_POINT ( 'NONE',  ( -24.22776226481240514, 33.34673583425730214, 13.94119854578937812 ) ) ;
#22736=CARTESIAN_POINT ( 'NONE',  ( -15.01150461594642138, 43.08072916666666430, -26.00068869287340334 ) ) ;
#22740=CARTESIAN_POINT ( 'NONE',  ( 14.97647472619900455, 52.52826416574268364, -26.02091320914876960 ) ) ;
#22742=CARTESIAN_POINT ( 'NONE',  ( -28.01184896238290278, 56.11458333333332860, 7.505752307973363457 ) ) ;
#22747=CARTESIAN_POINT ( 'NONE',  ( 27.95245687107222921, 27.03906250000000000, -2.463307335887066074E-13 ) ) ;
#22758=CARTESIAN_POINT ( 'NONE',  ( 25.98046417659831775, 28.75222249907602290, -15.04653450569338879 ) ) ;
#22760=CARTESIAN_POINT ( 'NONE',  ( -13.94119854578892514, 33.62201416574269075, 24.22776226481266448 ) ) ;
#22764=CARTESIAN_POINT ( 'NONE',  ( 26.07999730980490227, 64.99479166666665719, 6.988114217767821046 ) ) ;
#22769=CARTESIAN_POINT ( 'NONE',  ( 2.740863092043355209E-13, 34.77343750000000000, 30.02300923189239512 ) ) ;
#22770=CARTESIAN_POINT ( 'NONE',  ( -28.02196122052045268, 33.48996500092397355, 7.468012846824790607 ) ) ;
#22781=CARTESIAN_POINT ( 'NONE',  ( 26.00068869287367335, 13.57552083333332682, 15.01150461594596308 ) ) ;
#22784=CARTESIAN_POINT ( 'NONE',  ( -28.01184896238290278, 28.61458333333333215, 7.505752307973363457 ) ) ;
#22789=CARTESIAN_POINT ( 'NONE',  ( 24.18731323226221974, 49.37722249907602645, -14.01125832528328985 ) ) ;
#22796=CARTESIAN_POINT ( 'NONE',  ( -24.18731323226248264, 44.23215250092398065, -14.01125832528284931 ) ) ;
#22803=CARTESIAN_POINT ( 'NONE',  ( -20.47846945139866648, 68.14024333240935505, 20.53372385742108008 ) ) ;
#22807=CARTESIAN_POINT ( 'NONE',  ( -24.20753774853756823, 39.35677083333331439, -13.97622843553588723 ) ) ;
#22810=CARTESIAN_POINT ( 'NONE',  ( 15.01150461594643204, 41.36197916666666430, 26.00068869287340334 ) ) ;
#22813=CARTESIAN_POINT ( 'NONE',  ( 15.04653450569292872, 55.40402750092397355, -25.98046417659857710 ) ) ;
#22814=CARTESIAN_POINT ( 'NONE',  ( -26.09010956794232428, 60.98996500092398065, 6.950374756619732253 ) ) ;
#22816=CARTESIAN_POINT ( 'NONE',  ( -20.53372385742107653, 13.99961833240935327, -20.47846945139867003 ) ) ;
#22835=CARTESIAN_POINT ( 'NONE',  ( 26.09010956794232428, 18.02121500092397710, -6.950374756619718042 ) ) ;
#22840=CARTESIAN_POINT ( 'NONE',  ( -20.47846945139902175, 51.25038166759065206, -20.53372385742072481 ) ) ;
#22843=CARTESIAN_POINT ( 'NONE',  ( -14.97647472619899389, 33.62201416574269075, 26.02091320914878025 ) ) ;
#22847=CARTESIAN_POINT ( 'NONE',  ( -7.025853678916861966, 62.41107666574269075, -26.06988505166722803 ) ) ;
#22851=CARTESIAN_POINT ( 'NONE',  ( -2.584737979205441561E-13, 15.86718749999999645, -30.02300923189239512 ) ) ;
#22857=CARTESIAN_POINT ( 'NONE',  ( 15.01150461594643204, 41.36197916666666430, 26.00068869287340334 ) ) ;
#22867=CARTESIAN_POINT ( 'NONE',  ( 7.505752307972854531, 16.01041666666666075, -28.01184896238303423 ) ) ;
#22872=CARTESIAN_POINT ( 'NONE',  ( 19.11951029504797006, 22.59336833240935505, 19.06425588902558133 ) ) ;
#22881=CARTESIAN_POINT ( 'NONE',  ( -2.428612866367529427E-13, 50.24218750000000711, -27.95245687107222921 ) ) ;
#22885=CARTESIAN_POINT ( 'NONE',  ( 6.988114217767829928, 29.76041666666666430, -26.07999730980489872 ) ) ;
#22887=CARTESIAN_POINT ( 'NONE',  ( -14.97647472619946285, 23.89361083425731280, -26.02091320914851025 ) ) ;
#22888=CARTESIAN_POINT ( 'NONE',  ( -26.00068869287368756, 59.98177083333332149, -15.01150461594595775 ) ) ;
#22898=CARTESIAN_POINT ( 'NONE',  ( -7.025853678916393008, 32.91704833425729504, 26.06988505166735592 ) ) ;
#22902=CARTESIAN_POINT ( 'NONE',  ( 30.02300923189239512, 16.72656249999999645, -2.619432448724977703E-13 ) ) ;
#22908=CARTESIAN_POINT ( 'NONE',  ( 20.50609665441005092, 41.21875000000000000, 20.50609665440969209 ) ) ;
#22909=( BOUNDED_SURFACE ( )  B_SPLINE_SURFACE ( 3, 2, ( 
 ( #4879, #15870, #15704, #26159, #28552, #25650, #10210, #20852, #7277, #2653, #10374, #12604, #18449, #25815, #31298, #23073, #2128, #33534, #5050, #23251, #33713, #20691, #12434, #31132, #20334, #10038, #5393, #7624, #15186, #9857, #20512, #18104, #30958, #22902, #28726, #30784, #13115, #17760, #21020, #31471, #15534, #25986, #7962, #1959, #23589, #18281, #2479, #28218, #12778, #15360, #12947, #23420, #7790, #54, #10542, #4705, #7456, #17940, #2305, #3160, #8791, #26986, #31800, #21190, #11376, #5561, #3323, #16209, #8461, #13631, #18950, #24095, #31632, #10710, #29395, #23758, #13791, #16040, #5895, #24259, #21852, #729, #26496, #32134, #8629, #19112, #16374, #26663, #11054, #2990, #563, #10882, #26827, #895, #32297, #21357, #13955, #11214, #29551, #21518, #19275, #21687, #16534, #3486, #26327, #13459, #29716, #29056, #8291, #222, #23928, #6051, #397, #6222, #5731, #24418, #2815, #18781, #13282, #8130, #18619, #29226, #31968, #32461, #3649, #30054, #22686, #25258, #11533, #25083, #30566, #30222, #11701, #14456, #16702, #17033, #4152, #1733, #12213, #19945, #1053, #33136, #1220, #6390, #24912, #32794, #9287, #22184, #3816, #6722, #3982, #1562, #30390, #8961, #14625, #19771, #6558, #17204, #4320, #27663, #14125, #9639, #24582, #14288, #12038, #22508, #32960, #22347, #27493, #9462, #19444, #11874, #24745, #6892, #17373, #22016, #27836, #16867, #29889, #20122, #14794, #32631, #27157, #27328, #9125, #19607, #1398, #15143, #23376, #2257, #18235, #23202, #33664, #17717, #10334, #15662, #4663, #12388, #20810, #28176, #25607, #5003, #2086, #12561, #23032, #22857, #20463, #28506, #26111, #25435, #31254, #4491, #12731, #13070, #33489, #15486, #7408, #20291, #7746, #8, #15312, #17546, #30914, #25940, #9991, #30739, #4832, #10161, #20643, #17894, #28347, #31086, #25771, #2434, #28681, #33315, #12901, #7583, #18061, #33837, #5179, #2609, #14967, #23546, #1911, #10497, #20975, #7063, #28005, #9814, #7231, #11006, #13237, #26620, #29015, #3116, #13745, #28848, #31923, #31588, #23711, #26944, #11173, #15996, #8586, #26786, #21644, #29351, #5687, #5515, #24216, #13588, #19070, #24051, #519, #8087, #687, #6014, #26452, #2773, #32090, #18574, #2943, #5851, #13414, #23882, #353, #177, #10837, #18904, #16489, #15828, #29510, #5347, #21476, #3444, #21315, #16330, #31756, #10667, #13914, #24381, #16165, #7918, #8247, #3278, #18740, #8415, #854, #11334, #31425, #18403, #26282, #21146, #29182, #11495, #25217, #24541, #6351, #19235, #8919, #9250, #19402, #1695, #1182, #24871, #25045, #14248, #14585, #29673, #11833, #21810, #27285, #3610, #8751, #11663, #27796, #30352, #16660, #30180, #32258, #1354, #16830, #19570, #6178, #22145, #19735, #6854, #17332, #1526, #27117, #4280, #3777, #30018, #22311, #9088, #14083, #1012, #21974, #27452, #32589, #14754, #22471, #24705, #32422, #29851, #6522, #32756, #16994, #3943, #14418, #6683, #17168, #27624, #4111, #12000, #32919, #9418, #19903, #20422, #28304, #15444, #4792, #14926, #2211 ),
 ( #22816, #7367, #23159, #2046, #4966, #30871, #20602, #31047, #12171, #25392, #23338, #4448, #9770, #9599, #33275, #15271, #20253, #22644, #4622, #17851, #7540, #17674, #10121, #30524, #25732, #33096, #28136, #1869, #7022, #25566, #20081, #17504, #12347, #18025, #27966, #25899, #12690, #28471, #30696, #33622, #7192, #15101, #12521, #22989, #2392, #33448, #12861, #9946, #6627, #24986, #1469, #3886, #29961, #32862, #30124, #17273, #22582, #1123, #6794, #11945, #22256, #9359, #30465, #22414, #6295, #17448, #16771, #6466, #19840, #27736, #4224, #14526, #19678, #30293, #24649, #4051, #16940, #14698, #25156, #27230, #1632, #9034, #11608, #17106, #3724, #12110, #14865, #1294, #33033, #9193, #22090, #9537, #1808, #27565, #19349, #32699, #20019, #27397, #6963, #27909, #4391, #25330, #12284, #22758, #8864, #29791, #32534, #14194, #19513, #14359, #24817, #11776, #31521, #23470, #18669, #21242, #5948, #13339, #614, #7842, #277, #3043, #104, #12999, #31851, #13163, #29107, #13681, #23812, #15923, #26879, #26717, #3213, #5612, #2703, #31685, #8344, #18331, #24145, #21406, #23640, #29445, #2870, #18833, #10595, #21072, #8015, #16096, #10764, #8179, #26547, #33932, #13515, #31349, #18500, #16427, #23978, #26209, #20901, #28944, #449, #5442, #10423, #5780, #28776, #16260, #5273, #32019, #8515, #10931, #29279, #19001, #15755, #11104, #21573, #26379, #21743, #9014, #14009, #946, #24633, #1106, #16920, #11590, #785, #32189, #24311, #19496, #14176, #19824, #4034, #8846, #8683, #22399, #16587, #14341, #27213, #29944, #22070, #6448, #32514, #19167, #29605, #27380, #11267, #24799, #27043, #3869, #1276, #32847, #11756, #3537, #9339, #30276, #22237, #32682, #6776, #17257, #17087, #19661, #9177, #6106, #30104, #24471, #11426, #6610, #27547, #14509, #24968, #21901, #32353, #19328, #1450, #11929, #3374, #13845, #29770, #6278, #16754, #3704, #4715, #17596, #9866, #4545, #20343, #15020, #22562, #12093, #30793, #25139, #15195, #17429, #7286, #25659, #23260, #2138, #27890, #33543, #10045, #20524, #17770, #28058, #12444, #4374, #25490, #12264, #28229, #2314, #12787, #22740, #15369, #7114, #12613, #14678, #27718, #30448, #1615, #33014, #9519, #1969, #22914, #14848, #23082, #20001, #4206, #33191, #6946, #33370, #30968, #20700, #7467, #25824, #25314, #17950, #28399, #1787, #9694, #4888, #20174, #33723, #10221, #31142, #30618, #7633, #31810, #8301, #10721, #7801, #26337, #3000, #23431, #18793, #26507, #28735, #573, #7971, #13473, #5231, #18290, #15715, #21199, #5403, #15880, #2826, #28563, #13295, #2488, #26170, #11064, #23768, #31307, #25995, #2663, #235, #13123, #5058, #10893, #12957, #21366, #33891, #23598, #31643, #18115, #18458, #5571, #26676, #13641, #29237, #10383, #3171, #63, #10550, #8141, #18630, #29066, #21031, #31481, #16053, #23938, #407, #5741, #20861, #16221, #24105, #28902, #21529, #31977, #15543, #5907, #17045, #16384, #29561, #1066, #6404, #27341, #14136, #19285, #22028, #24271, #3661, #6062, #24593, #24757, #26837, #8973 ),
 ( #1235, #11546, #19619, #32472, #19455, #19124, #11713, #27506, #16545, #13803, #22196, #26998, #3496, #16878, #13965, #24429, #905, #738, #21863, #29902, #3995, #3332, #32643, #11224, #3827, #14468, #11386, #14301, #8803, #21700, #9138, #1410, #16714, #18961, #32310, #30065, #29728, #6571, #24925, #27168, #11887, #22359, #8474, #29405, #32145, #8639, #6233, #1576, #17387, #17732, #25621, #22523, #28189, #2274, #12226, #1925, #2101, #25273, #12574, #6736, #22872, #12748, #4335, #14639, #19783, #22699, #4849, #7423, #27677, #7244, #32806, #12402, #14808, #4167, #17909, #12053, #9827, #33151, #14979, #9655, #25449, #20135, #25099, #17218, #33330, #30232, #20303, #32974, #30754, #4677, #28362, #15156, #9478, #23045, #33503, #10007, #20479, #30580, #17560, #19960, #7076, #27852, #30930, #15330, #25785, #1746, #9299, #28017, #30408, #6907, #4505, #25956, #10179, #7597, #18075, #31441, #7933, #12916, #26299, #28524, #23221, #7764, #33680, #28865, #18421, #16633, #23561, #10854, #5019, #10514, #13254, #10348, #20661, #8102, #23392, #5362, #23897, #25, #26127, #3583, #2960, #13429, #15842, #33854, #2788, #18589, #15502, #368, #31604, #20826, #6148, #13087, #29029, #31270, #18250, #28697, #23728, #20992, #194, #10681, #31101, #21162, #2450, #5194, #27089, #5532, #15678, #2624, #16013, #26467, #21329, #31770, #8725, #19208, #29646, #21946, #33066, #9571, #9223, #19707, #20048, #6995, #27767, #30326, #27593, #32397, #30153, #24680, #11636, #1326, #11807, #4084, #22285, #11472, #8892, #987, #6657, #24846, #30494, #14727, #19376, #1154, #17140, #11974, #32890, #14558, #32730, #25018, #29822, #1498, #22120, #22443, #6822, #6326, #9389, #19873, #14055, #3917, #17477, #32563, #25188, #17304, #4252, #1665, #12140, #9062, #22613, #27939, #24517, #16802, #27259, #19543, #3750, #14224, #29991, #6495, #16968, #27426, #14389, #2362, #2017, #12492, #22961, #20226, #17821, #25871, #23479, #22789, #18167, #1839, #10094, #10432, #30845, #12836, #4764, #17646, #7681, #31358, #12659, #14897, #28277, #23310, #33419, #28444, #31191, #23128, #33940, #17999, #28609, #5109, #4422, #28107, #7850, #7164, #9917, #33775, #15593, #4594, #10266, #18338, #15242, #7514, #26047, #7336, #2540, #12319, #4935, #25361, #20394, #30666, #33242, #25704, #20907, #13007, #9740, #20748, #15071, #15417, #2185, #33594, #25538, #20573, #31016, #3380, #24316, #32025, #13171, #13851, #13346, #18508, #26555, #10939, #21414, #23819, #15931, #18839, #16104, #3218, #8522, #21080, #26722, #31857, #8187, #29285, #16432, #8349, #26218, #790, #28954, #3051, #13686, #111, #19006, #24150, #5450, #11273, #18677, #621, #26387, #2879, #285, #5785, #13522, #23985, #457, #5281, #16266, #23649, #10773, #21749, #11109, #8022, #2710, #21250, #21579, #31694, #15764, #29450, #10602, #5952, #31528, #32194, #8688, #26884, #28783, #29116, #5620, #32852, #1456, #32688, #3542, #24805, #29777, #16759, #6454, #16928, #9183, #27386, #16592, #14014, #6111, #1283, #29950, #1622, #19830 ),
 ( #24477, #11762, #27049, #30112, #8852, #22243, #6616, #14685, #17094, #19333, #24974, #11935, #22404, #19667, #19502, #3875, #6283, #14348, #3711, #27553, #27725, #4213, #14181, #6784, #32521, #4041, #951, #19172, #21907, #11431, #32358, #27218, #14515, #9347, #24637, #30282, #1111, #29609, #11596, #22076, #17262, #25146, #12100, #22571, #33021, #9020, #30800, #33550, #30625, #9527, #28406, #9701, #15202, #10228, #9872, #12451, #23439, #23268, #33730, #2145, #7121, #4722, #25831, #6952, #10051, #7293, #20008, #33377, #15551, #28065, #20708, #4896, #31150, #7475, #17778, #17603, #2321, #25666, #7641, #12620, #23087, #20181, #12794, #18125, #4552, #14855, #28570, #15031, #25496, #17957, #1976, #22921, #20350, #25321, #28236, #30975, #5066, #27897, #26003, #17436, #20532, #2496, #15376, #12965, #30455, #22747, #4380, #1795, #12273, #33198, #23778, #8309, #31489, #23946, #26683, #8149, #18968, #13481, #24112, #580, #33900, #23605, #3339, #2672, #18465, #18800, #3179, #72, #29244, #13810, #13303, #3009, #13648, #26345, #11070, #7809, #415, #10391, #5410, #15723, #20869, #244, #5914, #8481, #28743, #5748, #31317, #10901, #28909, #31651, #18298, #10730, #21374, #29412, #16391, #21536, #5239, #26844, #15889, #10560, #18638, #16060, #26515, #2834, #21039, #31818, #21207, #16229, #31984, #26178, #13131, #7979, #29075, #5579, #11896, #3835, #21707, #32814, #32153, #11392, #16886, #22204, #9145, #29911, #1074, #14310, #6069, #19463, #8646, #19131, #32480, #8981, #13973, #27349, #29568, #24278, #8810, #746, #6414, #24765, #17225, #24600, #22367, #16552, #11554, #1243, #21869, #11231, #19628, #24436, #11721, #24933, #22036, #27177, #4175, #4003, #14476, #32651, #913, #30073, #6579, #27005, #1418, #17054, #32319, #6745, #14144, #27515, #19293, #29736, #6241, #9307, #19792, #30240, #27685, #3503, #16722, #3670, #4342, #31110, #9835, #27860, #22532, #1754, #20312, #12234, #25108, #7431, #32982, #17918, #9486, #33689, #10187, #30762, #7252, #20670, #7604, #28370, #30938, #28198, #19969, #17739, #25282, #22709, #1933, #12411, #4685, #22881, #12061, #30415, #1584, #15164, #25458, #18084, #15338, #20144, #6914, #28532, #14816, #25630, #4513, #2109, #33338, #12582, #23052, #17396, #33160, #33511, #9663, #10016, #30588, #20487, #4858, #14649, #25793, #7084, #2282, #12757, #23229, #17568, #14987, #28026, #28704, #2795, #23568, #21169, #13610, #24075, #32, #26642, #18428, #13438, #25964, #5027, #7771, #2458, #26135, #5202, #2632, #8109, #26306, #13261, #23737, #15512, #201, #23401, #15685, #21497, #10688, #18258, #12924, #13094, #31612, #10522, #33861, #31777, #10355, #8269, #20833, #540, #11028, #18596, #29036, #31945, #8437, #18761, #21336, #5539, #31278, #16020, #20999, #31448, #26474, #2968, #23904, #376, #7941, #28873, #5369, #10862, #15850, #18927, #5710, #29205, #16189, #3137, #8608, #6371, #19253, #11514, #6199, #21994, #16679, #24236, #13766, #32442, #26806, #16849, #19091, #8943, #27306, #24891, #3796, #29529, #1201 ),
 ( #26963, #19421, #22166, #3630, #14436, #29871, #19588, #30036, #29373, #6032, #32775, #32108, #13934, #14269, #32609, #16511, #24726, #9269, #8770, #11682, #9107, #21832, #6541, #3301, #17013, #5872, #873, #11193, #16351, #29693, #1377, #3962, #707, #27474, #21664, #11851, #24398, #27136, #3464, #14104, #22330, #11353, #32277, #24560, #1034, #4812, #4299, #30546, #12367, #7042, #14607, #4132, #1890, #17186, #30718, #9438, #22835, #7213, #15291, #17696, #19925, #25585, #2065, #12541, #33295, #20100, #4472, #30371, #17525, #14774, #9795, #28323, #25751, #25239, #7388, #33116, #28156, #6703, #19753, #22489, #27644, #25063, #1544, #27985, #14946, #6872, #20271, #12020, #30201, #1714, #32940, #25412, #4642, #12710, #15121, #17872, #17352, #23012, #33467, #27815, #12192, #9967, #22663, #20442, #30893, #2235, #9619, #33644, #23181, #331, #2750, #33818, #18382, #28995, #15466, #10817, #18550, #20790, #26600, #33983, #5495, #31235, #10312, #7727, #13214, #31404, #7898, #28828, #20623, #5326, #28488, #18215, #3097, #15806, #23357, #18044, #28659, #26262, #5155, #31065, #2923, #4985, #13392, #25919, #29158, #5664, #23691, #156, #16147, #13568, #23864, #26430, #10647, #2414, #21124, #15640, #26091, #31567, #8065, #15974, #21297, #7559, #12881, #2588, #31737, #20955, #24031, #8228, #13052, #23524, #10141, #10477, #18722, #24362, #16641, #3923, #5994, #16311, #21457, #13895, #6501, #9069, #29330, #8898, #14397, #14061, #29490, #32239, #500, #832, #21953, #19549, #29997, #3756, #18881, #16974, #19051, #24195, #8732, #27095, #3588, #16470, #21624, #24523, #21791, #19382, #14230, #26767, #32402, #993, #11312, #11478, #22126, #29830, #31900, #27432, #8395, #32067, #6332, #16809, #27265, #6155, #19216, #24686, #3258, #29652, #8567, #1161, #11642, #5832, #32569, #10984, #13728, #665, #11153, #26925, #3423, #20233, #15557, #22796, #33073, #32896, #7171, #20057, #2503, #7002, #17484, #1504, #28577, #33906, #22449, #30159, #5073, #11981, #9395, #33251, #19879, #30332, #6829, #6664, #4259, #12326, #10397, #9229, #26011, #22291, #30501, #31324, #17311, #9747, #25194, #4090, #12971, #18304, #9579, #1332, #14733, #30673, #27773, #14904, #18133, #27946, #20876, #4429, #23445, #7815, #24852, #14565, #28749, #27599, #1672, #5247, #11815, #25024, #32736, #19713, #12147, #25368, #17146, #22620, #1846, #23611, #5753, #26688, #5416, #21541, #31990, #8486, #29249, #16065, #420, #15895, #13486, #251, #31824, #24284, #753, #10736, #3347, #29080, #24118, #2679, #15729, #18472, #13137, #80, #10567, #23951, #10907, #26351, #18805, #21045, #26183, #21213, #31495, #21379, #8315, #8652, #26520, #13817, #7985, #3014, #16234, #2841, #28915, #585, #13310, #3184, #16397, #13653, #18643, #29574, #29418, #5920, #11076, #23784, #18973, #26850, #31658, #11237, #21713, #8154, #32159, #5585, #19137, #27183, #6248, #3676, #9151, #27355, #3840, #14315, #16559, #24770, #24442, #29743, #22537, #1248, #19299, #13979, #14150, #11727, #24606, #27012, #32820 ),
 ( #19633, #919, #22209, #16728, #1080, #32656, #30078, #6584, #17059, #3509, #11398, #21875, #27521, #16892, #32987, #6750, #11560, #32325, #25114, #22042, #4008, #29918, #14482, #24938, #1423, #11901, #8816, #32486, #22373, #8988, #9312, #19469, #19797, #30245, #1589, #6420, #17230, #12066, #27690, #4180, #14654, #9491, #19974, #6075, #7257, #25287, #14822, #12587, #27865, #7440, #20149, #33517, #17924, #25970, #28375, #30593, #2288, #12762, #23235, #10021, #30768, #15169, #7089, #28204, #14994, #23057, #5033, #15518, #25464, #18090, #9841, #4863, #17401, #30420, #33165, #4347, #1759, #12239, #4690, #25635, #17573, #20493, #22715, #6919, #1939, #9668, #2114, #30943, #23406, #17744, #28537, #28031, #15344, #25798, #4519, #12417, #33694, #22887, #10196, #31116, #20676, #33344, #10360, #7609, #2463, #12929, #20319, #33867, #5716, #26140, #11033, #29210, #31453, #3308, #10694, #16194, #7946, #21004, #18434, #23910, #8114, #18601, #29041, #31283, #5544, #5207, #10527, #13772, #16025, #38, #28709, #28878, #26480, #5375, #7776, #13615, #15691, #24080, #2637, #5879, #16357, #2974, #13443, #26812, #24242, #546, #3142, #381, #13100, #10867, #15855, #26311, #21341, #31782, #8274, #18766, #18263, #23573, #2800, #26648, #31617, #713, #21502, #8443, #31950, #13267, #29380, #23742, #206, #18934, #20838, #21175, #16855, #22000, #24732, #26969, #6377, #8776, #27313, #27480, #8614, #11688, #8949, #11199, #1040, #17192, #29701, #22336, #6547, #1383, #9113, #19427, #19259, #3969, #3803, #32781, #14275, #1207, #21838, #14442, #19759, #6205, #16517, #24898, #32283, #16685, #19594, #27142, #3636, #14110, #3470, #24567, #32616, #30208, #29535, #11857, #19097, #22172, #27650, #11520, #30042, #32448, #24404, #9275, #4138, #29877, #21670, #17020, #6710, #14613, #25069, #32117, #6038, #13940, #880, #11360, #20448, #1550, #14779, #12715, #27821, #33121, #25590, #23017, #25244, #2070, #12026, #27990, #30723, #9972, #7047, #33472, #19930, #17701, #22495, #17529, #4304, #9446, #4477, #32945, #30376, #1719, #30898, #6877, #12546, #14952, #7218, #17357, #4647, #28329, #12198, #22669, #9624, #25418, #20105, #28161, #33300, #7392, #17877, #4817, #15127, #20276, #25756, #15296, #30551, #1896, #2240, #12372, #22840, #9800, #22277, #14049, #19201, #11628, #4245, #6815, #27083, #6649, #12132, #11799, #27252, #29983, #32229, #32556, #19700, #17296, #27757, #1491, #16628, #14719, #16794, #21941, #6488, #14379, #24838, #3744, #19371, #32720, #19535, #17130, #11965, #24510, #30145, #1316, #22112, #9216, #19864, #27586, #29640, #25179, #6143, #29815, #4075, #14550, #25009, #3910, #9055, #22436, #982, #27419, #6318, #32883, #9382, #3577, #30318, #16961, #8718, #1657, #11467, #14216, #32391, #8886, #24672, #1146, #30836, #30658, #4928, #17812, #33767, #4756, #15233, #33233, #25864, #31182, #20218, #27930, #2354, #9732, #7155, #20564, #17638, #28099, #4587, #4414, #2008, #10085, #7673, #6987, #12828, #20041, #28270, #28601, #15063, #31009, #22953 ),
 ( #18159, #2177, #23300, #10258, #22604, #12309, #26037, #25352, #25531, #7506, #15409, #22781, #17990, #2531, #12484, #25696, #20740, #33411, #5100, #30486, #12650, #33058, #9908, #17470, #23120, #20385, #9563, #7328, #15586, #33584, #14891, #28437, #1831, #29272, #99, #5606, #13838, #32012, #2862, #26203, #16421, #10588, #8338, #21236, #13509, #8172, #23972, #18663, #2697, #15748, #442, #28770, #18828, #21066, #10925, #5774, #26873, #16254, #31515, #3207, #13675, #24139, #21399, #31679, #16088, #8009, #29101, #15917, #31845, #5940, #3368, #26373, #18995, #10758, #26710, #18324, #31343, #18494, #5266, #13157, #23632, #26541, #3036, #28937, #606, #5436, #7835, #13332, #23806, #11098, #21567, #24305, #8507, #29439, #271, #779, #11261, #8840, #21737, #6605, #21896, #27375, #22393, #22065, #24628, #1610, #1445, #11922, #14336, #11421, #29939, #17082, #27036, #32842, #30098, #32346, #4201, #11584, #27542, #19323, #29765, #6272, #24792, #9010, #19490, #6443, #32182, #16914, #6100, #16749, #14673, #3864, #941, #29598, #27207, #1271, #3698, #8677, #14504, #16581, #24963, #3531, #6771, #17252, #11751, #22232, #27712, #25133, #9333, #4029, #32676, #14171, #19656, #1101, #32509, #9172, #14003, #19819, #30271, #19159, #24465, #25819, #9514, #17764, #18108, #4541, #10041, #12438, #25309, #15365, #5054, #20338, #22556, #1964, #20517, #9689, #2133, #4883, #30788, #31137, #25654, #2309, #12782, #12088, #1781, #15538, #14843, #30613, #30963, #23255, #12259, #7461, #25990, #25485, #15190, #33718, #15014, #10215, #19995, #12608, #33009, #17591, #27885, #30443, #22908, #28557, #20695, #6941, #17944, #17424, #23077, #7109, #9861, #4368, #33365, #33538, #7628, #22736, #33186, #20170, #28053, #7281, #28223, #4710, #28394, #29060, #31475, #23593, #26500, #23762, #10886, #16215, #28730, #400, #5565, #15874, #2993, #24099, #16045, #33886, #11058, #10378, #58, #13465, #21361, #31804, #8135, #13287, #23932, #18285, #31636, #10546, #18624, #18786, #20856, #8295, #227, #2484, #26331, #8465, #21025, #13635, #29230, #26668, #5735, #3164, #567, #18453, #21523, #31971, #18954, #29399, #13119, #5899, #16378, #7967, #7795, #12952, #28895, #5398, #23425, #31302, #2657, #5226, #15708, #2819, #10715, #26164, #21194, #17038, #19448, #16539, #1058, #11706, #32138, #27498, #1226, #3490, #9291, #16706, #22189, #13959, #26991, #24422, #29894, #14130, #24586, #11538, #3327, #22021, #11218, #899, #19776, #32465, #6055, #11381, #32636, #26831, #1402, #733, #21856, #6395, #24750, #9130, #8966, #3653, #16871, #8633, #27333, #32303, #3820, #19612, #24265, #14293, #30058, #13797, #27161, #32798, #8796, #3987, #6563, #14460, #24917, #11878, #22351, #19279, #30226, #6726, #21692, #19117, #29721, #29555, #6227, #14800, #22515, #20941, #4326, #25265, #15627, #2216, #12695, #23165, #32966, #31053, #5139, #2738, #1568, #31390, #14631, #23344, #23678, #10126, #26078, #18030, #30397, #7880, #10633, #25904, #27668, #7545, #2574, #33627, #7713, #10463, #2398 ) ),
 .UNSPECIFIED., .T., .F., .T. ) 
 B_SPLINE_SURFACE_WITH_KNOTS ( ( 4, 3, 4 ),
 ( 3, 2, 2, 2, 2, 2, 2, 2, 2, 2, 2, 2, 2, 2, 2, 2, 2, 2, 2, 2, 2, 2, 2, 2, 2, 2, 2, 2, 2, 2, 2, 2, 2, 2, 2, 2, 2, 2, 2, 2, 2, 2, 2, 2, 2, 2, 2, 2, 2, 2, 2, 2, 2, 2, 2, 2, 2, 2, 2, 2, 2, 2, 2, 2, 2, 2, 2, 2, 2, 2, 2, 2, 2, 2, 2, 2, 2, 2, 2, 2, 2, 2, 2, 2, 2, 2, 2, 2, 2, 2, 2, 2, 2, 2, 2, 2, 2, 2, 2, 2, 2, 2, 2, 2, 2, 2, 2, 2, 2, 2, 2, 2, 2, 2, 2, 2, 2, 2, 2, 2, 2, 2, 2, 2, 2, 2, 2, 2, 2, 2, 2, 2, 2, 2, 2, 2, 2, 2, 2, 2, 2, 2, 2, 2, 2, 2, 2, 2, 2, 2, 2, 2, 2, 2, 2, 2, 2, 2, 2, 2, 2, 2, 2, 2, 2, 2, 2, 2, 2, 2, 2, 2, 2, 2, 2, 2, 2, 2, 2, 2, 2, 2, 2, 2, 2, 2, 2, 2, 2, 2, 2, 2, 3 ),
 ( 0.000000000000000000, 0.5000000000000000000, 1.000000000000000000 ),
 ( 0.000000000000000000, 0.005208333333333333044, 0.01041666666666666609, 0.01562500000000000000, 0.02083333333333333218, 0.02604166666666666782, 0.03125000000000000000, 0.03645833333333333565, 0.04166666666666666435, 0.04687500000000000000, 0.05208333333333333565, 0.05729166666666666435, 0.06250000000000000000, 0.06770833333333332871, 0.07291666666666667129, 0.07812500000000000000, 0.08333333333333332871, 0.08854166666666667129, 0.09375000000000000000, 0.09895833333333332871, 0.1041666666666666713, 0.1093750000000000000, 0.1145833333333333287, 0.1197916666666666713, 0.1250000000000000000, 0.1302083333333333426, 0.1354166666666666574, 0.1406250000000000000, 0.1458333333333333426, 0.1510416666666666574, 0.1562500000000000000, 0.1614583333333333426, 0.1666666666666666574, 0.1718750000000000000, 0.1770833333333333426, 0.1822916666666666574, 0.1875000000000000000, 0.1927083333333333426, 0.1979166666666666574, 0.2031250000000000000, 0.2083333333333333426, 0.2135416666666666574, 0.2187500000000000000, 0.2239583333333333426, 0.2291666666666666574, 0.2343750000000000000, 0.2395833333333333426, 0.2447916666666666574, 0.2500000000000000000, 0.2552083333333333148, 0.2604166666666666852, 0.2656250000000000000, 0.2708333333333333148, 0.2760416666666666852, 0.2812500000000000000, 0.2864583333333333148, 0.2916666666666666852, 0.2968750000000000000, 0.3020833333333333148, 0.3072916666666666852, 0.3125000000000000000, 0.3177083333333333148, 0.3229166666666666852, 0.3281250000000000000, 0.3333333333333333148, 0.3385416666666666852, 0.3437500000000000000, 0.3489583333333333148, 0.3541666666666666852, 0.3593750000000000000, 0.3645833333333333148, 0.3697916666666666852, 0.3750000000000000000, 0.3802083333333333148, 0.3854166666666666852, 0.3906250000000000000, 0.3958333333333333148, 0.4010416666666666852, 0.4062500000000000000, 0.4114583333333333148, 0.4166666666666666852, 0.4218750000000000000, 0.4270833333333333148, 0.4322916666666666852, 0.4375000000000000000, 0.4427083333333333148, 0.4479166666666666852, 0.4531250000000000000, 0.4583333333333333148, 0.4635416666666666852, 0.4687500000000000000, 0.4739583333333333148, 0.4791666666666666852, 0.4843750000000000000, 0.4895833333333333148, 0.4947916666666666852, 0.5000000000000000000, 0.5052083333333333703, 0.5104166666666666297, 0.5156250000000000000, 0.5208333333333333703, 0.5260416666666666297, 0.5312500000000000000, 0.5364583333333333703, 0.5416666666666666297, 0.5468750000000000000, 0.5520833333333333703, 0.5572916666666666297, 0.5625000000000000000, 0.5677083333333333703, 0.5729166666666666297, 0.5781250000000000000, 0.5833333333333333703, 0.5885416666666666297, 0.5937500000000000000, 0.5989583333333333703, 0.6041666666666666297, 0.6093750000000000000, 0.6145833333333333703, 0.6197916666666666297, 0.6250000000000000000, 0.6302083333333333703, 0.6354166666666666297, 0.6406250000000000000, 0.6458333333333333703, 0.6510416666666666297, 0.6562500000000000000, 0.6614583333333333703, 0.6666666666666666297, 0.6718750000000000000, 0.6770833333333333703, 0.6822916666666666297, 0.6875000000000000000, 0.6927083333333333703, 0.6979166666666666297, 0.7031250000000000000, 0.7083333333333333703, 0.7135416666666666297, 0.7187500000000000000, 0.7239583333333333703, 0.7291666666666666297, 0.7343750000000000000, 0.7395833333333333703, 0.7447916666666666297, 0.7500000000000000000, 0.7552083333333333703, 0.7604166666666666297, 0.7656250000000000000, 0.7708333333333333703, 0.7760416666666666297, 0.7812500000000000000, 0.7864583333333333703, 0.7916666666666666297, 0.7968750000000000000, 0.8020833333333333703, 0.8072916666666666297, 0.8125000000000000000, 0.8177083333333333703, 0.8229166666666666297, 0.8281250000000000000, 0.8333333333333333703, 0.8385416666666666297, 0.8437500000000000000, 0.8489583333333333703, 0.8541666666666666297, 0.8593750000000000000, 0.8645833333333333703, 0.8697916666666666297, 0.8750000000000000000, 0.8802083333333333703, 0.8854166666666666297, 0.8906250000000000000, 0.8958333333333333703, 0.9010416666666666297, 0.9062500000000000000, 0.9114583333333333703, 0.9166666666666666297, 0.9218750000000000000, 0.9270833333333333703, 0.9322916666666666297, 0.9375000000000000000, 0.9427083333333333703, 0.9479166666666666297, 0.9531250000000000000, 0.9583333333333333703, 0.9635416666666666297, 0.9687500000000000000, 0.9739583333333333703, 0.9791666666666666297, 0.9843750000000000000, 0.9895833333333333703, 0.9947916666666666297, 1.000000000000000000 ),
 .UNSPECIFIED. ) 
 GEOMETRIC_REPRESENTATION_ITEM ( )  RATIONAL_B_SPLINE_SURFACE ( (
 ( 1.000000000000000000, 0.9659258262890683122, 1.000000000000000000, 0.9659258262890683122, 1.000000000000000000, 0.9659258262890683122, 1.000000000000000000, 0.9659258262890683122, 1.000000000000000000, 0.9659258262890683122, 1.000000000000000000, 0.9659258262890683122, 1.000000000000000000, 0.9659258262890683122, 1.000000000000000000, 0.9659258262890683122, 1.000000000000000000, 0.9659258262890683122, 1.000000000000000000, 0.9659258262890683122, 1.000000000000000000, 0.9659258262890683122, 1.000000000000000000, 0.9659258262890683122, 1.000000000000000000, 0.9659258262890683122, 1.000000000000000000, 0.9659258262890683122, 1.000000000000000000, 0.9659258262890683122, 1.000000000000000000, 0.9659258262890683122, 1.000000000000000000, 0.9659258262890683122, 1.000000000000000000, 0.9659258262890683122, 1.000000000000000000, 0.9659258262890683122, 1.000000000000000000, 0.9659258262890683122, 1.000000000000000000, 0.9659258262890683122, 1.000000000000000000, 0.9659258262890683122, 1.000000000000000000, 0.9659258262890683122, 1.000000000000000000, 0.9659258262890683122, 1.000000000000000000, 0.9659258262890683122, 1.000000000000000000, 0.9659258262890683122, 1.000000000000000000, 0.9659258262890683122, 1.000000000000000000, 0.9659258262890683122, 1.000000000000000000, 0.9659258262890683122, 1.000000000000000000, 0.9659258262890683122, 1.000000000000000000, 0.9659258262890683122, 1.000000000000000000, 0.9659258262890683122, 1.000000000000000000, 0.9659258262890683122, 1.000000000000000000, 0.9659258262890683122, 1.000000000000000000, 0.9659258262890683122, 1.000000000000000000, 0.9659258262890683122, 1.000000000000000000, 0.9659258262890683122, 1.000000000000000000, 0.9659258262890683122, 1.000000000000000000, 0.9659258262890683122, 1.000000000000000000, 0.9659258262890683122, 1.000000000000000000, 0.9659258262890683122, 1.000000000000000000, 0.9659258262890683122, 1.000000000000000000, 0.9659258262890683122, 1.000000000000000000, 0.9659258262890683122, 1.000000000000000000, 0.9659258262890683122, 1.000000000000000000, 0.9659258262890683122, 1.000000000000000000, 0.9659258262890683122, 1.000000000000000000, 0.9659258262890683122, 1.000000000000000000, 0.9659258262890683122, 1.000000000000000000, 0.9659258262890683122, 1.000000000000000000, 0.9659258262890683122, 1.000000000000000000, 0.9659258262890683122, 1.000000000000000000, 0.9659258262890683122, 1.000000000000000000, 0.9659258262890683122, 1.000000000000000000, 0.9659258262890683122, 1.000000000000000000, 0.9659258262890683122, 1.000000000000000000, 0.9659258262890683122, 1.000000000000000000, 0.9659258262890683122, 1.000000000000000000, 0.9659258262890683122, 1.000000000000000000, 0.9659258262890683122, 1.000000000000000000, 0.9659258262890683122, 1.000000000000000000, 0.9659258262890683122, 1.000000000000000000, 0.9659258262890683122, 1.000000000000000000, 0.9659258262890683122, 1.000000000000000000, 0.9659258262890683122, 1.000000000000000000, 0.9659258262890683122, 1.000000000000000000, 0.9659258262890683122, 1.000000000000000000, 0.9659258262890683122, 1.000000000000000000, 0.9659258262890683122, 1.000000000000000000, 0.9659258262890683122, 1.000000000000000000, 0.9659258262890683122, 1.000000000000000000, 0.9659258262890683122, 1.000000000000000000, 0.9659258262890683122, 1.000000000000000000, 0.9659258262890683122, 1.000000000000000000, 0.9659258262890683122, 1.000000000000000000, 0.9659258262890683122, 1.000000000000000000, 0.9659258262890683122, 1.000000000000000000, 0.9659258262890683122, 1.000000000000000000, 0.9659258262890683122, 1.000000000000000000, 0.9659258262890683122, 1.000000000000000000, 0.9659258262890683122, 1.000000000000000000, 0.9659258262890683122, 1.000000000000000000, 0.9659258262890683122, 1.000000000000000000, 0.9659258262890683122, 1.000000000000000000, 0.9659258262890683122, 1.000000000000000000, 0.9659258262890683122, 1.000000000000000000, 0.9659258262890683122, 1.000000000000000000, 0.9659258262890683122, 1.000000000000000000, 0.9659258262890683122, 1.000000000000000000, 0.9659258262890683122, 1.000000000000000000, 0.9659258262890683122, 1.000000000000000000, 0.9659258262890683122, 1.000000000000000000, 0.9659258262890683122, 1.000000000000000000, 0.9659258262890683122, 1.000000000000000000, 0.9659258262890683122, 1.000000000000000000, 0.9659258262890683122, 1.000000000000000000, 0.9659258262890683122, 1.000000000000000000, 0.9659258262890683122, 1.000000000000000000, 0.9659258262890683122, 1.000000000000000000, 0.9659258262890683122, 1.000000000000000000, 0.9659258262890683122, 1.000000000000000000, 0.9659258262890683122, 1.000000000000000000, 0.9659258262890683122, 1.000000000000000000, 0.9659258262890683122, 1.000000000000000000, 0.9659258262890683122, 1.000000000000000000, 0.9659258262890683122, 1.000000000000000000, 0.9659258262890683122, 1.000000000000000000, 0.9659258262890683122, 1.000000000000000000, 0.9659258262890683122, 1.000000000000000000, 0.9659258262890683122, 1.000000000000000000, 0.9659258262890683122, 1.000000000000000000, 0.9659258262890683122, 1.000000000000000000, 0.9659258262890683122, 1.000000000000000000, 0.9659258262890683122, 1.000000000000000000, 0.9659258262890683122, 1.000000000000000000, 0.9659258262890683122, 1.000000000000000000, 0.9659258262890683122, 1.000000000000000000, 0.9659258262890683122, 1.000000000000000000, 0.9659258262890683122, 1.000000000000000000, 0.9659258262890683122, 1.000000000000000000, 0.9659258262890683122, 1.000000000000000000, 0.9659258262890683122, 1.000000000000000000, 0.9659258262890683122, 1.000000000000000000, 0.9659258262890683122, 1.000000000000000000, 0.9659258262890683122, 1.000000000000000000, 0.9659258262890683122, 1.000000000000000000, 0.9659258262890683122, 1.000000000000000000, 0.9659258262890683122, 1.000000000000000000, 0.9659258262890683122, 1.000000000000000000, 0.9659258262890683122, 1.000000000000000000, 0.9659258262890683122, 1.000000000000000000, 0.9659258262890683122, 1.000000000000000000, 0.9659258262890683122, 1.000000000000000000, 0.9659258262890683122, 1.000000000000000000, 0.9659258262890683122, 1.000000000000000000, 0.9659258262890683122, 1.000000000000000000, 0.9659258262890683122, 1.000000000000000000, 0.9659258262890683122, 1.000000000000000000, 0.9659258262890683122, 1.000000000000000000, 0.9659258262890683122, 1.000000000000000000, 0.9659258262890683122, 1.000000000000000000, 0.9659258262890683122, 1.000000000000000000, 0.9659258262890683122, 1.000000000000000000, 0.9659258262890683122, 1.000000000000000000, 0.9659258262890683122, 1.000000000000000000, 0.9659258262890683122, 1.000000000000000000, 0.9659258262890683122, 1.000000000000000000, 0.9659258262890683122, 1.000000000000000000, 0.9659258262890683122, 1.000000000000000000, 0.9659258262890683122, 1.000000000000000000, 0.9659258262890683122, 1.000000000000000000, 0.9659258262890683122, 1.000000000000000000, 0.9659258262890683122, 1.000000000000000000, 0.9659258262890683122, 1.000000000000000000, 0.9659258262890683122, 1.000000000000000000, 0.9659258262890683122, 1.000000000000000000, 0.9659258262890683122, 1.000000000000000000, 0.9659258262890683122, 1.000000000000000000, 0.9659258262890683122, 1.000000000000000000, 0.9659258262890683122, 1.000000000000000000, 0.9659258262890683122, 1.000000000000000000, 0.9659258262890683122, 1.000000000000000000, 0.9659258262890683122, 1.000000000000000000, 0.9659258262890683122, 1.000000000000000000, 0.9659258262890683122, 1.000000000000000000, 0.9659258262890683122, 1.000000000000000000, 0.9659258262890683122, 1.000000000000000000, 0.9659258262890683122, 1.000000000000000000, 0.9659258262890683122, 1.000000000000000000, 0.9659258262890683122, 1.000000000000000000, 0.9659258262890683122, 1.000000000000000000, 0.9659258262890683122, 1.000000000000000000, 0.9659258262890683122, 1.000000000000000000, 0.9659258262890683122, 1.000000000000000000, 0.9659258262890683122, 1.000000000000000000, 0.9659258262890683122, 1.000000000000000000, 0.9659258262890683122, 1.000000000000000000, 0.9659258262890683122, 1.000000000000000000, 0.9659258262890683122, 1.000000000000000000, 0.9659258262890683122, 1.000000000000000000, 0.9659258262890683122, 1.000000000000000000, 0.9659258262890683122, 1.000000000000000000, 0.9659258262890683122, 1.000000000000000000, 0.9659258262890683122, 1.000000000000000000, 0.9659258262890683122, 1.000000000000000000, 0.9659258262890683122, 1.000000000000000000, 0.9659258262890683122, 1.000000000000000000, 0.9659258262890683122, 1.000000000000000000, 0.9659258262890683122, 1.000000000000000000, 0.9659258262890683122, 1.000000000000000000, 0.9659258262890683122, 1.000000000000000000, 0.9659258262890683122, 1.000000000000000000),
 ( 0.3333333333333333703, 0.3219752754296894559, 0.3333333333333333703, 0.3219752754296894559, 0.3333333333333333703, 0.3219752754296894559, 0.3333333333333333703, 0.3219752754296894559, 0.3333333333333333703, 0.3219752754296894559, 0.3333333333333333703, 0.3219752754296894559, 0.3333333333333333703, 0.3219752754296894559, 0.3333333333333333703, 0.3219752754296894559, 0.3333333333333333703, 0.3219752754296894559, 0.3333333333333333703, 0.3219752754296894559, 0.3333333333333333703, 0.3219752754296894559, 0.3333333333333333703, 0.3219752754296894559, 0.3333333333333333703, 0.3219752754296894559, 0.3333333333333333703, 0.3219752754296894559, 0.3333333333333333703, 0.3219752754296894559, 0.3333333333333333703, 0.3219752754296894559, 0.3333333333333333703, 0.3219752754296894559, 0.3333333333333333703, 0.3219752754296894559, 0.3333333333333333703, 0.3219752754296894559, 0.3333333333333333703, 0.3219752754296894559, 0.3333333333333333703, 0.3219752754296894559, 0.3333333333333333703, 0.3219752754296894559, 0.3333333333333333703, 0.3219752754296894559, 0.3333333333333333703, 0.3219752754296894559, 0.3333333333333333703, 0.3219752754296894559, 0.3333333333333333703, 0.3219752754296894559, 0.3333333333333333703, 0.3219752754296894559, 0.3333333333333333703, 0.3219752754296894559, 0.3333333333333333703, 0.3219752754296894559, 0.3333333333333333703, 0.3219752754296894559, 0.3333333333333333703, 0.3219752754296894559, 0.3333333333333333703, 0.3219752754296894559, 0.3333333333333333703, 0.3219752754296894559, 0.3333333333333333703, 0.3219752754296894559, 0.3333333333333333703, 0.3219752754296894559, 0.3333333333333333703, 0.3219752754296894559, 0.3333333333333333703, 0.3219752754296894559, 0.3333333333333333703, 0.3219752754296894559, 0.3333333333333333703, 0.3219752754296894559, 0.3333333333333333703, 0.3219752754296894559, 0.3333333333333333703, 0.3219752754296894559, 0.3333333333333333703, 0.3219752754296894559, 0.3333333333333333703, 0.3219752754296894559, 0.3333333333333333703, 0.3219752754296894559, 0.3333333333333333703, 0.3219752754296894559, 0.3333333333333333703, 0.3219752754296894559, 0.3333333333333333703, 0.3219752754296894559, 0.3333333333333333703, 0.3219752754296894559, 0.3333333333333333703, 0.3219752754296894559, 0.3333333333333333703, 0.3219752754296894559, 0.3333333333333333703, 0.3219752754296894559, 0.3333333333333333703, 0.3219752754296894559, 0.3333333333333333703, 0.3219752754296894559, 0.3333333333333333703, 0.3219752754296894559, 0.3333333333333333703, 0.3219752754296894559, 0.3333333333333333703, 0.3219752754296894559, 0.3333333333333333703, 0.3219752754296894559, 0.3333333333333333703, 0.3219752754296894559, 0.3333333333333333703, 0.3219752754296894559, 0.3333333333333333703, 0.3219752754296894559, 0.3333333333333333703, 0.3219752754296894559, 0.3333333333333333703, 0.3219752754296894559, 0.3333333333333333703, 0.3219752754296894559, 0.3333333333333333703, 0.3219752754296894559, 0.3333333333333333703, 0.3219752754296894559, 0.3333333333333333703, 0.3219752754296894559, 0.3333333333333333703, 0.3219752754296894559, 0.3333333333333333703, 0.3219752754296894559, 0.3333333333333333703, 0.3219752754296894559, 0.3333333333333333703, 0.3219752754296894559, 0.3333333333333333703, 0.3219752754296894559, 0.3333333333333333703, 0.3219752754296894559, 0.3333333333333333703, 0.3219752754296894559, 0.3333333333333333703, 0.3219752754296894559, 0.3333333333333333703, 0.3219752754296894559, 0.3333333333333333703, 0.3219752754296894559, 0.3333333333333333703, 0.3219752754296894559, 0.3333333333333333703, 0.3219752754296894559, 0.3333333333333333703, 0.3219752754296894559, 0.3333333333333333703, 0.3219752754296894559, 0.3333333333333333703, 0.3219752754296894559, 0.3333333333333333703, 0.3219752754296894559, 0.3333333333333333703, 0.3219752754296894559, 0.3333333333333333703, 0.3219752754296894559, 0.3333333333333333703, 0.3219752754296894559, 0.3333333333333333703, 0.3219752754296894559, 0.3333333333333333703, 0.3219752754296894559, 0.3333333333333333703, 0.3219752754296894559, 0.3333333333333333703, 0.3219752754296894559, 0.3333333333333333703, 0.3219752754296894559, 0.3333333333333333703, 0.3219752754296894559, 0.3333333333333333703, 0.3219752754296894559, 0.3333333333333333703, 0.3219752754296894559, 0.3333333333333333703, 0.3219752754296894559, 0.3333333333333333703, 0.3219752754296894559, 0.3333333333333333703, 0.3219752754296894559, 0.3333333333333333703, 0.3219752754296894559, 0.3333333333333333703, 0.3219752754296894559, 0.3333333333333333703, 0.3219752754296894559, 0.3333333333333333703, 0.3219752754296894559, 0.3333333333333333703, 0.3219752754296894559, 0.3333333333333333703, 0.3219752754296894559, 0.3333333333333333703, 0.3219752754296894559, 0.3333333333333333703, 0.3219752754296894559, 0.3333333333333333703, 0.3219752754296894559, 0.3333333333333333703, 0.3219752754296894559, 0.3333333333333333703, 0.3219752754296894559, 0.3333333333333333703, 0.3219752754296894559, 0.3333333333333333703, 0.3219752754296894559, 0.3333333333333333703, 0.3219752754296894559, 0.3333333333333333703, 0.3219752754296894559, 0.3333333333333333703, 0.3219752754296894559, 0.3333333333333333703, 0.3219752754296894559, 0.3333333333333333703, 0.3219752754296894559, 0.3333333333333333703, 0.3219752754296894559, 0.3333333333333333703, 0.3219752754296894559, 0.3333333333333333703, 0.3219752754296894559, 0.3333333333333333703, 0.3219752754296894559, 0.3333333333333333703, 0.3219752754296894559, 0.3333333333333333703, 0.3219752754296894559, 0.3333333333333333703, 0.3219752754296894559, 0.3333333333333333703, 0.3219752754296894559, 0.3333333333333333703, 0.3219752754296894559, 0.3333333333333333703, 0.3219752754296894559, 0.3333333333333333703, 0.3219752754296894559, 0.3333333333333333703, 0.3219752754296894559, 0.3333333333333333703, 0.3219752754296894559, 0.3333333333333333703, 0.3219752754296894559, 0.3333333333333333703, 0.3219752754296894559, 0.3333333333333333703, 0.3219752754296894559, 0.3333333333333333703, 0.3219752754296894559, 0.3333333333333333703, 0.3219752754296894559, 0.3333333333333333703, 0.3219752754296894559, 0.3333333333333333703, 0.3219752754296894559, 0.3333333333333333703, 0.3219752754296894559, 0.3333333333333333703, 0.3219752754296894559, 0.3333333333333333703, 0.3219752754296894559, 0.3333333333333333703, 0.3219752754296894559, 0.3333333333333333703, 0.3219752754296894559, 0.3333333333333333703, 0.3219752754296894559, 0.3333333333333333703, 0.3219752754296894559, 0.3333333333333333703, 0.3219752754296894559, 0.3333333333333333703, 0.3219752754296894559, 0.3333333333333333703, 0.3219752754296894559, 0.3333333333333333703, 0.3219752754296894559, 0.3333333333333333703, 0.3219752754296894559, 0.3333333333333333703, 0.3219752754296894559, 0.3333333333333333703, 0.3219752754296894559, 0.3333333333333333703, 0.3219752754296894559, 0.3333333333333333703, 0.3219752754296894559, 0.3333333333333333703, 0.3219752754296894559, 0.3333333333333333703, 0.3219752754296894559, 0.3333333333333333703, 0.3219752754296894559, 0.3333333333333333703, 0.3219752754296894559, 0.3333333333333333703, 0.3219752754296894559, 0.3333333333333333703, 0.3219752754296894559, 0.3333333333333333703, 0.3219752754296894559, 0.3333333333333333703, 0.3219752754296894559, 0.3333333333333333703, 0.3219752754296894559, 0.3333333333333333703, 0.3219752754296894559, 0.3333333333333333703, 0.3219752754296894559, 0.3333333333333333703, 0.3219752754296894559, 0.3333333333333333703, 0.3219752754296894559, 0.3333333333333333703, 0.3219752754296894559, 0.3333333333333333703, 0.3219752754296894559, 0.3333333333333333703, 0.3219752754296894559, 0.3333333333333333703, 0.3219752754296894559, 0.3333333333333333703, 0.3219752754296894559, 0.3333333333333333703, 0.3219752754296894559, 0.3333333333333333703, 0.3219752754296894559, 0.3333333333333333703, 0.3219752754296894559, 0.3333333333333333703, 0.3219752754296894559, 0.3333333333333333703, 0.3219752754296894559, 0.3333333333333333703, 0.3219752754296894559, 0.3333333333333333703, 0.3219752754296894559, 0.3333333333333333703, 0.3219752754296894559, 0.3333333333333333703, 0.3219752754296894559, 0.3333333333333333703, 0.3219752754296894559, 0.3333333333333333703, 0.3219752754296894559, 0.3333333333333333703, 0.3219752754296894559, 0.3333333333333333703, 0.3219752754296894559, 0.3333333333333333703, 0.3219752754296894559, 0.3333333333333333703, 0.3219752754296894559, 0.3333333333333333703, 0.3219752754296894559, 0.3333333333333333703, 0.3219752754296894559, 0.3333333333333333703, 0.3219752754296894559, 0.3333333333333333703, 0.3219752754296894559, 0.3333333333333333703, 0.3219752754296894559, 0.3333333333333333703, 0.3219752754296894559, 0.3333333333333333703, 0.3219752754296894559, 0.3333333333333333703, 0.3219752754296894559, 0.3333333333333333703, 0.3219752754296894559, 0.3333333333333333703),
 ( 0.3333333333333333703, 0.3219752754296894559, 0.3333333333333333703, 0.3219752754296894559, 0.3333333333333333703, 0.3219752754296894559, 0.3333333333333333703, 0.3219752754296894559, 0.3333333333333333703, 0.3219752754296894559, 0.3333333333333333703, 0.3219752754296894559, 0.3333333333333333703, 0.3219752754296894559, 0.3333333333333333703, 0.3219752754296894559, 0.3333333333333333703, 0.3219752754296894559, 0.3333333333333333703, 0.3219752754296894559, 0.3333333333333333703, 0.3219752754296894559, 0.3333333333333333703, 0.3219752754296894559, 0.3333333333333333703, 0.3219752754296894559, 0.3333333333333333703, 0.3219752754296894559, 0.3333333333333333703, 0.3219752754296894559, 0.3333333333333333703, 0.3219752754296894559, 0.3333333333333333703, 0.3219752754296894559, 0.3333333333333333703, 0.3219752754296894559, 0.3333333333333333703, 0.3219752754296894559, 0.3333333333333333703, 0.3219752754296894559, 0.3333333333333333703, 0.3219752754296894559, 0.3333333333333333703, 0.3219752754296894559, 0.3333333333333333703, 0.3219752754296894559, 0.3333333333333333703, 0.3219752754296894559, 0.3333333333333333703, 0.3219752754296894559, 0.3333333333333333703, 0.3219752754296894559, 0.3333333333333333703, 0.3219752754296894559, 0.3333333333333333703, 0.3219752754296894559, 0.3333333333333333703, 0.3219752754296894559, 0.3333333333333333703, 0.3219752754296894559, 0.3333333333333333703, 0.3219752754296894559, 0.3333333333333333703, 0.3219752754296894559, 0.3333333333333333703, 0.3219752754296894559, 0.3333333333333333703, 0.3219752754296894559, 0.3333333333333333703, 0.3219752754296894559, 0.3333333333333333703, 0.3219752754296894559, 0.3333333333333333703, 0.3219752754296894559, 0.3333333333333333703, 0.3219752754296894559, 0.3333333333333333703, 0.3219752754296894559, 0.3333333333333333703, 0.3219752754296894559, 0.3333333333333333703, 0.3219752754296894559, 0.3333333333333333703, 0.3219752754296894559, 0.3333333333333333703, 0.3219752754296894559, 0.3333333333333333703, 0.3219752754296894559, 0.3333333333333333703, 0.3219752754296894559, 0.3333333333333333703, 0.3219752754296894559, 0.3333333333333333703, 0.3219752754296894559, 0.3333333333333333703, 0.3219752754296894559, 0.3333333333333333703, 0.3219752754296894559, 0.3333333333333333703, 0.3219752754296894559, 0.3333333333333333703, 0.3219752754296894559, 0.3333333333333333703, 0.3219752754296894559, 0.3333333333333333703, 0.3219752754296894559, 0.3333333333333333703, 0.3219752754296894559, 0.3333333333333333703, 0.3219752754296894559, 0.3333333333333333703, 0.3219752754296894559, 0.3333333333333333703, 0.3219752754296894559, 0.3333333333333333703, 0.3219752754296894559, 0.3333333333333333703, 0.3219752754296894559, 0.3333333333333333703, 0.3219752754296894559, 0.3333333333333333703, 0.3219752754296894559, 0.3333333333333333703, 0.3219752754296894559, 0.3333333333333333703, 0.3219752754296894559, 0.3333333333333333703, 0.3219752754296894559, 0.3333333333333333703, 0.3219752754296894559, 0.3333333333333333703, 0.3219752754296894559, 0.3333333333333333703, 0.3219752754296894559, 0.3333333333333333703, 0.3219752754296894559, 0.3333333333333333703, 0.3219752754296894559, 0.3333333333333333703, 0.3219752754296894559, 0.3333333333333333703, 0.3219752754296894559, 0.3333333333333333703, 0.3219752754296894559, 0.3333333333333333703, 0.3219752754296894559, 0.3333333333333333703, 0.3219752754296894559, 0.3333333333333333703, 0.3219752754296894559, 0.3333333333333333703, 0.3219752754296894559, 0.3333333333333333703, 0.3219752754296894559, 0.3333333333333333703, 0.3219752754296894559, 0.3333333333333333703, 0.3219752754296894559, 0.3333333333333333703, 0.3219752754296894559, 0.3333333333333333703, 0.3219752754296894559, 0.3333333333333333703, 0.3219752754296894559, 0.3333333333333333703, 0.3219752754296894559, 0.3333333333333333703, 0.3219752754296894559, 0.3333333333333333703, 0.3219752754296894559, 0.3333333333333333703, 0.3219752754296894559, 0.3333333333333333703, 0.3219752754296894559, 0.3333333333333333703, 0.3219752754296894559, 0.3333333333333333703, 0.3219752754296894559, 0.3333333333333333703, 0.3219752754296894559, 0.3333333333333333703, 0.3219752754296894559, 0.3333333333333333703, 0.3219752754296894559, 0.3333333333333333703, 0.3219752754296894559, 0.3333333333333333703, 0.3219752754296894559, 0.3333333333333333703, 0.3219752754296894559, 0.3333333333333333703, 0.3219752754296894559, 0.3333333333333333703, 0.3219752754296894559, 0.3333333333333333703, 0.3219752754296894559, 0.3333333333333333703, 0.3219752754296894559, 0.3333333333333333703, 0.3219752754296894559, 0.3333333333333333703, 0.3219752754296894559, 0.3333333333333333703, 0.3219752754296894559, 0.3333333333333333703, 0.3219752754296894559, 0.3333333333333333703, 0.3219752754296894559, 0.3333333333333333703, 0.3219752754296894559, 0.3333333333333333703, 0.3219752754296894559, 0.3333333333333333703, 0.3219752754296894559, 0.3333333333333333703, 0.3219752754296894559, 0.3333333333333333703, 0.3219752754296894559, 0.3333333333333333703, 0.3219752754296894559, 0.3333333333333333703, 0.3219752754296894559, 0.3333333333333333703, 0.3219752754296894559, 0.3333333333333333703, 0.3219752754296894559, 0.3333333333333333703, 0.3219752754296894559, 0.3333333333333333703, 0.3219752754296894559, 0.3333333333333333703, 0.3219752754296894559, 0.3333333333333333703, 0.3219752754296894559, 0.3333333333333333703, 0.3219752754296894559, 0.3333333333333333703, 0.3219752754296894559, 0.3333333333333333703, 0.3219752754296894559, 0.3333333333333333703, 0.3219752754296894559, 0.3333333333333333703, 0.3219752754296894559, 0.3333333333333333703, 0.3219752754296894559, 0.3333333333333333703, 0.3219752754296894559, 0.3333333333333333703, 0.3219752754296894559, 0.3333333333333333703, 0.3219752754296894559, 0.3333333333333333703, 0.3219752754296894559, 0.3333333333333333703, 0.3219752754296894559, 0.3333333333333333703, 0.3219752754296894559, 0.3333333333333333703, 0.3219752754296894559, 0.3333333333333333703, 0.3219752754296894559, 0.3333333333333333703, 0.3219752754296894559, 0.3333333333333333703, 0.3219752754296894559, 0.3333333333333333703, 0.3219752754296894559, 0.3333333333333333703, 0.3219752754296894559, 0.3333333333333333703, 0.3219752754296894559, 0.3333333333333333703, 0.3219752754296894559, 0.3333333333333333703, 0.3219752754296894559, 0.3333333333333333703, 0.3219752754296894559, 0.3333333333333333703, 0.3219752754296894559, 0.3333333333333333703, 0.3219752754296894559, 0.3333333333333333703, 0.3219752754296894559, 0.3333333333333333703, 0.3219752754296894559, 0.3333333333333333703, 0.3219752754296894559, 0.3333333333333333703, 0.3219752754296894559, 0.3333333333333333703, 0.3219752754296894559, 0.3333333333333333703, 0.3219752754296894559, 0.3333333333333333703, 0.3219752754296894559, 0.3333333333333333703, 0.3219752754296894559, 0.3333333333333333703, 0.3219752754296894559, 0.3333333333333333703, 0.3219752754296894559, 0.3333333333333333703, 0.3219752754296894559, 0.3333333333333333703, 0.3219752754296894559, 0.3333333333333333703, 0.3219752754296894559, 0.3333333333333333703, 0.3219752754296894559, 0.3333333333333333703, 0.3219752754296894559, 0.3333333333333333703, 0.3219752754296894559, 0.3333333333333333703, 0.3219752754296894559, 0.3333333333333333703, 0.3219752754296894559, 0.3333333333333333703, 0.3219752754296894559, 0.3333333333333333703, 0.3219752754296894559, 0.3333333333333333703, 0.3219752754296894559, 0.3333333333333333703, 0.3219752754296894559, 0.3333333333333333703, 0.3219752754296894559, 0.3333333333333333703, 0.3219752754296894559, 0.3333333333333333703, 0.3219752754296894559, 0.3333333333333333703, 0.3219752754296894559, 0.3333333333333333703, 0.3219752754296894559, 0.3333333333333333703, 0.3219752754296894559, 0.3333333333333333703, 0.3219752754296894559, 0.3333333333333333703, 0.3219752754296894559, 0.3333333333333333703, 0.3219752754296894559, 0.3333333333333333703, 0.3219752754296894559, 0.3333333333333333703, 0.3219752754296894559, 0.3333333333333333703, 0.3219752754296894559, 0.3333333333333333703, 0.3219752754296894559, 0.3333333333333333703, 0.3219752754296894559, 0.3333333333333333703, 0.3219752754296894559, 0.3333333333333333703, 0.3219752754296894559, 0.3333333333333333703, 0.3219752754296894559, 0.3333333333333333703, 0.3219752754296894559, 0.3333333333333333703, 0.3219752754296894559, 0.3333333333333333703, 0.3219752754296894559, 0.3333333333333333703, 0.3219752754296894559, 0.3333333333333333703, 0.3219752754296894559, 0.3333333333333333703, 0.3219752754296894559, 0.3333333333333333703, 0.3219752754296894559, 0.3333333333333333703, 0.3219752754296894559, 0.3333333333333333703, 0.3219752754296894559, 0.3333333333333333703, 0.3219752754296894559, 0.3333333333333333703, 0.3219752754296894559, 0.3333333333333333703, 0.3219752754296894559, 0.3333333333333333703),
 ( 1.000000000000000000, 0.9659258262890683122, 1.000000000000000000, 0.9659258262890683122, 1.000000000000000000, 0.9659258262890683122, 1.000000000000000000, 0.9659258262890683122, 1.000000000000000000, 0.9659258262890683122, 1.000000000000000000, 0.9659258262890683122, 1.000000000000000000, 0.9659258262890683122, 1.000000000000000000, 0.9659258262890683122, 1.000000000000000000, 0.9659258262890683122, 1.000000000000000000, 0.9659258262890683122, 1.000000000000000000, 0.9659258262890683122, 1.000000000000000000, 0.9659258262890683122, 1.000000000000000000, 0.9659258262890683122, 1.000000000000000000, 0.9659258262890683122, 1.000000000000000000, 0.9659258262890683122, 1.000000000000000000, 0.9659258262890683122, 1.000000000000000000, 0.9659258262890683122, 1.000000000000000000, 0.9659258262890683122, 1.000000000000000000, 0.9659258262890683122, 1.000000000000000000, 0.9659258262890683122, 1.000000000000000000, 0.9659258262890683122, 1.000000000000000000, 0.9659258262890683122, 1.000000000000000000, 0.9659258262890683122, 1.000000000000000000, 0.9659258262890683122, 1.000000000000000000, 0.9659258262890683122, 1.000000000000000000, 0.9659258262890683122, 1.000000000000000000, 0.9659258262890683122, 1.000000000000000000, 0.9659258262890683122, 1.000000000000000000, 0.9659258262890683122, 1.000000000000000000, 0.9659258262890683122, 1.000000000000000000, 0.9659258262890683122, 1.000000000000000000, 0.9659258262890683122, 1.000000000000000000, 0.9659258262890683122, 1.000000000000000000, 0.9659258262890683122, 1.000000000000000000, 0.9659258262890683122, 1.000000000000000000, 0.9659258262890683122, 1.000000000000000000, 0.9659258262890683122, 1.000000000000000000, 0.9659258262890683122, 1.000000000000000000, 0.9659258262890683122, 1.000000000000000000, 0.9659258262890683122, 1.000000000000000000, 0.9659258262890683122, 1.000000000000000000, 0.9659258262890683122, 1.000000000000000000, 0.9659258262890683122, 1.000000000000000000, 0.9659258262890683122, 1.000000000000000000, 0.9659258262890683122, 1.000000000000000000, 0.9659258262890683122, 1.000000000000000000, 0.9659258262890683122, 1.000000000000000000, 0.9659258262890683122, 1.000000000000000000, 0.9659258262890683122, 1.000000000000000000, 0.9659258262890683122, 1.000000000000000000, 0.9659258262890683122, 1.000000000000000000, 0.9659258262890683122, 1.000000000000000000, 0.9659258262890683122, 1.000000000000000000, 0.9659258262890683122, 1.000000000000000000, 0.9659258262890683122, 1.000000000000000000, 0.9659258262890683122, 1.000000000000000000, 0.9659258262890683122, 1.000000000000000000, 0.9659258262890683122, 1.000000000000000000, 0.9659258262890683122, 1.000000000000000000, 0.9659258262890683122, 1.000000000000000000, 0.9659258262890683122, 1.000000000000000000, 0.9659258262890683122, 1.000000000000000000, 0.9659258262890683122, 1.000000000000000000, 0.9659258262890683122, 1.000000000000000000, 0.9659258262890683122, 1.000000000000000000, 0.9659258262890683122, 1.000000000000000000, 0.9659258262890683122, 1.000000000000000000, 0.9659258262890683122, 1.000000000000000000, 0.9659258262890683122, 1.000000000000000000, 0.9659258262890683122, 1.000000000000000000, 0.9659258262890683122, 1.000000000000000000, 0.9659258262890683122, 1.000000000000000000, 0.9659258262890683122, 1.000000000000000000, 0.9659258262890683122, 1.000000000000000000, 0.9659258262890683122, 1.000000000000000000, 0.9659258262890683122, 1.000000000000000000, 0.9659258262890683122, 1.000000000000000000, 0.9659258262890683122, 1.000000000000000000, 0.9659258262890683122, 1.000000000000000000, 0.9659258262890683122, 1.000000000000000000, 0.9659258262890683122, 1.000000000000000000, 0.9659258262890683122, 1.000000000000000000, 0.9659258262890683122, 1.000000000000000000, 0.9659258262890683122, 1.000000000000000000, 0.9659258262890683122, 1.000000000000000000, 0.9659258262890683122, 1.000000000000000000, 0.9659258262890683122, 1.000000000000000000, 0.9659258262890683122, 1.000000000000000000, 0.9659258262890683122, 1.000000000000000000, 0.9659258262890683122, 1.000000000000000000, 0.9659258262890683122, 1.000000000000000000, 0.9659258262890683122, 1.000000000000000000, 0.9659258262890683122, 1.000000000000000000, 0.9659258262890683122, 1.000000000000000000, 0.9659258262890683122, 1.000000000000000000, 0.9659258262890683122, 1.000000000000000000, 0.9659258262890683122, 1.000000000000000000, 0.9659258262890683122, 1.000000000000000000, 0.9659258262890683122, 1.000000000000000000, 0.9659258262890683122, 1.000000000000000000, 0.9659258262890683122, 1.000000000000000000, 0.9659258262890683122, 1.000000000000000000, 0.9659258262890683122, 1.000000000000000000, 0.9659258262890683122, 1.000000000000000000, 0.9659258262890683122, 1.000000000000000000, 0.9659258262890683122, 1.000000000000000000, 0.9659258262890683122, 1.000000000000000000, 0.9659258262890683122, 1.000000000000000000, 0.9659258262890683122, 1.000000000000000000, 0.9659258262890683122, 1.000000000000000000, 0.9659258262890683122, 1.000000000000000000, 0.9659258262890683122, 1.000000000000000000, 0.9659258262890683122, 1.000000000000000000, 0.9659258262890683122, 1.000000000000000000, 0.9659258262890683122, 1.000000000000000000, 0.9659258262890683122, 1.000000000000000000, 0.9659258262890683122, 1.000000000000000000, 0.9659258262890683122, 1.000000000000000000, 0.9659258262890683122, 1.000000000000000000, 0.9659258262890683122, 1.000000000000000000, 0.9659258262890683122, 1.000000000000000000, 0.9659258262890683122, 1.000000000000000000, 0.9659258262890683122, 1.000000000000000000, 0.9659258262890683122, 1.000000000000000000, 0.9659258262890683122, 1.000000000000000000, 0.9659258262890683122, 1.000000000000000000, 0.9659258262890683122, 1.000000000000000000, 0.9659258262890683122, 1.000000000000000000, 0.9659258262890683122, 1.000000000000000000, 0.9659258262890683122, 1.000000000000000000, 0.9659258262890683122, 1.000000000000000000, 0.9659258262890683122, 1.000000000000000000, 0.9659258262890683122, 1.000000000000000000, 0.9659258262890683122, 1.000000000000000000, 0.9659258262890683122, 1.000000000000000000, 0.9659258262890683122, 1.000000000000000000, 0.9659258262890683122, 1.000000000000000000, 0.9659258262890683122, 1.000000000000000000, 0.9659258262890683122, 1.000000000000000000, 0.9659258262890683122, 1.000000000000000000, 0.9659258262890683122, 1.000000000000000000, 0.9659258262890683122, 1.000000000000000000, 0.9659258262890683122, 1.000000000000000000, 0.9659258262890683122, 1.000000000000000000, 0.9659258262890683122, 1.000000000000000000, 0.9659258262890683122, 1.000000000000000000, 0.9659258262890683122, 1.000000000000000000, 0.9659258262890683122, 1.000000000000000000, 0.9659258262890683122, 1.000000000000000000, 0.9659258262890683122, 1.000000000000000000, 0.9659258262890683122, 1.000000000000000000, 0.9659258262890683122, 1.000000000000000000, 0.9659258262890683122, 1.000000000000000000, 0.9659258262890683122, 1.000000000000000000, 0.9659258262890683122, 1.000000000000000000, 0.9659258262890683122, 1.000000000000000000, 0.9659258262890683122, 1.000000000000000000, 0.9659258262890683122, 1.000000000000000000, 0.9659258262890683122, 1.000000000000000000, 0.9659258262890683122, 1.000000000000000000, 0.9659258262890683122, 1.000000000000000000, 0.9659258262890683122, 1.000000000000000000, 0.9659258262890683122, 1.000000000000000000, 0.9659258262890683122, 1.000000000000000000, 0.9659258262890683122, 1.000000000000000000, 0.9659258262890683122, 1.000000000000000000, 0.9659258262890683122, 1.000000000000000000, 0.9659258262890683122, 1.000000000000000000, 0.9659258262890683122, 1.000000000000000000, 0.9659258262890683122, 1.000000000000000000, 0.9659258262890683122, 1.000000000000000000, 0.9659258262890683122, 1.000000000000000000, 0.9659258262890683122, 1.000000000000000000, 0.9659258262890683122, 1.000000000000000000, 0.9659258262890683122, 1.000000000000000000, 0.9659258262890683122, 1.000000000000000000, 0.9659258262890683122, 1.000000000000000000, 0.9659258262890683122, 1.000000000000000000, 0.9659258262890683122, 1.000000000000000000, 0.9659258262890683122, 1.000000000000000000, 0.9659258262890683122, 1.000000000000000000, 0.9659258262890683122, 1.000000000000000000, 0.9659258262890683122, 1.000000000000000000, 0.9659258262890683122, 1.000000000000000000, 0.9659258262890683122, 1.000000000000000000, 0.9659258262890683122, 1.000000000000000000, 0.9659258262890683122, 1.000000000000000000, 0.9659258262890683122, 1.000000000000000000, 0.9659258262890683122, 1.000000000000000000, 0.9659258262890683122, 1.000000000000000000, 0.9659258262890683122, 1.000000000000000000, 0.9659258262890683122, 1.000000000000000000),
 ( 0.3333333333333333703, 0.3219752754296894559, 0.3333333333333333703, 0.3219752754296894559, 0.3333333333333333703, 0.3219752754296894559, 0.3333333333333333703, 0.3219752754296894559, 0.3333333333333333703, 0.3219752754296894559, 0.3333333333333333703, 0.3219752754296894559, 0.3333333333333333703, 0.3219752754296894559, 0.3333333333333333703, 0.3219752754296894559, 0.3333333333333333703, 0.3219752754296894559, 0.3333333333333333703, 0.3219752754296894559, 0.3333333333333333703, 0.3219752754296894559, 0.3333333333333333703, 0.3219752754296894559, 0.3333333333333333703, 0.3219752754296894559, 0.3333333333333333703, 0.3219752754296894559, 0.3333333333333333703, 0.3219752754296894559, 0.3333333333333333703, 0.3219752754296894559, 0.3333333333333333703, 0.3219752754296894559, 0.3333333333333333703, 0.3219752754296894559, 0.3333333333333333703, 0.3219752754296894559, 0.3333333333333333703, 0.3219752754296894559, 0.3333333333333333703, 0.3219752754296894559, 0.3333333333333333703, 0.3219752754296894559, 0.3333333333333333703, 0.3219752754296894559, 0.3333333333333333703, 0.3219752754296894559, 0.3333333333333333703, 0.3219752754296894559, 0.3333333333333333703, 0.3219752754296894559, 0.3333333333333333703, 0.3219752754296894559, 0.3333333333333333703, 0.3219752754296894559, 0.3333333333333333703, 0.3219752754296894559, 0.3333333333333333703, 0.3219752754296894559, 0.3333333333333333703, 0.3219752754296894559, 0.3333333333333333703, 0.3219752754296894559, 0.3333333333333333703, 0.3219752754296894559, 0.3333333333333333703, 0.3219752754296894559, 0.3333333333333333703, 0.3219752754296894559, 0.3333333333333333703, 0.3219752754296894559, 0.3333333333333333703, 0.3219752754296894559, 0.3333333333333333703, 0.3219752754296894559, 0.3333333333333333703, 0.3219752754296894559, 0.3333333333333333703, 0.3219752754296894559, 0.3333333333333333703, 0.3219752754296894559, 0.3333333333333333703, 0.3219752754296894559, 0.3333333333333333703, 0.3219752754296894559, 0.3333333333333333703, 0.3219752754296894559, 0.3333333333333333703, 0.3219752754296894559, 0.3333333333333333703, 0.3219752754296894559, 0.3333333333333333703, 0.3219752754296894559, 0.3333333333333333703, 0.3219752754296894559, 0.3333333333333333703, 0.3219752754296894559, 0.3333333333333333703, 0.3219752754296894559, 0.3333333333333333703, 0.3219752754296894559, 0.3333333333333333703, 0.3219752754296894559, 0.3333333333333333703, 0.3219752754296894559, 0.3333333333333333703, 0.3219752754296894559, 0.3333333333333333703, 0.3219752754296894559, 0.3333333333333333703, 0.3219752754296894559, 0.3333333333333333703, 0.3219752754296894559, 0.3333333333333333703, 0.3219752754296894559, 0.3333333333333333703, 0.3219752754296894559, 0.3333333333333333703, 0.3219752754296894559, 0.3333333333333333703, 0.3219752754296894559, 0.3333333333333333703, 0.3219752754296894559, 0.3333333333333333703, 0.3219752754296894559, 0.3333333333333333703, 0.3219752754296894559, 0.3333333333333333703, 0.3219752754296894559, 0.3333333333333333703, 0.3219752754296894559, 0.3333333333333333703, 0.3219752754296894559, 0.3333333333333333703, 0.3219752754296894559, 0.3333333333333333703, 0.3219752754296894559, 0.3333333333333333703, 0.3219752754296894559, 0.3333333333333333703, 0.3219752754296894559, 0.3333333333333333703, 0.3219752754296894559, 0.3333333333333333703, 0.3219752754296894559, 0.3333333333333333703, 0.3219752754296894559, 0.3333333333333333703, 0.3219752754296894559, 0.3333333333333333703, 0.3219752754296894559, 0.3333333333333333703, 0.3219752754296894559, 0.3333333333333333703, 0.3219752754296894559, 0.3333333333333333703, 0.3219752754296894559, 0.3333333333333333703, 0.3219752754296894559, 0.3333333333333333703, 0.3219752754296894559, 0.3333333333333333703, 0.3219752754296894559, 0.3333333333333333703, 0.3219752754296894559, 0.3333333333333333703, 0.3219752754296894559, 0.3333333333333333703, 0.3219752754296894559, 0.3333333333333333703, 0.3219752754296894559, 0.3333333333333333703, 0.3219752754296894559, 0.3333333333333333703, 0.3219752754296894559, 0.3333333333333333703, 0.3219752754296894559, 0.3333333333333333703, 0.3219752754296894559, 0.3333333333333333703, 0.3219752754296894559, 0.3333333333333333703, 0.3219752754296894559, 0.3333333333333333703, 0.3219752754296894559, 0.3333333333333333703, 0.3219752754296894559, 0.3333333333333333703, 0.3219752754296894559, 0.3333333333333333703, 0.3219752754296894559, 0.3333333333333333703, 0.3219752754296894559, 0.3333333333333333703, 0.3219752754296894559, 0.3333333333333333703, 0.3219752754296894559, 0.3333333333333333703, 0.3219752754296894559, 0.3333333333333333703, 0.3219752754296894559, 0.3333333333333333703, 0.3219752754296894559, 0.3333333333333333703, 0.3219752754296894559, 0.3333333333333333703, 0.3219752754296894559, 0.3333333333333333703, 0.3219752754296894559, 0.3333333333333333703, 0.3219752754296894559, 0.3333333333333333703, 0.3219752754296894559, 0.3333333333333333703, 0.3219752754296894559, 0.3333333333333333703, 0.3219752754296894559, 0.3333333333333333703, 0.3219752754296894559, 0.3333333333333333703, 0.3219752754296894559, 0.3333333333333333703, 0.3219752754296894559, 0.3333333333333333703, 0.3219752754296894559, 0.3333333333333333703, 0.3219752754296894559, 0.3333333333333333703, 0.3219752754296894559, 0.3333333333333333703, 0.3219752754296894559, 0.3333333333333333703, 0.3219752754296894559, 0.3333333333333333703, 0.3219752754296894559, 0.3333333333333333703, 0.3219752754296894559, 0.3333333333333333703, 0.3219752754296894559, 0.3333333333333333703, 0.3219752754296894559, 0.3333333333333333703, 0.3219752754296894559, 0.3333333333333333703, 0.3219752754296894559, 0.3333333333333333703, 0.3219752754296894559, 0.3333333333333333703, 0.3219752754296894559, 0.3333333333333333703, 0.3219752754296894559, 0.3333333333333333703, 0.3219752754296894559, 0.3333333333333333703, 0.3219752754296894559, 0.3333333333333333703, 0.3219752754296894559, 0.3333333333333333703, 0.3219752754296894559, 0.3333333333333333703, 0.3219752754296894559, 0.3333333333333333703, 0.3219752754296894559, 0.3333333333333333703, 0.3219752754296894559, 0.3333333333333333703, 0.3219752754296894559, 0.3333333333333333703, 0.3219752754296894559, 0.3333333333333333703, 0.3219752754296894559, 0.3333333333333333703, 0.3219752754296894559, 0.3333333333333333703, 0.3219752754296894559, 0.3333333333333333703, 0.3219752754296894559, 0.3333333333333333703, 0.3219752754296894559, 0.3333333333333333703, 0.3219752754296894559, 0.3333333333333333703, 0.3219752754296894559, 0.3333333333333333703, 0.3219752754296894559, 0.3333333333333333703, 0.3219752754296894559, 0.3333333333333333703, 0.3219752754296894559, 0.3333333333333333703, 0.3219752754296894559, 0.3333333333333333703, 0.3219752754296894559, 0.3333333333333333703, 0.3219752754296894559, 0.3333333333333333703, 0.3219752754296894559, 0.3333333333333333703, 0.3219752754296894559, 0.3333333333333333703, 0.3219752754296894559, 0.3333333333333333703, 0.3219752754296894559, 0.3333333333333333703, 0.3219752754296894559, 0.3333333333333333703, 0.3219752754296894559, 0.3333333333333333703, 0.3219752754296894559, 0.3333333333333333703, 0.3219752754296894559, 0.3333333333333333703, 0.3219752754296894559, 0.3333333333333333703, 0.3219752754296894559, 0.3333333333333333703, 0.3219752754296894559, 0.3333333333333333703, 0.3219752754296894559, 0.3333333333333333703, 0.3219752754296894559, 0.3333333333333333703, 0.3219752754296894559, 0.3333333333333333703, 0.3219752754296894559, 0.3333333333333333703, 0.3219752754296894559, 0.3333333333333333703, 0.3219752754296894559, 0.3333333333333333703, 0.3219752754296894559, 0.3333333333333333703, 0.3219752754296894559, 0.3333333333333333703, 0.3219752754296894559, 0.3333333333333333703, 0.3219752754296894559, 0.3333333333333333703, 0.3219752754296894559, 0.3333333333333333703, 0.3219752754296894559, 0.3333333333333333703, 0.3219752754296894559, 0.3333333333333333703, 0.3219752754296894559, 0.3333333333333333703, 0.3219752754296894559, 0.3333333333333333703, 0.3219752754296894559, 0.3333333333333333703, 0.3219752754296894559, 0.3333333333333333703, 0.3219752754296894559, 0.3333333333333333703, 0.3219752754296894559, 0.3333333333333333703, 0.3219752754296894559, 0.3333333333333333703, 0.3219752754296894559, 0.3333333333333333703, 0.3219752754296894559, 0.3333333333333333703, 0.3219752754296894559, 0.3333333333333333703, 0.3219752754296894559, 0.3333333333333333703, 0.3219752754296894559, 0.3333333333333333703, 0.3219752754296894559, 0.3333333333333333703, 0.3219752754296894559, 0.3333333333333333703, 0.3219752754296894559, 0.3333333333333333703, 0.3219752754296894559, 0.3333333333333333703, 0.3219752754296894559, 0.3333333333333333703, 0.3219752754296894559, 0.3333333333333333703, 0.3219752754296894559, 0.3333333333333333703, 0.3219752754296894559, 0.3333333333333333703),
 ( 0.3333333333333333703, 0.3219752754296894559, 0.3333333333333333703, 0.3219752754296894559, 0.3333333333333333703, 0.3219752754296894559, 0.3333333333333333703, 0.3219752754296894559, 0.3333333333333333703, 0.3219752754296894559, 0.3333333333333333703, 0.3219752754296894559, 0.3333333333333333703, 0.3219752754296894559, 0.3333333333333333703, 0.3219752754296894559, 0.3333333333333333703, 0.3219752754296894559, 0.3333333333333333703, 0.3219752754296894559, 0.3333333333333333703, 0.3219752754296894559, 0.3333333333333333703, 0.3219752754296894559, 0.3333333333333333703, 0.3219752754296894559, 0.3333333333333333703, 0.3219752754296894559, 0.3333333333333333703, 0.3219752754296894559, 0.3333333333333333703, 0.3219752754296894559, 0.3333333333333333703, 0.3219752754296894559, 0.3333333333333333703, 0.3219752754296894559, 0.3333333333333333703, 0.3219752754296894559, 0.3333333333333333703, 0.3219752754296894559, 0.3333333333333333703, 0.3219752754296894559, 0.3333333333333333703, 0.3219752754296894559, 0.3333333333333333703, 0.3219752754296894559, 0.3333333333333333703, 0.3219752754296894559, 0.3333333333333333703, 0.3219752754296894559, 0.3333333333333333703, 0.3219752754296894559, 0.3333333333333333703, 0.3219752754296894559, 0.3333333333333333703, 0.3219752754296894559, 0.3333333333333333703, 0.3219752754296894559, 0.3333333333333333703, 0.3219752754296894559, 0.3333333333333333703, 0.3219752754296894559, 0.3333333333333333703, 0.3219752754296894559, 0.3333333333333333703, 0.3219752754296894559, 0.3333333333333333703, 0.3219752754296894559, 0.3333333333333333703, 0.3219752754296894559, 0.3333333333333333703, 0.3219752754296894559, 0.3333333333333333703, 0.3219752754296894559, 0.3333333333333333703, 0.3219752754296894559, 0.3333333333333333703, 0.3219752754296894559, 0.3333333333333333703, 0.3219752754296894559, 0.3333333333333333703, 0.3219752754296894559, 0.3333333333333333703, 0.3219752754296894559, 0.3333333333333333703, 0.3219752754296894559, 0.3333333333333333703, 0.3219752754296894559, 0.3333333333333333703, 0.3219752754296894559, 0.3333333333333333703, 0.3219752754296894559, 0.3333333333333333703, 0.3219752754296894559, 0.3333333333333333703, 0.3219752754296894559, 0.3333333333333333703, 0.3219752754296894559, 0.3333333333333333703, 0.3219752754296894559, 0.3333333333333333703, 0.3219752754296894559, 0.3333333333333333703, 0.3219752754296894559, 0.3333333333333333703, 0.3219752754296894559, 0.3333333333333333703, 0.3219752754296894559, 0.3333333333333333703, 0.3219752754296894559, 0.3333333333333333703, 0.3219752754296894559, 0.3333333333333333703, 0.3219752754296894559, 0.3333333333333333703, 0.3219752754296894559, 0.3333333333333333703, 0.3219752754296894559, 0.3333333333333333703, 0.3219752754296894559, 0.3333333333333333703, 0.3219752754296894559, 0.3333333333333333703, 0.3219752754296894559, 0.3333333333333333703, 0.3219752754296894559, 0.3333333333333333703, 0.3219752754296894559, 0.3333333333333333703, 0.3219752754296894559, 0.3333333333333333703, 0.3219752754296894559, 0.3333333333333333703, 0.3219752754296894559, 0.3333333333333333703, 0.3219752754296894559, 0.3333333333333333703, 0.3219752754296894559, 0.3333333333333333703, 0.3219752754296894559, 0.3333333333333333703, 0.3219752754296894559, 0.3333333333333333703, 0.3219752754296894559, 0.3333333333333333703, 0.3219752754296894559, 0.3333333333333333703, 0.3219752754296894559, 0.3333333333333333703, 0.3219752754296894559, 0.3333333333333333703, 0.3219752754296894559, 0.3333333333333333703, 0.3219752754296894559, 0.3333333333333333703, 0.3219752754296894559, 0.3333333333333333703, 0.3219752754296894559, 0.3333333333333333703, 0.3219752754296894559, 0.3333333333333333703, 0.3219752754296894559, 0.3333333333333333703, 0.3219752754296894559, 0.3333333333333333703, 0.3219752754296894559, 0.3333333333333333703, 0.3219752754296894559, 0.3333333333333333703, 0.3219752754296894559, 0.3333333333333333703, 0.3219752754296894559, 0.3333333333333333703, 0.3219752754296894559, 0.3333333333333333703, 0.3219752754296894559, 0.3333333333333333703, 0.3219752754296894559, 0.3333333333333333703, 0.3219752754296894559, 0.3333333333333333703, 0.3219752754296894559, 0.3333333333333333703, 0.3219752754296894559, 0.3333333333333333703, 0.3219752754296894559, 0.3333333333333333703, 0.3219752754296894559, 0.3333333333333333703, 0.3219752754296894559, 0.3333333333333333703, 0.3219752754296894559, 0.3333333333333333703, 0.3219752754296894559, 0.3333333333333333703, 0.3219752754296894559, 0.3333333333333333703, 0.3219752754296894559, 0.3333333333333333703, 0.3219752754296894559, 0.3333333333333333703, 0.3219752754296894559, 0.3333333333333333703, 0.3219752754296894559, 0.3333333333333333703, 0.3219752754296894559, 0.3333333333333333703, 0.3219752754296894559, 0.3333333333333333703, 0.3219752754296894559, 0.3333333333333333703, 0.3219752754296894559, 0.3333333333333333703, 0.3219752754296894559, 0.3333333333333333703, 0.3219752754296894559, 0.3333333333333333703, 0.3219752754296894559, 0.3333333333333333703, 0.3219752754296894559, 0.3333333333333333703, 0.3219752754296894559, 0.3333333333333333703, 0.3219752754296894559, 0.3333333333333333703, 0.3219752754296894559, 0.3333333333333333703, 0.3219752754296894559, 0.3333333333333333703, 0.3219752754296894559, 0.3333333333333333703, 0.3219752754296894559, 0.3333333333333333703, 0.3219752754296894559, 0.3333333333333333703, 0.3219752754296894559, 0.3333333333333333703, 0.3219752754296894559, 0.3333333333333333703, 0.3219752754296894559, 0.3333333333333333703, 0.3219752754296894559, 0.3333333333333333703, 0.3219752754296894559, 0.3333333333333333703, 0.3219752754296894559, 0.3333333333333333703, 0.3219752754296894559, 0.3333333333333333703, 0.3219752754296894559, 0.3333333333333333703, 0.3219752754296894559, 0.3333333333333333703, 0.3219752754296894559, 0.3333333333333333703, 0.3219752754296894559, 0.3333333333333333703, 0.3219752754296894559, 0.3333333333333333703, 0.3219752754296894559, 0.3333333333333333703, 0.3219752754296894559, 0.3333333333333333703, 0.3219752754296894559, 0.3333333333333333703, 0.3219752754296894559, 0.3333333333333333703, 0.3219752754296894559, 0.3333333333333333703, 0.3219752754296894559, 0.3333333333333333703, 0.3219752754296894559, 0.3333333333333333703, 0.3219752754296894559, 0.3333333333333333703, 0.3219752754296894559, 0.3333333333333333703, 0.3219752754296894559, 0.3333333333333333703, 0.3219752754296894559, 0.3333333333333333703, 0.3219752754296894559, 0.3333333333333333703, 0.3219752754296894559, 0.3333333333333333703, 0.3219752754296894559, 0.3333333333333333703, 0.3219752754296894559, 0.3333333333333333703, 0.3219752754296894559, 0.3333333333333333703, 0.3219752754296894559, 0.3333333333333333703, 0.3219752754296894559, 0.3333333333333333703, 0.3219752754296894559, 0.3333333333333333703, 0.3219752754296894559, 0.3333333333333333703, 0.3219752754296894559, 0.3333333333333333703, 0.3219752754296894559, 0.3333333333333333703, 0.3219752754296894559, 0.3333333333333333703, 0.3219752754296894559, 0.3333333333333333703, 0.3219752754296894559, 0.3333333333333333703, 0.3219752754296894559, 0.3333333333333333703, 0.3219752754296894559, 0.3333333333333333703, 0.3219752754296894559, 0.3333333333333333703, 0.3219752754296894559, 0.3333333333333333703, 0.3219752754296894559, 0.3333333333333333703, 0.3219752754296894559, 0.3333333333333333703, 0.3219752754296894559, 0.3333333333333333703, 0.3219752754296894559, 0.3333333333333333703, 0.3219752754296894559, 0.3333333333333333703, 0.3219752754296894559, 0.3333333333333333703, 0.3219752754296894559, 0.3333333333333333703, 0.3219752754296894559, 0.3333333333333333703, 0.3219752754296894559, 0.3333333333333333703, 0.3219752754296894559, 0.3333333333333333703, 0.3219752754296894559, 0.3333333333333333703, 0.3219752754296894559, 0.3333333333333333703, 0.3219752754296894559, 0.3333333333333333703, 0.3219752754296894559, 0.3333333333333333703, 0.3219752754296894559, 0.3333333333333333703, 0.3219752754296894559, 0.3333333333333333703, 0.3219752754296894559, 0.3333333333333333703, 0.3219752754296894559, 0.3333333333333333703, 0.3219752754296894559, 0.3333333333333333703, 0.3219752754296894559, 0.3333333333333333703, 0.3219752754296894559, 0.3333333333333333703, 0.3219752754296894559, 0.3333333333333333703, 0.3219752754296894559, 0.3333333333333333703, 0.3219752754296894559, 0.3333333333333333703, 0.3219752754296894559, 0.3333333333333333703, 0.3219752754296894559, 0.3333333333333333703, 0.3219752754296894559, 0.3333333333333333703, 0.3219752754296894559, 0.3333333333333333703, 0.3219752754296894559, 0.3333333333333333703, 0.3219752754296894559, 0.3333333333333333703, 0.3219752754296894559, 0.3333333333333333703, 0.3219752754296894559, 0.3333333333333333703, 0.3219752754296894559, 0.3333333333333333703, 0.3219752754296894559, 0.3333333333333333703),
 ( 1.000000000000000000, 0.9659258262890683122, 1.000000000000000000, 0.9659258262890683122, 1.000000000000000000, 0.9659258262890683122, 1.000000000000000000, 0.9659258262890683122, 1.000000000000000000, 0.9659258262890683122, 1.000000000000000000, 0.9659258262890683122, 1.000000000000000000, 0.9659258262890683122, 1.000000000000000000, 0.9659258262890683122, 1.000000000000000000, 0.9659258262890683122, 1.000000000000000000, 0.9659258262890683122, 1.000000000000000000, 0.9659258262890683122, 1.000000000000000000, 0.9659258262890683122, 1.000000000000000000, 0.9659258262890683122, 1.000000000000000000, 0.9659258262890683122, 1.000000000000000000, 0.9659258262890683122, 1.000000000000000000, 0.9659258262890683122, 1.000000000000000000, 0.9659258262890683122, 1.000000000000000000, 0.9659258262890683122, 1.000000000000000000, 0.9659258262890683122, 1.000000000000000000, 0.9659258262890683122, 1.000000000000000000, 0.9659258262890683122, 1.000000000000000000, 0.9659258262890683122, 1.000000000000000000, 0.9659258262890683122, 1.000000000000000000, 0.9659258262890683122, 1.000000000000000000, 0.9659258262890683122, 1.000000000000000000, 0.9659258262890683122, 1.000000000000000000, 0.9659258262890683122, 1.000000000000000000, 0.9659258262890683122, 1.000000000000000000, 0.9659258262890683122, 1.000000000000000000, 0.9659258262890683122, 1.000000000000000000, 0.9659258262890683122, 1.000000000000000000, 0.9659258262890683122, 1.000000000000000000, 0.9659258262890683122, 1.000000000000000000, 0.9659258262890683122, 1.000000000000000000, 0.9659258262890683122, 1.000000000000000000, 0.9659258262890683122, 1.000000000000000000, 0.9659258262890683122, 1.000000000000000000, 0.9659258262890683122, 1.000000000000000000, 0.9659258262890683122, 1.000000000000000000, 0.9659258262890683122, 1.000000000000000000, 0.9659258262890683122, 1.000000000000000000, 0.9659258262890683122, 1.000000000000000000, 0.9659258262890683122, 1.000000000000000000, 0.9659258262890683122, 1.000000000000000000, 0.9659258262890683122, 1.000000000000000000, 0.9659258262890683122, 1.000000000000000000, 0.9659258262890683122, 1.000000000000000000, 0.9659258262890683122, 1.000000000000000000, 0.9659258262890683122, 1.000000000000000000, 0.9659258262890683122, 1.000000000000000000, 0.9659258262890683122, 1.000000000000000000, 0.9659258262890683122, 1.000000000000000000, 0.9659258262890683122, 1.000000000000000000, 0.9659258262890683122, 1.000000000000000000, 0.9659258262890683122, 1.000000000000000000, 0.9659258262890683122, 1.000000000000000000, 0.9659258262890683122, 1.000000000000000000, 0.9659258262890683122, 1.000000000000000000, 0.9659258262890683122, 1.000000000000000000, 0.9659258262890683122, 1.000000000000000000, 0.9659258262890683122, 1.000000000000000000, 0.9659258262890683122, 1.000000000000000000, 0.9659258262890683122, 1.000000000000000000, 0.9659258262890683122, 1.000000000000000000, 0.9659258262890683122, 1.000000000000000000, 0.9659258262890683122, 1.000000000000000000, 0.9659258262890683122, 1.000000000000000000, 0.9659258262890683122, 1.000000000000000000, 0.9659258262890683122, 1.000000000000000000, 0.9659258262890683122, 1.000000000000000000, 0.9659258262890683122, 1.000000000000000000, 0.9659258262890683122, 1.000000000000000000, 0.9659258262890683122, 1.000000000000000000, 0.9659258262890683122, 1.000000000000000000, 0.9659258262890683122, 1.000000000000000000, 0.9659258262890683122, 1.000000000000000000, 0.9659258262890683122, 1.000000000000000000, 0.9659258262890683122, 1.000000000000000000, 0.9659258262890683122, 1.000000000000000000, 0.9659258262890683122, 1.000000000000000000, 0.9659258262890683122, 1.000000000000000000, 0.9659258262890683122, 1.000000000000000000, 0.9659258262890683122, 1.000000000000000000, 0.9659258262890683122, 1.000000000000000000, 0.9659258262890683122, 1.000000000000000000, 0.9659258262890683122, 1.000000000000000000, 0.9659258262890683122, 1.000000000000000000, 0.9659258262890683122, 1.000000000000000000, 0.9659258262890683122, 1.000000000000000000, 0.9659258262890683122, 1.000000000000000000, 0.9659258262890683122, 1.000000000000000000, 0.9659258262890683122, 1.000000000000000000, 0.9659258262890683122, 1.000000000000000000, 0.9659258262890683122, 1.000000000000000000, 0.9659258262890683122, 1.000000000000000000, 0.9659258262890683122, 1.000000000000000000, 0.9659258262890683122, 1.000000000000000000, 0.9659258262890683122, 1.000000000000000000, 0.9659258262890683122, 1.000000000000000000, 0.9659258262890683122, 1.000000000000000000, 0.9659258262890683122, 1.000000000000000000, 0.9659258262890683122, 1.000000000000000000, 0.9659258262890683122, 1.000000000000000000, 0.9659258262890683122, 1.000000000000000000, 0.9659258262890683122, 1.000000000000000000, 0.9659258262890683122, 1.000000000000000000, 0.9659258262890683122, 1.000000000000000000, 0.9659258262890683122, 1.000000000000000000, 0.9659258262890683122, 1.000000000000000000, 0.9659258262890683122, 1.000000000000000000, 0.9659258262890683122, 1.000000000000000000, 0.9659258262890683122, 1.000000000000000000, 0.9659258262890683122, 1.000000000000000000, 0.9659258262890683122, 1.000000000000000000, 0.9659258262890683122, 1.000000000000000000, 0.9659258262890683122, 1.000000000000000000, 0.9659258262890683122, 1.000000000000000000, 0.9659258262890683122, 1.000000000000000000, 0.9659258262890683122, 1.000000000000000000, 0.9659258262890683122, 1.000000000000000000, 0.9659258262890683122, 1.000000000000000000, 0.9659258262890683122, 1.000000000000000000, 0.9659258262890683122, 1.000000000000000000, 0.9659258262890683122, 1.000000000000000000, 0.9659258262890683122, 1.000000000000000000, 0.9659258262890683122, 1.000000000000000000, 0.9659258262890683122, 1.000000000000000000, 0.9659258262890683122, 1.000000000000000000, 0.9659258262890683122, 1.000000000000000000, 0.9659258262890683122, 1.000000000000000000, 0.9659258262890683122, 1.000000000000000000, 0.9659258262890683122, 1.000000000000000000, 0.9659258262890683122, 1.000000000000000000, 0.9659258262890683122, 1.000000000000000000, 0.9659258262890683122, 1.000000000000000000, 0.9659258262890683122, 1.000000000000000000, 0.9659258262890683122, 1.000000000000000000, 0.9659258262890683122, 1.000000000000000000, 0.9659258262890683122, 1.000000000000000000, 0.9659258262890683122, 1.000000000000000000, 0.9659258262890683122, 1.000000000000000000, 0.9659258262890683122, 1.000000000000000000, 0.9659258262890683122, 1.000000000000000000, 0.9659258262890683122, 1.000000000000000000, 0.9659258262890683122, 1.000000000000000000, 0.9659258262890683122, 1.000000000000000000, 0.9659258262890683122, 1.000000000000000000, 0.9659258262890683122, 1.000000000000000000, 0.9659258262890683122, 1.000000000000000000, 0.9659258262890683122, 1.000000000000000000, 0.9659258262890683122, 1.000000000000000000, 0.9659258262890683122, 1.000000000000000000, 0.9659258262890683122, 1.000000000000000000, 0.9659258262890683122, 1.000000000000000000, 0.9659258262890683122, 1.000000000000000000, 0.9659258262890683122, 1.000000000000000000, 0.9659258262890683122, 1.000000000000000000, 0.9659258262890683122, 1.000000000000000000, 0.9659258262890683122, 1.000000000000000000, 0.9659258262890683122, 1.000000000000000000, 0.9659258262890683122, 1.000000000000000000, 0.9659258262890683122, 1.000000000000000000, 0.9659258262890683122, 1.000000000000000000, 0.9659258262890683122, 1.000000000000000000, 0.9659258262890683122, 1.000000000000000000, 0.9659258262890683122, 1.000000000000000000, 0.9659258262890683122, 1.000000000000000000, 0.9659258262890683122, 1.000000000000000000, 0.9659258262890683122, 1.000000000000000000, 0.9659258262890683122, 1.000000000000000000, 0.9659258262890683122, 1.000000000000000000, 0.9659258262890683122, 1.000000000000000000, 0.9659258262890683122, 1.000000000000000000, 0.9659258262890683122, 1.000000000000000000, 0.9659258262890683122, 1.000000000000000000, 0.9659258262890683122, 1.000000000000000000, 0.9659258262890683122, 1.000000000000000000, 0.9659258262890683122, 1.000000000000000000, 0.9659258262890683122, 1.000000000000000000, 0.9659258262890683122, 1.000000000000000000, 0.9659258262890683122, 1.000000000000000000, 0.9659258262890683122, 1.000000000000000000, 0.9659258262890683122, 1.000000000000000000, 0.9659258262890683122, 1.000000000000000000, 0.9659258262890683122, 1.000000000000000000, 0.9659258262890683122, 1.000000000000000000, 0.9659258262890683122, 1.000000000000000000, 0.9659258262890683122, 1.000000000000000000, 0.9659258262890683122, 1.000000000000000000, 0.9659258262890683122, 1.000000000000000000, 0.9659258262890683122, 1.000000000000000000, 0.9659258262890683122, 1.000000000000000000) ) ) 
 REPRESENTATION_ITEM ( '' )  SURFACE ( )  );
#22914=CARTESIAN_POINT ( 'NONE',  ( -7.468012846824272799, 54.10378499907602645, 28.02196122052058413 ) ) ;
#22921=CARTESIAN_POINT ( 'NONE',  ( -24.20753774853730889, 25.03385416666666785, 13.97622843553633842 ) ) ;
#22933=CARTESIAN_POINT ( 'NONE',  ( -7.025853678916861966, 38.34857666574267654, -26.06988505166722803 ) ) ;
#22937=CARTESIAN_POINT ( 'NONE',  ( -13.97622843553632421, 60.26822916666665009, -24.20753774853731599 ) ) ;
#22942=CARTESIAN_POINT ( 'NONE',  ( -15.01150461594642138, 36.20572916666666430, -26.00068869287340334 ) ) ;
#22943=CARTESIAN_POINT ( 'NONE',  ( 25.98046417659858420, 28.76340250092398065, 15.04653450569292872 ) ) ;
#22953=CARTESIAN_POINT ( 'NONE',  ( -20.47846945139902175, 65.00038166759063074, -20.53372385742072481 ) ) ;
#22956=CARTESIAN_POINT ( 'NONE',  ( 20.50609665440969565, 26.60937499999999645, -20.50609665441004736 ) ) ;
#22961=CARTESIAN_POINT ( 'NONE',  ( -7.025853678916861966, 48.66107666574268364, -26.06988505166722803 ) ) ;
#22974=CARTESIAN_POINT ( 'NONE',  ( 26.02091320914876960, 67.13763916574266943, 14.97647472619900455 ) ) ;
#22979=CARTESIAN_POINT ( 'NONE',  ( -24.20753774853756823, 32.48177083333332860, -13.97622843553588723 ) ) ;
#22982=CARTESIAN_POINT ( 'NONE',  ( 28.01184896238290278, 37.20833333333332860, -7.505752307973347470 ) ) ;
#22985=CARTESIAN_POINT ( 'NONE',  ( 7.543491769121427382, 58.69829833425730925, -28.00173670424548433 ) ) ;
#22986=CARTESIAN_POINT ( 'NONE',  ( 27.95245687107223986, 62.85194416759064495, 0.04044903254993640479 ) ) ;
#22989=CARTESIAN_POINT ( 'NONE',  ( -25.98046417659831420, 20.15847249907602290, 15.04653450569339945 ) ) ;
#23012=CARTESIAN_POINT ( 'NONE',  ( -13.94119854578936923, 23.89361083425731280, -24.22776226481241224 ) ) ;
#23017=CARTESIAN_POINT ( 'NONE',  ( 0.04044903254992426173, 44.80506916759064495, -30.02300923189239867 ) ) ;
#23019=CARTESIAN_POINT ( 'NONE',  ( 28.02196122052058413, 39.49440999907601224, 7.468012846824272799 ) ) ;
#23023=CARTESIAN_POINT ( 'NONE',  ( -19.06425588902558133, 61.26524333240935505, 19.11951029504797006 ) ) ;
#23032=CARTESIAN_POINT ( 'NONE',  ( 20.50609665441005092, 41.21875000000000000, 20.50609665440969209 ) ) ;
#23040=CARTESIAN_POINT ( 'NONE',  ( -7.505752307972844761, 14.29166666666666430, 28.01184896238304134 ) ) ;
#23045=CARTESIAN_POINT ( 'NONE',  ( -27.95245687107223986, 27.31993083240935505, 0.04044903255043252877 ) ) ;
#23052=CARTESIAN_POINT ( 'NONE',  ( -26.07999730980477437, 52.67708333333333570, 6.988114217768305103 ) ) ;
#23056=CARTESIAN_POINT ( 'NONE',  ( -19.09188309203694445, 32.62500000000000000, -19.09188309203661049 ) ) ;
#23057=CARTESIAN_POINT ( 'NONE',  ( -15.04653450569291984, 19.31027750092397710, 25.98046417659859486 ) ) ;
#23058=CARTESIAN_POINT ( 'NONE',  ( 20.50609665441005092, 65.28125000000000000, 20.50609665440969209 ) ) ;
#23065=CARTESIAN_POINT ( 'NONE',  ( -27.95245687107223276, 66.57031250000000000, 2.498001805406602216E-13 ) ) ;
#23069=CARTESIAN_POINT ( 'NONE',  ( 19.11951029504763611, 45.23475666759063785, -19.06425588902591173 ) ) ;
#23073=CARTESIAN_POINT ( 'NONE',  ( 2.740863092043355209E-13, 14.14843749999999289, 30.02300923189239512 ) ) ;
#23077=CARTESIAN_POINT ( 'NONE',  ( -20.50609665440969209, 42.07812499999999289, 20.50609665441005092 ) ) ;
#23082=CARTESIAN_POINT ( 'NONE',  ( -20.47846945139866648, 54.39024333240934794, 20.53372385742108008 ) ) ;
#23087=CARTESIAN_POINT ( 'NONE',  ( 26.07999730980477437, 23.45833333333333215, -6.988114217768290004 ) ) ;
#23105=CARTESIAN_POINT ( 'NONE',  ( 6.950374756619721595, 12.00559000092397532, 26.09010956794232428 ) ) ;
#23109=CARTESIAN_POINT ( 'NONE',  ( -7.505752307972844761, 31.47916666666666075, 28.01184896238304134 ) ) ;
#23120=CARTESIAN_POINT ( 'NONE',  ( -20.50609665441004736, 15.43749999999999645, -20.50609665440969565 ) ) ;
#23123=CARTESIAN_POINT ( 'NONE',  ( -2.584737979205442066E-13, 39.92968750000000000, -30.02300923189239867 ) ) ;
#23128=CARTESIAN_POINT ( 'NONE',  ( -14.01125832528328985, 51.95534749907602645, -24.18731323226223040 ) ) ;
#23133=CARTESIAN_POINT ( 'NONE',  ( 19.09188309203694800, 13.71874999999999467, 19.09188309203660694 ) ) ;
#23141=CARTESIAN_POINT ( 'NONE',  ( -6.950374756619247307, 19.72878499907601935, 26.09010956794245217 ) ) ;
#23147=CARTESIAN_POINT ( 'NONE',  ( 6.988114217768294445, 34.63020833333332860, 26.07999730980477437 ) ) ;
#23150=CARTESIAN_POINT ( 'NONE',  ( 2.740863092043355209E-13, 48.52343750000000000, 30.02300923189239512 ) ) ;
#23153=CARTESIAN_POINT ( 'NONE',  ( -28.02196122052045268, 60.98996500092398065, 7.468012846824790607 ) ) ;
#23154=CARTESIAN_POINT ( 'NONE',  ( 26.09010956794232428, 59.27121500092397355, -6.950374756619718042 ) ) ;
#23159=CARTESIAN_POINT ( 'NONE',  ( -7.543491769121917656, 14.28607666574268720, -28.00173670424536354 ) ) ;
#23165=CARTESIAN_POINT ( 'NONE',  ( -15.01150461594642138, 63.70572916666667140, -26.00068869287340334 ) ) ;
#23181=CARTESIAN_POINT ( 'NONE',  ( 19.06425588902592239, 25.46913166759064140, 19.11951029504763611 ) ) ;
#23188=CARTESIAN_POINT ( 'NONE',  ( -0.04044903255044120238, 41.92930583240936215, -30.02300923189239867 ) ) ;
#23192=CARTESIAN_POINT ( 'NONE',  ( -26.06988505166722803, 68.42670166574269786, 7.025853678916877953 ) ) ;
#23195=CARTESIAN_POINT ( 'NONE',  ( -26.00068869287340334, 14.72135416666666607, 15.01150461594643382 ) ) ;
#23202=CARTESIAN_POINT ( 'NONE',  ( -26.00068869287368756, 39.35677083333331439, -15.01150461594595775 ) ) ;
#23203=CARTESIAN_POINT ( 'NONE',  ( 7.505752307972854531, 60.69791666666667140, -28.01184896238303423 ) ) ;
#23215=CARTESIAN_POINT ( 'NONE',  ( 15.01150461594596486, 12.71614583333333037, -26.00068869287367690 ) ) ;
#23221=CARTESIAN_POINT ( 'NONE',  ( -19.11951029504797006, 31.18711833240935150, -19.06425588902558133 ) ) ;
#23229=CARTESIAN_POINT ( 'NONE',  ( 26.07999730980490227, 54.68229166666665719, 6.988114217767821046 ) ) ;
#23233=CARTESIAN_POINT ( 'NONE',  ( -24.20753774853756823, 32.48177083333332860, -13.97622843553588723 ) ) ;
#23235=CARTESIAN_POINT ( 'NONE',  ( 28.00173670424549499, 18.30767333425730214, 7.543491769121417612 ) ) ;
#23236=CARTESIAN_POINT ( 'NONE',  ( -26.00068869287368756, 66.85677083333334281, -15.01150461594595775 ) ) ;
#23247=CARTESIAN_POINT ( 'NONE',  ( 24.18731323226247554, 42.51340250092398065, 14.01125832528285997 ) ) ;
#23251=CARTESIAN_POINT ( 'NONE',  ( -26.00068869287340334, 14.72135416666666607, 15.01150461594643382 ) ) ;
#23255=CARTESIAN_POINT ( 'NONE',  ( -30.02300923189239512, 39.07031249999997868, 2.654126918244515359E-13 ) ) ;
#23260=CARTESIAN_POINT ( 'NONE',  ( 7.543491769121922985, 50.37982666574269075, 28.00173670424535644 ) ) ;
#23268=CARTESIAN_POINT ( 'NONE',  ( 27.95245687107222921, 20.16406249999999645, -2.463307335887066074E-13 ) ) ;
#23283=CARTESIAN_POINT ( 'NONE',  ( -6.950374756619716266, 10.28684000092397532, -26.09010956794232428 ) ) ;
#23288=CARTESIAN_POINT ( 'NONE',  ( -30.02300923189239512, 39.07031249999997868, 2.654126918244515359E-13 ) ) ;
#23300=CARTESIAN_POINT ( 'NONE',  ( -7.505752307973343918, 12.28645833333333037, -28.01184896238290989 ) ) ;
#23302=CARTESIAN_POINT ( 'NONE',  ( 7.505752307973351023, 41.50520833333333570, 28.01184896238290278 ) ) ;
#23310=CARTESIAN_POINT ( 'NONE',  ( -27.95245687107223986, 51.38243083240936215, 0.04044903255043252877 ) ) ;
#23323=CARTESIAN_POINT ( 'NONE',  ( 7.025853678916867295, 19.44232666574268364, 26.06988505166722803 ) ) ;
#23326=PRODUCT ( 'Linear Compliance Spring & Shaft', 'Linear Compliance Spring & Shaft', '', ( #5103 ) ) ;
#23328=CARTESIAN_POINT ( 'NONE',  ( 19.09188309203661049, 43.79687500000000000, -19.09188309203694445 ) ) ;
#23331=CARTESIAN_POINT ( 'NONE',  ( 20.50609665440969565, 47.23437499999999289, -20.50609665441004736 ) ) ;
#23334=CARTESIAN_POINT ( 'NONE',  ( -28.02196122052045268, 64.42746500092397355, 7.468012846824790607 ) ) ;
#23335=CARTESIAN_POINT ( 'NONE',  ( 15.04653450569292872, 17.59152750092397355, -25.98046417659857710 ) ) ;
#23338=CARTESIAN_POINT ( 'NONE',  ( 28.02196122052058413, 15.43190999907601935, 7.468012846824272799 ) ) ;
#23344=CARTESIAN_POINT ( 'NONE',  ( 30.02300923189239512, 64.85156249999998579, -2.619432448724977703E-13 ) ) ;
#23357=CARTESIAN_POINT ( 'NONE',  ( 6.950374756619721595, 29.19309000092397000, 26.09010956794232428 ) ) ;
#23363=CARTESIAN_POINT ( 'NONE',  ( -20.47846945139866648, 47.51524333240936215, 20.53372385742108008 ) ) ;
#23367=CARTESIAN_POINT ( 'NONE',  ( -13.97622843553632421, 19.01822916666666785, -24.20753774853731599 ) ) ;
#23370=CARTESIAN_POINT ( 'NONE',  ( 7.505752307973351023, 24.31770833333332504, 28.01184896238290278 ) ) ;
#23376=CARTESIAN_POINT ( 'NONE',  ( -28.01184896238290278, 38.92708333333333570, 7.505752307973363457 ) ) ;
#23377=CARTESIAN_POINT ( 'NONE',  ( 28.01184896238290278, 57.83333333333333570, -7.505752307973347470 ) ) ;
#23392=CARTESIAN_POINT ( 'NONE',  ( 7.025853678916867295, 33.19232666574268364, 26.06988505166722803 ) ) ;
#23401=CARTESIAN_POINT ( 'NONE',  ( 13.97622843553633665, 58.54947916666665009, 24.20753774853730889 ) ) ;
#23405=CARTESIAN_POINT ( 'NONE',  ( 24.20753774853756113, 44.51302083333332860, 13.97622843553589789 ) ) ;
#23406=CARTESIAN_POINT ( 'NONE',  ( -7.543491769121417612, 22.60454833425730925, 28.00173670424549499 ) ) ;
#23407=CARTESIAN_POINT ( 'NONE',  ( -14.97647472619899389, 19.87201416574269075, 26.02091320914878025 ) ) ;
#23415=CARTESIAN_POINT ( 'NONE',  ( 7.025853678916403666, 38.07329833425730925, -26.06988505166735237 ) ) ;
#23420=CARTESIAN_POINT ( 'NONE',  ( -2.584737979205441561E-13, 19.30468749999999645, -30.02300923189239512 ) ) ;
#23425=CARTESIAN_POINT ( 'NONE',  ( -7.505752307972844761, 52.10416666666666430, 28.01184896238304134 ) ) ;
#23431=CARTESIAN_POINT ( 'NONE',  ( -28.02196122052058413, 58.40065999907601935, -7.468012846824272799 ) ) ;
#23433=CARTESIAN_POINT ( 'NONE',  ( -7.505752307973343918, 63.84895833333332860, -28.01184896238290989 ) ) ;
#23436=CARTESIAN_POINT ( 'NONE',  ( 6.988114217767829928, 64.13541666666667140, -26.07999730980489872 ) ) ;
#23439=CARTESIAN_POINT ( 'NONE',  ( 26.07999730980477437, 20.02083333333332860, -6.988114217768290004 ) ) ;
#23445=CARTESIAN_POINT ( 'NONE',  ( -26.09010956794232428, 50.67746500092398065, 6.950374756619732253 ) ) ;
#23456=CARTESIAN_POINT ( 'NONE',  ( 27.95245687107223986, 18.16444416759064140, 0.04044903254993640479 ) ) ;
#23460=CARTESIAN_POINT ( 'NONE',  ( 20.50609665441005092, 44.65624999999999289, 20.50609665440969209 ) ) ;
#23470=CARTESIAN_POINT ( 'NONE',  ( -14.97647472619899389, 30.18451416574268720, 26.02091320914878025 ) ) ;
#23472=CARTESIAN_POINT ( 'NONE',  ( 20.50609665441005092, 41.21875000000000000, 20.50609665440969209 ) ) ;
#23479=CARTESIAN_POINT ( 'NONE',  ( 19.06425588902558133, 49.23399333240936215, -19.11951029504797006 ) ) ;
#23484=CARTESIAN_POINT ( 'NONE',  ( 24.20753774853756113, 13.57552083333333037, 13.97622843553589789 ) ) ;
#23493=CARTESIAN_POINT ( 'NONE',  ( 14.01125832528330051, 19.29909749907602290, 24.18731323226221974 ) ) ;
#23498=CARTESIAN_POINT ( 'NONE',  ( 2.584737979205441561E-13, 41.64843750000000000, 27.95245687107222921 ) ) ;
#23502=CARTESIAN_POINT ( 'NONE',  ( 20.50609665441005092, 48.09375000000000000, 20.50609665440969209 ) ) ;
#23504=CARTESIAN_POINT ( 'NONE',  ( -28.00173670424549499, 64.71392333425730214, -7.543491769121417612 ) ) ;
#23505=CARTESIAN_POINT ( 'NONE',  ( -7.468012846824771955, 13.72434000092397532, -28.02196122052045624 ) ) ;
#23524=CARTESIAN_POINT ( 'NONE',  ( -13.94119854578936923, 34.20611083425730925, -24.22776226481241224 ) ) ;
#23531=CARTESIAN_POINT ( 'NONE',  ( 25.98046417659831775, 45.93972249907602645, -15.04653450569338879 ) ) ;
#23536=CARTESIAN_POINT ( 'NONE',  ( -2.428612866367529427E-13, 12.42968749999999289, -27.95245687107222921 ) ) ;
#23540=CARTESIAN_POINT ( 'NONE',  ( -7.505752307973343918, 26.03645833333333215, -28.01184896238290989 ) ) ;
#23544=CARTESIAN_POINT ( 'NONE',  ( 20.53372385742072481, 41.79725666759063785, -20.47846945139902175 ) ) ;
#23546=CARTESIAN_POINT ( 'NONE',  ( -2.584737979205441561E-13, 46.80468750000000000, -30.02300923189239512 ) ) ;
#23556=CARTESIAN_POINT ( 'NONE',  ( -26.00068869287368756, 22.16927083333332860, -15.01150461594595775 ) ) ;
#23561=CARTESIAN_POINT ( 'NONE',  ( 19.06425588902558133, 32.04649333240934084, -19.11951029504797006 ) ) ;
#23568=CARTESIAN_POINT ( 'NONE',  ( -6.988114217767819270, 55.54166666666667140, 26.07999730980490583 ) ) ;
#23572=CARTESIAN_POINT ( 'NONE',  ( -24.20753774853730889, 38.78385416666665719, 13.97622843553634020 ) ) ;
#23573=CARTESIAN_POINT ( 'NONE',  ( 14.97647472619947351, 32.48736083425731636, 26.02091320914850314 ) ) ;
#23574=CARTESIAN_POINT ( 'NONE',  ( 28.02196122052058413, 15.43190999907601935, 7.468012846824272799 ) ) ;
#23578=CARTESIAN_POINT ( 'NONE',  ( 24.18731323226221974, 45.93972249907602645, -14.01125832528328985 ) ) ;
#23585=CARTESIAN_POINT ( 'NONE',  ( -24.18731323226248264, 40.79465250092398065, -14.01125832528284931 ) ) ;
#23589=CARTESIAN_POINT ( 'NONE',  ( -28.01184896238290278, 18.30208333333332860, 7.505752307973363457 ) ) ;
#23593=CARTESIAN_POINT ( 'NONE',  ( 26.00068869287367335, 44.51302083333331439, 15.01150461594596308 ) ) ;
#23598=CARTESIAN_POINT ( 'NONE',  ( 7.468012846824281681, 62.69753499907601224, -28.02196122052058058 ) ) ;
#23600=CARTESIAN_POINT ( 'NONE',  ( -15.01150461594595775, 65.99739583333332860, 26.00068869287368756 ) ) ;
#23602=CARTESIAN_POINT ( 'NONE',  ( 26.07999730980490227, 64.99479166666665719, 6.988114217767821046 ) ) ;
#23605=CARTESIAN_POINT ( 'NONE',  ( -13.97622843553632421, 29.33072916666665719, -24.20753774853731599 ) ) ;
#23611=CARTESIAN_POINT ( 'NONE',  ( 13.94119854578937812, 53.11236083425731636, 24.22776226481240514 ) ) ;
#23623=CARTESIAN_POINT ( 'NONE',  ( 19.06425588902592239, 15.15663166759064495, 19.11951029504763611 ) ) ;
#23628=CARTESIAN_POINT ( 'NONE',  ( 7.505752307972854531, 40.07291666666666430, -28.01184896238303423 ) ) ;
#23632=CARTESIAN_POINT ( 'NONE',  ( 28.01184896238290278, 23.45833333333333215, -7.505752307973347470 ) ) ;
#23640=CARTESIAN_POINT ( 'NONE',  ( -28.00173670424535644, 34.05170166574267654, 7.543491769121936308 ) ) ;
#23642=CARTESIAN_POINT ( 'NONE',  ( -7.505752307973343918, 39.78645833333332860, -28.01184896238290989 ) ) ;
#23649=CARTESIAN_POINT ( 'NONE',  ( 24.22776226481265383, 63.70013916574268364, 13.94119854578893580 ) ) ;
#23662=CARTESIAN_POINT ( 'NONE',  ( 19.06425588902558133, 18.29649333240935150, -19.11951029504797006 ) ) ;
#23667=CARTESIAN_POINT ( 'NONE',  ( 2.584737979205441561E-13, 45.08593750000000711, 27.95245687107222921 ) ) ;
#23671=CARTESIAN_POINT ( 'NONE',  ( -20.50609665441004736, 18.87499999999999645, -20.50609665440969565 ) ) ;
#23672=CARTESIAN_POINT ( 'NONE',  ( -15.04653450569291984, 15.87277750092397710, 25.98046417659859486 ) ) ;
#23678=CARTESIAN_POINT ( 'NONE',  ( 28.01184896238304134, 64.99479166666665719, 7.505752307972846538 ) ) ;
#23691=CARTESIAN_POINT ( 'NONE',  ( -6.950374756619716266, 30.91184000092396644, -26.09010956794232428 ) ) ;
#23698=CARTESIAN_POINT ( 'NONE',  ( 26.02091320914876960, 43.07513916574269786, 14.97647472619900455 ) ) ;
#23702=CARTESIAN_POINT ( 'NONE',  ( -19.09188309203694445, 15.43749999999999645, -19.09188309203661049 ) ) ;
#23705=CARTESIAN_POINT ( 'NONE',  ( -20.50609665440969209, 18.01562499999999645, 20.50609665441005092 ) ) ;
#23709=CARTESIAN_POINT ( 'NONE',  ( 25.98046417659858420, 39.07590250092398065, 15.04653450569292872 ) ) ;
#23711=CARTESIAN_POINT ( 'NONE',  ( -28.01184896238290278, 49.23958333333332860, 7.505752307973363457 ) ) ;
#23722=CARTESIAN_POINT ( 'NONE',  ( -15.01150461594642316, 19.01822916666666430, -26.00068869287341045 ) ) ;
#23728=CARTESIAN_POINT ( 'NONE',  ( 19.11951029504797006, 36.34336833240934794, 19.06425588902558133 ) ) ;
#23737=CARTESIAN_POINT ( 'NONE',  ( 26.07999730980490227, 58.11979166666665719, 6.988114217767821046 ) ) ;
#23741=CARTESIAN_POINT ( 'NONE',  ( 26.07999730980477437, 37.20833333333332860, -6.988114217768290004 ) ) ;
#23742=CARTESIAN_POINT ( 'NONE',  ( -25.98046417659859486, 33.91965250092398065, -15.04653450569291628 ) ) ;
#23743=CARTESIAN_POINT ( 'NONE',  ( 25.98046417659831775, 15.00222249907602112, -15.04653450569338879 ) ) ;
#23747=CARTESIAN_POINT ( 'NONE',  ( -13.94119854578892514, 50.80951416574269075, 24.22776226481266448 ) ) ;
#23753=CARTESIAN_POINT ( 'NONE',  ( -26.06988505166735237, 44.08892333425729504, -7.025853678916388567 ) ) ;
#23758=CARTESIAN_POINT ( 'NONE',  ( -2.584737979205441561E-13, 22.74218749999999645, -30.02300923189239512 ) ) ;
#23762=CARTESIAN_POINT ( 'NONE',  ( 15.01150461594643204, 44.79947916666667140, 26.00068869287340334 ) ) ;
#23768=CARTESIAN_POINT ( 'NONE',  ( -14.97647472619899389, 61.12201416574268364, 26.02091320914878025 ) ) ;
#23773=CARTESIAN_POINT ( 'NONE',  ( -27.95245687107223276, 56.25781249999999289, 2.498001805406602216E-13 ) ) ;
#23778=CARTESIAN_POINT ( 'NONE',  ( 6.988114217768294445, 27.75520833333332860, 26.07999730980477437 ) ) ;
#23784=CARTESIAN_POINT ( 'NONE',  ( -24.22776226481240514, 60.84673583425731636, 13.94119854578937812 ) ) ;
#23796=CARTESIAN_POINT ( 'NONE',  ( 24.18731323226247554, 11.57590250092397355, 14.01125832528285997 ) ) ;
#23801=CARTESIAN_POINT ( 'NONE',  ( 15.01150461594596308, 47.09114583333332860, -26.00068869287367335 ) ) ;
#23806=CARTESIAN_POINT ( 'NONE',  ( -7.505752307972844761, 24.60416666666666430, 28.01184896238304134 ) ) ;
#23812=CARTESIAN_POINT ( 'NONE',  ( 28.00173670424535644, 32.33295166574267654, -7.543491769121920321 ) ) ;
#23814=CARTESIAN_POINT ( 'NONE',  ( -26.00068869287368756, 53.10677083333332149, -15.01150461594595775 ) ) ;
#23819=CARTESIAN_POINT ( 'NONE',  ( -14.01125832528328985, 58.83034749907602645, -24.18731323226223040 ) ) ;
#23826=CARTESIAN_POINT ( 'NONE',  ( -26.07999730980490583, 25.46354166666666430, -6.988114217767815717 ) ) ;
#23834=CARTESIAN_POINT ( 'NONE',  ( -14.01125832528328985, 17.58034749907602290, -24.18731323226223040 ) ) ;
#23838=CARTESIAN_POINT ( 'NONE',  ( 24.20753774853756113, 47.95052083333331439, 13.97622843553589789 ) ) ;
#23842=CARTESIAN_POINT ( 'NONE',  ( -28.01184896238290278, 14.86458333333333037, 7.505752307973363457 ) ) ;
#23843=CARTESIAN_POINT ( 'NONE',  ( -28.02196122052045268, 12.86496500092397710, 7.468012846824790607 ) ) ;
#23864=CARTESIAN_POINT ( 'NONE',  ( 19.11951029504763611, 31.48475666759063074, -19.06425588902591173 ) ) ;
#23871=CARTESIAN_POINT ( 'NONE',  ( 14.97647472619900455, 42.21576416574269075, -26.02091320914876960 ) ) ;
#23874=CARTESIAN_POINT ( 'NONE',  ( 24.20753774853731244, 13.00260416666666430, -13.97622843553632599 ) ) ;
#23876=CARTESIAN_POINT ( 'NONE',  ( 20.50609665441005092, 20.59374999999999645, 20.50609665440969209 ) ) ;
#23880=CARTESIAN_POINT ( 'NONE',  ( 7.468012846824777284, 39.50559000092398065, 28.02196122052045268 ) ) ;
#23882=CARTESIAN_POINT ( 'NONE',  ( -30.02300923189239512, 52.82031249999997868, 2.654126918244515359E-13 ) ) ;
#23883=CARTESIAN_POINT ( 'NONE',  ( -15.01150461594595775, 65.99739583333334281, 26.00068869287368756 ) ) ;
#23892=CARTESIAN_POINT ( 'NONE',  ( -20.50609665441004736, 18.87499999999999645, -20.50609665440969565 ) ) ;
#23897=CARTESIAN_POINT ( 'NONE',  ( -6.950374756619247307, 33.47878499907601935, 26.09010956794245217 ) ) ;
#23904=CARTESIAN_POINT ( 'NONE',  ( -19.09188309203660694, 62.70312500000000000, 19.09188309203694800 ) ) ;
#23909=CARTESIAN_POINT ( 'NONE',  ( -6.988114217768288228, 39.78645833333332860, -26.07999730980477437 ) ) ;
#23910=CARTESIAN_POINT ( 'NONE',  ( -25.98046417659859486, 27.04465250092397000, -15.04653450569291628 ) ) ;
#23911=CARTESIAN_POINT ( 'NONE',  ( 7.543491769121922985, 22.87982666574268720, 28.00173670424535644 ) ) ;
#23915=CARTESIAN_POINT ( 'NONE',  ( -19.06425588902558133, 47.51524333240936215, 19.11951029504797006 ) ) ;
#23923=CARTESIAN_POINT ( 'NONE',  ( 0.04044903254993986036, 51.68006916759063785, -27.95245687107223986 ) ) ;
#23928=CARTESIAN_POINT ( 'NONE',  ( 7.505752307973351023, 27.75520833333332860, 28.01184896238290278 ) ) ;
#23932=CARTESIAN_POINT ( 'NONE',  ( 28.01184896238290278, 47.52083333333332860, -7.505752307973347470 ) ) ;
#23938=CARTESIAN_POINT ( 'NONE',  ( -28.02196122052058413, 65.27565999907601224, -7.468012846824272799 ) ) ;
#23943=CARTESIAN_POINT ( 'NONE',  ( 6.988114217768294445, 62.13020833333334281, 26.07999730980477437 ) ) ;
#23946=CARTESIAN_POINT ( 'NONE',  ( -13.97622843553588901, 28.18489583333332860, 24.20753774853756823 ) ) ;
#23951=CARTESIAN_POINT ( 'NONE',  ( -0.04044903254992426173, 56.83631916759064495, 27.95245687107223276 ) ) ;
#23964=CARTESIAN_POINT ( 'NONE',  ( -19.06425588902591173, 20.31288166759063785, -19.11951029504763611 ) ) ;
#23969=CARTESIAN_POINT ( 'NONE',  ( -30.02300923189239512, 45.94531249999997868, 2.654126918244515359E-13 ) ) ;
#23972=CARTESIAN_POINT ( 'NONE',  ( -28.01184896238304134, 18.58854166666666430, -7.505752307972844761 ) ) ;
#23978=CARTESIAN_POINT ( 'NONE',  ( 20.53372385742108008, 36.34336833240934794, 20.47846945139866648 ) ) ;
#23980=CARTESIAN_POINT ( 'NONE',  ( 20.50609665441005092, 48.09375000000000000, 20.50609665440969209 ) ) ;
#23985=CARTESIAN_POINT ( 'NONE',  ( 24.18731323226221974, 63.12722249907601224, -14.01125832528328985 ) ) ;
#23992=CARTESIAN_POINT ( 'NONE',  ( 6.988114217767829928, 22.88541666666666430, -26.07999730980489872 ) ) ;
#23999=CARTESIAN_POINT ( 'NONE',  ( 0.04044903255044120238, 26.46055583240935505, 27.95245687107223276 ) ) ;
#24002=CARTESIAN_POINT ( 'NONE',  ( -6.988114217767819270, 48.66666666666666430, 26.07999730980490583 ) ) ;
#24006=CARTESIAN_POINT ( 'NONE',  ( 20.50609665440969565, 16.29687499999999645, -20.50609665441004736 ) ) ;
#24007=CARTESIAN_POINT ( 'NONE',  ( -7.543491769121417612, 19.16704833425730570, 28.00173670424549499 ) ) ;
#24019=( NAMED_UNIT ( * ) SI_UNIT ( $, .STERADIAN. ) SOLID_ANGLE_UNIT ( ) );
#24031=CARTESIAN_POINT ( 'NONE',  ( -26.06988505166735237, 33.77642333425730214, -7.025853678916388567 ) ) ;
#24039=CARTESIAN_POINT ( 'NONE',  ( 26.02091320914876960, 46.51263916574269786, 14.97647472619900455 ) ) ;
#24042=SURFACE_STYLE_USAGE ( .BOTH. , #10487 ) ;
#24043=CARTESIAN_POINT ( 'NONE',  ( -26.07999730980477437, 18.30208333333332860, 6.988114217768305103 ) ) ;
#24045=CARTESIAN_POINT ( 'NONE',  ( 2.740863092043355209E-13, 17.58593749999999645, 30.02300923189239512 ) ) ;
#24048=CARTESIAN_POINT ( 'NONE',  ( -25.98046417659859486, 37.35715250092397355, -15.04653450569291628 ) ) ;
#24051=CARTESIAN_POINT ( 'NONE',  ( 30.02300923189239512, 51.10156249999998579, -2.619432448724977703E-13 ) ) ;
#24063=CARTESIAN_POINT ( 'NONE',  ( 7.505752307973351023, 17.44270833333333215, 28.01184896238290278 ) ) ;
#24075=CARTESIAN_POINT ( 'NONE',  ( -24.20753774853730889, 55.97135416666665719, 13.97622843553633842 ) ) ;
#24079=CARTESIAN_POINT ( 'NONE',  ( 27.95245687107223276, 37.35156249999999289, -2.463307335887066074E-13 ) ) ;
#24080=CARTESIAN_POINT ( 'NONE',  ( -15.04653450569291984, 29.62277750092397355, 25.98046417659859486 ) ) ;
#24081=CARTESIAN_POINT ( 'NONE',  ( 15.04653450569339945, 15.86159749907602112, 25.98046417659831775 ) ) ;
#24085=CARTESIAN_POINT ( 'NONE',  ( -7.025853678916861966, 45.22357666574267654, -26.06988505166722803 ) ) ;
#24091=CARTESIAN_POINT ( 'NONE',  ( -6.950374756619716266, 54.97434000092398065, -26.09010956794232428 ) ) ;
#24095=CARTESIAN_POINT ( 'NONE',  ( -26.00068869287368756, 22.16927083333332504, -15.01150461594595775 ) ) ;
#24099=CARTESIAN_POINT ( 'NONE',  ( -30.02300923189239512, 45.94531249999997868, 2.654126918244515359E-13 ) ) ;
#24105=CARTESIAN_POINT ( 'NONE',  ( -0.04044903255044120238, 65.99180583240935505, -30.02300923189239867 ) ) ;
#24109=CARTESIAN_POINT ( 'NONE',  ( -26.07999730980490583, 63.27604166666667140, -6.988114217767815717 ) ) ;
#24112=CARTESIAN_POINT ( 'NONE',  ( -26.07999730980490583, 28.90104166666666785, -6.988114217767815717 ) ) ;
#24118=CARTESIAN_POINT ( 'NONE',  ( 26.09010956794232428, 55.83371500092398065, -6.950374756619718042 ) ) ;
#24130=CARTESIAN_POINT ( 'NONE',  ( 0.04044903254993986036, 20.74256916759064495, -27.95245687107223986 ) ) ;
#24135=CARTESIAN_POINT ( 'NONE',  ( 28.01184896238290278, 54.39583333333332860, -7.505752307973347470 ) ) ;
#24139=CARTESIAN_POINT ( 'NONE',  ( 15.01150461594643204, 20.73697916666666075, 26.00068869287340334 ) ) ;
#24145=CARTESIAN_POINT ( 'NONE',  ( -20.47846945139866648, 33.76524333240934084, 20.53372385742108008 ) ) ;
#24147=CARTESIAN_POINT ( 'NONE',  ( 20.50609665441005092, 44.65624999999999289, 20.50609665440969209 ) ) ;
#24150=CARTESIAN_POINT ( 'NONE',  ( -27.95245687107223986, 61.69493083240936926, 0.04044903255043252877 ) ) ;
#24157=CARTESIAN_POINT ( 'NONE',  ( -13.97622843553588901, 17.87239583333332860, 24.20753774853756823 ) ) ;
#24164=CARTESIAN_POINT ( 'NONE',  ( -13.94119854578892514, 26.74701416574268720, 24.22776226481266448 ) ) ;
#24167=CARTESIAN_POINT ( 'NONE',  ( 6.988114217768294445, 55.25520833333333570, 26.07999730980477437 ) ) ;
#24171=CARTESIAN_POINT ( 'NONE',  ( -2.584737979205441561E-13, 22.74218749999999645, -30.02300923189239512 ) ) ;
#24172=CARTESIAN_POINT ( 'NONE',  ( -15.04653450569291984, 19.31027750092397710, 25.98046417659859486 ) ) ;
#24195=CARTESIAN_POINT ( 'NONE',  ( 14.01125832528286352, 38.21652750092398065, -24.18731323226246843 ) ) ;
#24203=CARTESIAN_POINT ( 'NONE',  ( -30.02300923189239867, 58.25743083240935505, 0.04044903255044988294 ) ) ;
#24206=CARTESIAN_POINT ( 'NONE',  ( 26.07999730980490227, 27.18229166666666430, 6.988114217767821046 ) ) ;
#24209=CARTESIAN_POINT ( 'NONE',  ( -15.01150461594595775, 28.18489583333332860, 26.00068869287368756 ) ) ;
#24213=CARTESIAN_POINT ( 'NONE',  ( 7.543491769121427382, 41.51079833425730214, -28.00173670424548433 ) ) ;
#24216=CARTESIAN_POINT ( 'NONE',  ( 20.50609665440969565, 50.67187500000000000, -20.50609665441004736 ) ) ;
#24236=CARTESIAN_POINT ( 'NONE',  ( 13.97622843553633665, 65.42447916666667140, 24.20753774853730889 ) ) ;
#24241=CARTESIAN_POINT ( 'NONE',  ( -24.20753774853756823, 53.10677083333332149, -13.97622843553588723 ) ) ;
#24242=CARTESIAN_POINT ( 'NONE',  ( -20.47846945139902175, 30.62538166759064495, -20.53372385742072481 ) ) ;
#24243=CARTESIAN_POINT ( 'NONE',  ( 26.02091320914876960, 25.88763916574269075, 14.97647472619900455 ) ) ;
#24247=CARTESIAN_POINT ( 'NONE',  ( -14.01125832528328985, 45.08034749907603356, -24.18731323226223040 ) ) ;
#24254=CARTESIAN_POINT ( 'NONE',  ( -24.18731323226248264, 51.10715250092397355, -14.01125832528284931 ) ) ;
#24259=CARTESIAN_POINT ( 'NONE',  ( 26.00068869287340334, 23.31510416666666430, -15.01150461594642316 ) ) ;
#24265=CARTESIAN_POINT ( 'NONE',  ( -28.01184896238290278, 59.55208333333332149, 7.505752307973363457 ) ) ;
#24271=CARTESIAN_POINT ( 'NONE',  ( -20.47846945139866648, 68.14024333240935505, 20.53372385742108008 ) ) ;
#24278=CARTESIAN_POINT ( 'NONE',  ( -2.428612866367529427E-13, 39.92968750000000000, -27.95245687107222921 ) ) ;
#24284=CARTESIAN_POINT ( 'NONE',  ( 0.04044903254993986036, 55.11756916759064495, -27.95245687107223986 ) ) ;
#24286=CARTESIAN_POINT ( 'NONE',  ( -30.02300923189239512, 52.82031249999997868, 2.654126918244515359E-13 ) ) ;
#24298=CARTESIAN_POINT ( 'NONE',  ( -19.06425588902591173, 23.75038166759064140, -19.11951029504763611 ) ) ;
#24302=CARTESIAN_POINT ( 'NONE',  ( -26.00068869287340334, 49.09635416666665719, 15.01150461594643382 ) ) ;
#24305=CARTESIAN_POINT ( 'NONE',  ( -26.00068869287340334, 25.03385416666666785, 15.01150461594643382 ) ) ;
#24311=CARTESIAN_POINT ( 'NONE',  ( -20.47846945139866648, 40.64024333240936215, 20.53372385742108008 ) ) ;
#24313=CARTESIAN_POINT ( 'NONE',  ( -20.50609665441004736, 49.81249999999999289, -20.50609665440969565 ) ) ;
#24316=CARTESIAN_POINT ( 'NONE',  ( -6.950374756619247307, 57.54128499907602645, 26.09010956794245217 ) ) ;
#24323=CARTESIAN_POINT ( 'NONE',  ( -26.07999730980477437, 18.30208333333332860, 6.988114217768305103 ) ) ;
#24330=CARTESIAN_POINT ( 'NONE',  ( -0.04044903255042732459, 24.74180583240935505, -27.95245687107223986 ) ) ;
#24335=CARTESIAN_POINT ( 'NONE',  ( -24.20753774853756823, 49.66927083333330728, -13.97622843553588723 ) ) ;
#24341=CARTESIAN_POINT ( 'NONE',  ( -15.01150461594595775, 24.74739583333332504, 26.00068869287368756 ) ) ;
#24342=CARTESIAN_POINT ( 'NONE',  ( -7.543491769121417612, 22.60454833425730925, 28.00173670424549499 ) ) ;
#24362=CARTESIAN_POINT ( 'NONE',  ( 14.01125832528286352, 34.77902750092397355, -24.18731323226246843 ) ) ;
#24369=CARTESIAN_POINT ( 'NONE',  ( -0.04044903255044120238, 59.11680583240937636, -30.02300923189239867 ) ) ;
#24373=CARTESIAN_POINT ( 'NONE',  ( -6.988114217767819270, 28.04166666666666075, 26.07999730980490583 ) ) ;
#24375=CARTESIAN_POINT ( 'NONE',  ( -2.584737979205441561E-13, 33.05468750000000000, -30.02300923189239512 ) ) ;
#24379=CARTESIAN_POINT ( 'NONE',  ( 30.02300923189239867, 45.66444416759065916, 0.04044903254992252006 ) ) ;
#24381=CARTESIAN_POINT ( 'NONE',  ( 15.01150461594643204, 55.11197916666664298, 26.00068869287340334 ) ) ;
#24398=CARTESIAN_POINT ( 'NONE',  ( 19.06425588902592239, 15.15663166759064495, 19.11951029504763611 ) ) ;
#24403=CARTESIAN_POINT ( 'NONE',  ( 13.97622843553589966, 53.96614583333333570, -24.20753774853756113 ) ) ;
#24404=CARTESIAN_POINT ( 'NONE',  ( 20.53372385742072481, 41.79725666759063785, -20.47846945139902175 ) ) ;
#24405=CARTESIAN_POINT ( 'NONE',  ( 0.04044903255045854962, 29.89805583240935860, 30.02300923189239867 ) ) ;
#24408=CARTESIAN_POINT ( 'NONE',  ( 6.950374756619257965, 59.26003499907601935, -26.09010956794244507 ) ) ;
#24414=CARTESIAN_POINT ( 'NONE',  ( 0.04044903254993986036, 48.24256916759064495, -27.95245687107223986 ) ) ;
#24418=CARTESIAN_POINT ( 'NONE',  ( -26.00068869287340334, 28.47135416666666075, 15.01150461594643382 ) ) ;
#24422=CARTESIAN_POINT ( 'NONE',  ( 2.740863092043355209E-13, 55.39843749999999289, 30.02300923189239512 ) ) ;
#24429=CARTESIAN_POINT ( 'NONE',  ( 0.04044903255044120238, 16.14805583240936215, 27.95245687107223276 ) ) ;
#24436=CARTESIAN_POINT ( 'NONE',  ( -13.97622843553588901, 41.93489583333333570, 24.20753774853756823 ) ) ;
#24442=CARTESIAN_POINT ( 'NONE',  ( 6.950374756619721595, 63.56809000092398065, 26.09010956794232428 ) ) ;
#24444=CARTESIAN_POINT ( 'NONE',  ( 15.01150461594596308, 57.40364583333333570, -26.00068869287367335 ) ) ;
#24456=CARTESIAN_POINT ( 'NONE',  ( 14.01125832528286352, 21.02902750092397710, -24.18731323226246843 ) ) ;
#24461=CARTESIAN_POINT ( 'NONE',  ( -15.01150461594595775, 52.24739583333332860, 26.00068869287368756 ) ) ;
#24465=CARTESIAN_POINT ( 'NONE',  ( -7.505752307972844761, 34.91666666666666430, 28.01184896238304134 ) ) ;
#24471=CARTESIAN_POINT ( 'NONE',  ( 25.98046417659831775, 45.93972249907602645, -15.04653450569338879 ) ) ;
#24473=CARTESIAN_POINT ( 'NONE',  ( 28.01184896238304134, 51.24479166666666430, 7.505752307972846538 ) ) ;
#24477=CARTESIAN_POINT ( 'NONE',  ( -19.09188309203694445, 11.99999999999999645, -19.09188309203661049 ) ) ;
#24483=CARTESIAN_POINT ( 'NONE',  ( -6.988114217768288228, 22.59895833333332860, -26.07999730980477437 ) ) ;
#24491=CARTESIAN_POINT ( 'NONE',  ( 26.06988505166722803, 32.33295166574267654, -7.025853678916862854 ) ) ;
#24495=CARTESIAN_POINT ( 'NONE',  ( -24.20753774853730889, 52.53385416666666430, 13.97622843553633842 ) ) ;
#24500=CARTESIAN_POINT ( 'NONE',  ( 20.50609665440969565, 19.73437500000000000, -20.50609665441004736 ) ) ;
#24501=CARTESIAN_POINT ( 'NONE',  ( -26.02091320914849959, 23.03423583425731280, 14.97647472619947528 ) ) ;
#24510=CARTESIAN_POINT ( 'NONE',  ( 30.02300923189239867, 55.97694416759064495, 0.04044903254992252006 ) ) ;
#24517=CARTESIAN_POINT ( 'NONE',  ( 19.11951029504797006, 46.65586833240934794, 19.06425588902558133 ) ) ;
#24523=CARTESIAN_POINT ( 'NONE',  ( 24.18731323226247554, 39.07590250092398065, 14.01125832528285997 ) ) ;
#24530=CARTESIAN_POINT ( 'NONE',  ( 20.47846945139867003, 56.10899333240935505, -20.53372385742107653 ) ) ;
#24534=CARTESIAN_POINT ( 'NONE',  ( -26.07999730980477437, 21.73958333333332860, 6.988114217768305103 ) ) ;
#24536=CARTESIAN_POINT ( 'NONE',  ( -30.02300923189239512, 28.75781249999999645, 2.654126918244515359E-13 ) ) ;
#24539=CARTESIAN_POINT ( 'NONE',  ( -15.04653450569291984, 53.68527750092398065, 25.98046417659859486 ) ) ;
#24541=CARTESIAN_POINT ( 'NONE',  ( 15.01150461594596308, 57.40364583333333570, -26.00068869287367335 ) ) ;
#24560=CARTESIAN_POINT ( 'NONE',  ( -24.22776226481240514, 16.15923583425731636, 13.94119854578937812 ) ) ;
#24566=CARTESIAN_POINT ( 'NONE',  ( 13.97622843553589966, 47.09114583333332860, -24.20753774853756113 ) ) ;
#24567=CARTESIAN_POINT ( 'NONE',  ( -26.02091320914849959, 40.22173583425730925, 14.97647472619947528 ) ) ;
#24569=CARTESIAN_POINT ( 'NONE',  ( -30.02300923189239867, 30.75743083240935505, 0.04044903255044988294 ) ) ;
#24572=CARTESIAN_POINT ( 'NONE',  ( -27.95245687107223986, 54.81993083240935505, 0.04044903255043252877 ) ) ;
#24578=CARTESIAN_POINT ( 'NONE',  ( -26.09010956794232428, 47.23996500092398065, 6.950374756619732253 ) ) ;
#24582=CARTESIAN_POINT ( 'NONE',  ( -20.50609665440969209, 35.20312500000000000, 20.50609665441005092 ) ) ;
#24586=CARTESIAN_POINT ( 'NONE',  ( -20.50609665440969209, 55.82812499999999289, 20.50609665441005092 ) ) ;
#24593=CARTESIAN_POINT ( 'NONE',  ( -30.02300923189239867, 68.56993083240934084, 0.04044903255044988294 ) ) ;
#24600=CARTESIAN_POINT ( 'NONE',  ( 27.95245687107222921, 40.78906249999998579, -2.463307335887066074E-13 ) ) ;
#24606=CARTESIAN_POINT ( 'NONE',  ( -26.06988505166735237, 64.71392333425730214, -7.025853678916388567 ) ) ;
#24607=CARTESIAN_POINT ( 'NONE',  ( -28.01184896238304134, 49.52604166666666430, -7.505752307972844761 ) ) ;
#24618=CARTESIAN_POINT ( 'NONE',  ( 27.95245687107223986, 28.47694416759064495, 0.04044903254993640479 ) ) ;
#24624=CARTESIAN_POINT ( 'NONE',  ( 30.02300923189239512, 51.10156249999998579, -2.619432448724977703E-13 ) ) ;
#24628=CARTESIAN_POINT ( 'NONE',  ( 28.01184896238290278, 26.89583333333332860, -7.505752307973347470 ) ) ;
#24633=CARTESIAN_POINT ( 'NONE',  ( 20.53372385742108008, 39.78086833240934794, 20.47846945139866648 ) ) ;
#24635=CARTESIAN_POINT ( 'NONE',  ( 7.505752307973351023, 62.13020833333334281, 28.01184896238290278 ) ) ;
#24637=CARTESIAN_POINT ( 'NONE',  ( 26.07999730980490227, 16.86979166666666075, 6.988114217767821046 ) ) ;
#24643=CARTESIAN_POINT ( 'NONE',  ( -24.20753774853756823, 29.04427083333332860, -13.97622843553588723 ) ) ;
#24649=CARTESIAN_POINT ( 'NONE',  ( -7.543491769121917656, 24.59857666574268720, -28.00173670424536354 ) ) ;
#24652=CARTESIAN_POINT ( 'NONE',  ( -26.06988505166722803, 27.17670166574268009, 7.025853678916877953 ) ) ;
#24656=CARTESIAN_POINT ( 'NONE',  ( -6.988114217768288228, 56.97395833333333570, -26.07999730980477437 ) ) ;
#24662=CARTESIAN_POINT ( 'NONE',  ( 26.00068869287340334, 23.31510416666666430, -15.01150461594642316 ) ) ;
#24663=CARTESIAN_POINT ( 'NONE',  ( -20.53372385742071771, 26.32850666759063785, 20.47846945139902530 ) ) ;
#24672=CARTESIAN_POINT ( 'NONE',  ( -7.543491769121417612, 60.41704833425730214, 28.00173670424549499 ) ) ;
#24675=CARTESIAN_POINT ( 'NONE',  ( -26.02091320914878025, 48.23138916574269786, -14.97647472619899389 ) ) ;
#24676=CARTESIAN_POINT ( 'NONE',  ( -20.50609665441004736, 25.74999999999999645, -20.50609665440969565 ) ) ;
#24680=CARTESIAN_POINT ( 'NONE',  ( -24.18731323226221974, 40.78347249907601935, 14.01125832528330406 ) ) ;
#24686=CARTESIAN_POINT ( 'NONE',  ( 24.22776226481241224, 41.94048583425730925, -13.94119854578936923 ) ) ;
#24689=UNCERTAINTY_MEASURE_WITH_UNIT (LENGTH_MEASURE( 1.000000000000000082E-05 ), #5485, 'distance_accuracy_value', 'NONE');
#24694=CARTESIAN_POINT ( 'NONE',  ( 28.02196122052058413, 56.68190999907602645, 7.468012846824272799 ) ) ;
#24697=CARTESIAN_POINT ( 'NONE',  ( -24.20753774853756823, 22.16927083333332504, -13.97622843553588723 ) ) ;
#24700=CARTESIAN_POINT ( 'NONE',  ( -30.02300923189239512, 32.19531250000000000, 2.654126918244515359E-13 ) ) ;
#24703=CARTESIAN_POINT ( 'NONE',  ( 30.02300923189239867, 52.53944416759064495, 0.04044903254992252006 ) ) ;
#24705=CARTESIAN_POINT ( 'NONE',  ( -2.584737979205441561E-13, 63.99218749999997868, -30.02300923189239512 ) ) ;
#24726=CARTESIAN_POINT ( 'NONE',  ( -7.025853678916393008, 12.29204833425730925, 26.06988505166735592 ) ) ;
#24731=CARTESIAN_POINT ( 'NONE',  ( -24.20753774853756823, 49.66927083333332149, -13.97622843553588723 ) ) ;
#24732=CARTESIAN_POINT ( 'NONE',  ( 20.53372385742072481, 34.92225666759063074, -20.47846945139902175 ) ) ;
#24733=CARTESIAN_POINT ( 'NONE',  ( -20.53372385742107653, 31.18711833240935150, -20.47846945139867003 ) ) ;
#24736=CARTESIAN_POINT ( 'NONE',  ( -14.01125832528328985, 51.95534749907602645, -24.18731323226223040 ) ) ;
#24745=CARTESIAN_POINT ( 'NONE',  ( 7.505752307972854531, 36.63541666666666430, -28.01184896238303423 ) ) ;
#24750=CARTESIAN_POINT ( 'NONE',  ( 28.01184896238304134, 58.11979166666665719, 7.505752307972846538 ) ) ;
#24757=CARTESIAN_POINT ( 'NONE',  ( -28.02196122052058413, 68.71315999907601224, -7.468012846824272799 ) ) ;
#24765=CARTESIAN_POINT ( 'NONE',  ( 24.20753774853731244, 40.50260416666666430, -13.97622843553632599 ) ) ;
#24770=CARTESIAN_POINT ( 'NONE',  ( 13.94119854578937812, 63.42486083425730925, 24.22776226481240514 ) ) ;
#24771=CARTESIAN_POINT ( 'NONE',  ( -28.01184896238304134, 56.40104166666666430, -7.505752307972844761 ) ) ;
#24783=CARTESIAN_POINT ( 'NONE',  ( 19.11951029504763611, 31.48475666759063074, -19.06425588902591173 ) ) ;
#24788=CARTESIAN_POINT ( 'NONE',  ( 30.02300923189239512, 47.66406249999998579, -2.619432448724977703E-13 ) ) ;
#24792=CARTESIAN_POINT ( 'NONE',  ( -7.505752307973343918, 29.47395833333332860, -28.01184896238290989 ) ) ;
#24799=CARTESIAN_POINT ( 'NONE',  ( 15.04653450569339945, 43.36159749907602645, 25.98046417659831775 ) ) ;
#24801=CARTESIAN_POINT ( 'NONE',  ( -7.505752307972844761, 58.97916666666666430, 28.01184896238304134 ) ) ;
#24805=CARTESIAN_POINT ( 'NONE',  ( 24.22776226481265383, 67.13763916574266943, 13.94119854578893580 ) ) ;
#24813=CARTESIAN_POINT ( 'NONE',  ( -27.95245687107223276, 35.63281249999999289, 2.498001805406602216E-13 ) ) ;
#24817=CARTESIAN_POINT ( 'NONE',  ( 7.543491769121922985, 29.75482666574269075, 28.00173670424535644 ) ) ;
#24819=CARTESIAN_POINT ( 'NONE',  ( -14.01125832528328985, 41.64284749907602645, -24.18731323226223040 ) ) ;
#24822=CARTESIAN_POINT ( 'NONE',  ( 27.95245687107222921, 57.97656249999997868, -2.463307335887066074E-13 ) ) ;
#24827=CARTESIAN_POINT ( 'NONE',  ( -20.50609665441004736, 25.74999999999999645, -20.50609665440969565 ) ) ;
#24828=CARTESIAN_POINT ( 'NONE',  ( 28.00173670424549499, 25.18267333425730214, 7.543491769121417612 ) ) ;
#24838=CARTESIAN_POINT ( 'NONE',  ( -7.468012846824771955, 54.97434000092398065, -28.02196122052045624 ) ) ;
#24841=CARTESIAN_POINT ( 'NONE',  ( -28.01184896238304134, 28.90104166666666785, -7.505752307972844761 ) ) ;
#24846=CARTESIAN_POINT ( 'NONE',  ( 13.94119854578893580, 42.21576416574269075, -24.22776226481265383 ) ) ;
#24852=CARTESIAN_POINT ( 'NONE',  ( -26.06988505166735237, 50.96392333425730925, -7.025853678916388567 ) ) ;
#24860=CARTESIAN_POINT ( 'NONE',  ( -0.04044903255042732459, 14.42930583240935505, -27.95245687107223986 ) ) ;
#24863=CARTESIAN_POINT ( 'NONE',  ( 13.97622843553589966, 23.02864583333332149, -24.20753774853756113 ) ) ;
#24866=CARTESIAN_POINT ( 'NONE',  ( 30.02300923189239512, 27.03906250000000000, -2.619432448724977703E-13 ) ) ;
#24869=CARTESIAN_POINT ( 'NONE',  ( -20.53372385742071771, 46.95350666759064495, 20.47846945139902530 ) ) ;
#24871=CARTESIAN_POINT ( 'NONE',  ( 15.01150461594643204, 58.54947916666665009, 26.00068869287340334 ) ) ;
#24891=CARTESIAN_POINT ( 'NONE',  ( -27.95245687107222921, 66.57031250000000000, 2.498001805406602216E-13 ) ) ;
#24896=CARTESIAN_POINT ( 'NONE',  ( 6.988114217768294445, 51.81770833333332860, 26.07999730980477437 ) ) ;
#24898=CARTESIAN_POINT ( 'NONE',  ( 25.98046417659858420, 39.07590250092398065, 15.04653450569292872 ) ) ;
#24899=CARTESIAN_POINT ( 'NONE',  ( 15.04653450569339945, 26.17409749907601935, 25.98046417659831775 ) ) ;
#24904=CARTESIAN_POINT ( 'NONE',  ( 14.01125832528330051, 53.67409749907601935, 24.18731323226221974 ) ) ;
#24912=CARTESIAN_POINT ( 'NONE',  ( -20.50609665441004736, 32.62500000000000000, -20.50609665440969565 ) ) ;
#24917=CARTESIAN_POINT ( 'NONE',  ( 20.50609665440969565, 60.98437499999999289, -20.50609665441004736 ) ) ;
#24925=CARTESIAN_POINT ( 'NONE',  ( 7.025853678916867295, 19.44232666574268364, 26.06988505166722803 ) ) ;
#24933=CARTESIAN_POINT ( 'NONE',  ( -24.20753774853730889, 42.22135416666666430, 13.97622843553633842 ) ) ;
#24938=CARTESIAN_POINT ( 'NONE',  ( -25.98046417659859486, 13.29465250092397532, -15.04653450569291628 ) ) ;
#24939=CARTESIAN_POINT ( 'NONE',  ( -15.01150461594642138, 56.83072916666665009, -26.00068869287340334 ) ) ;
#24952=CARTESIAN_POINT ( 'NONE',  ( 27.95245687107223986, 31.91444416759064495, 0.04044903254993640479 ) ) ;
#24956=ORIENTED_EDGE ( 'NONE', *, *, #1024, .F. ) ;
#24957=CARTESIAN_POINT ( 'NONE',  ( -20.50609665440969209, 59.26562500000000000, 20.50609665441005092 ) ) ;
#24963=CARTESIAN_POINT ( 'NONE',  ( -28.01184896238290278, 32.05208333333332860, 7.505752307973363457 ) ) ;
#24968=CARTESIAN_POINT ( 'NONE',  ( 20.53372385742108008, 46.65586833240934794, 20.47846945139866648 ) ) ;
#24970=CARTESIAN_POINT ( 'NONE',  ( -15.01150461594595775, 59.12239583333333570, 26.00068869287368756 ) ) ;
#24974=CARTESIAN_POINT ( 'NONE',  ( 26.07999730980490227, 13.43229166666666607, 6.988114217767821046 ) ) ;
#24986=CARTESIAN_POINT ( 'NONE',  ( -15.04653450569338524, 21.01784749907601579, -25.98046417659831775 ) ) ;
#24989=CARTESIAN_POINT ( 'NONE',  ( -0.04044903255042732459, 35.05430583240935505, -27.95245687107223986 ) ) ;
#24993=CARTESIAN_POINT ( 'NONE',  ( 24.20753774853756113, 58.26302083333332149, 13.97622843553589789 ) ) ;
#24999=CARTESIAN_POINT ( 'NONE',  ( 20.50609665440969565, 30.04687500000000000, -20.50609665441004736 ) ) ;
#25000=CARTESIAN_POINT ( 'NONE',  ( -26.02091320914849959, 29.90923583425730925, 14.97647472619947528 ) ) ;
#25009=CARTESIAN_POINT ( 'NONE',  ( -28.00173670424549499, 57.83892333425730214, -7.543491769121417612 ) ) ;
#25012=CARTESIAN_POINT ( 'NONE',  ( 20.50609665441005092, 30.90624999999999645, 20.50609665440969209 ) ) ;
#25018=CARTESIAN_POINT ( 'NONE',  ( 0.04044903255044120238, 43.64805583240936215, 27.95245687107223276 ) ) ;
#25024=CARTESIAN_POINT ( 'NONE',  ( 14.01125832528286352, 51.96652750092398065, -24.18731323226246843 ) ) ;
#25029=DIRECTION ( 'NONE',  ( 0.7069718413157916048, 0.01953538259431456675, -0.7069718413158002646 ) ) ;
#25031=CARTESIAN_POINT ( 'NONE',  ( 28.00173670424535644, 63.27045166574269075, -7.543491769121920321 ) ) ;
#25036=CARTESIAN_POINT ( 'NONE',  ( 26.07999730980490227, 34.05729166666666430, 6.988114217767821046 ) ) ;
#25039=CARTESIAN_POINT ( 'NONE',  ( 26.00068869287367335, 44.51302083333331439, 15.01150461594596308 ) ) ;
#25042=CARTESIAN_POINT ( 'NONE',  ( 20.53372385742072481, 52.10975666759065206, -20.47846945139902175 ) ) ;
#25045=CARTESIAN_POINT ( 'NONE',  ( 7.505752307973351023, 58.69270833333332860, 28.01184896238290278 ) ) ;
#25063=CARTESIAN_POINT ( 'NONE',  ( 27.95245687107223986, 21.60194416759064495, 0.04044903254993640479 ) ) ;
#25068=CARTESIAN_POINT ( 'NONE',  ( -13.97622843553588901, 55.68489583333332860, 24.20753774853756823 ) ) ;
#25069=CARTESIAN_POINT ( 'NONE',  ( 7.468012846824777284, 42.94309000092397355, 28.02196122052045268 ) ) ;
#25070=CARTESIAN_POINT ( 'NONE',  ( -20.47846945139866648, 33.76524333240934084, 20.53372385742108008 ) ) ;
#25073=CARTESIAN_POINT ( 'NONE',  ( 6.950374756619257965, 55.82253499907601935, -26.09010956794244507 ) ) ;
#25083=CARTESIAN_POINT ( 'NONE',  ( 30.02300923189239512, 30.47656250000000355, -2.619432448724977703E-13 ) ) ;
#25099=CARTESIAN_POINT ( 'NONE',  ( 26.09010956794244507, 25.74440999907601935, 6.950374756619249084 ) ) ;
#25108=CARTESIAN_POINT ( 'NONE',  ( 19.09188309203661049, 47.23437499999999289, -19.09188309203694445 ) ) ;
#25114=CARTESIAN_POINT ( 'NONE',  ( -20.53372385742071771, 12.57850666759064140, 20.47846945139902530 ) ) ;
#25115=CARTESIAN_POINT ( 'NONE',  ( -15.01150461594642138, 60.26822916666665009, -26.00068869287340334 ) ) ;
#25124=CARTESIAN_POINT ( 'NONE',  ( 26.09010956794232428, 35.20871500092396644, -6.950374756619718042 ) ) ;
#25129=CARTESIAN_POINT ( 'NONE',  ( 20.50609665441005092, 65.28125000000000000, 20.50609665440969209 ) ) ;
#25133=CARTESIAN_POINT ( 'NONE',  ( -2.584737979205441561E-13, 33.05468750000000000, -30.02300923189239512 ) ) ;
#25139=CARTESIAN_POINT ( 'NONE',  ( 30.02300923189239867, 49.66368083240936215, -0.04044903255044467877 ) ) ;
#25141=CARTESIAN_POINT ( 'NONE',  ( -26.00068869287340334, 59.40885416666666430, 15.01150461594643559 ) ) ;
#25146=CARTESIAN_POINT ( 'NONE',  ( -13.97622843553588901, 17.87239583333332149, 24.20753774853756823 ) ) ;
#25156=CARTESIAN_POINT ( 'NONE',  ( 20.47846945139867003, 25.17149333240934439, -20.53372385742107653 ) ) ;
#25158=CARTESIAN_POINT ( 'NONE',  ( 26.06988505166722803, 35.77045166574266943, -7.025853678916862854 ) ) ;
#25162=CARTESIAN_POINT ( 'NONE',  ( -24.20753774853756823, 59.98177083333332149, -13.97622843553588723 ) ) ;
#25167=CARTESIAN_POINT ( 'NONE',  ( 20.50609665440969565, 36.92187499999999289, -20.50609665441004736 ) ) ;
#25168=CARTESIAN_POINT ( 'NONE',  ( -7.468012846824771955, 34.34934000092397355, -28.02196122052045624 ) ) ;
#25179=CARTESIAN_POINT ( 'NONE',  ( -15.04653450569291984, 57.12277750092398065, 25.98046417659859486 ) ) ;
#25182=CARTESIAN_POINT ( 'NONE',  ( 28.01184896238290278, 26.89583333333332860, -7.505752307973347470 ) ) ;
#25188=CARTESIAN_POINT ( 'NONE',  ( 6.950374756619257965, 45.51003499907601935, -26.09010956794244507 ) ) ;
#25194=CARTESIAN_POINT ( 'NONE',  ( 19.11951029504763611, 48.67225666759065206, -19.06425588902591173 ) ) ;
#25201=CARTESIAN_POINT ( 'NONE',  ( 0.04044903255045854962, 60.83555583240935505, 30.02300923189239867 ) ) ;
#25207=CARTESIAN_POINT ( 'NONE',  ( -6.988114217767819270, 31.47916666666666075, 26.07999730980490583 ) ) ;
#25210=CARTESIAN_POINT ( 'NONE',  ( -20.50609665441004736, 39.49999999999999289, -20.50609665440969565 ) ) ;
#25213=CARTESIAN_POINT ( 'NONE',  ( 20.53372385742072481, 62.42225666759065206, -20.47846945139902175 ) ) ;
#25214=CARTESIAN_POINT ( 'NONE',  ( -27.95245687107223986, 61.13319416759063785, -0.04044903254993292840 ) ) ;
#25217=CARTESIAN_POINT ( 'NONE',  ( 7.505752307972854531, 57.26041666666666430, -28.01184896238303423 ) ) ;
#25239=CARTESIAN_POINT ( 'NONE',  ( -13.94119854578936923, 20.45611083425730925, -24.22776226481241224 ) ) ;
#25244=CARTESIAN_POINT ( 'NONE',  ( 7.543491769121427382, 44.94829833425730925, -28.00173670424548433 ) ) ;
#25245=CARTESIAN_POINT ( 'NONE',  ( 20.53372385742108008, 39.78086833240934794, 20.47846945139866648 ) ) ;
#25248=CARTESIAN_POINT ( 'NONE',  ( 13.94119854578893580, 66.27826416574268364, -24.22776226481265383 ) ) ;
#25251=CARTESIAN_POINT ( 'NONE',  ( 20.50609665441005092, 13.71874999999999467, 20.50609665440969209 ) ) ;
#25258=CARTESIAN_POINT ( 'NONE',  ( 26.00068869287340334, 30.19010416666665719, -15.01150461594642316 ) ) ;
#25265=CARTESIAN_POINT ( 'NONE',  ( -30.02300923189239512, 63.13281250000000000, 2.654126918244515359E-13 ) ) ;
#25268=CARTESIAN_POINT ( 'NONE',  ( 28.01184896238304134, 13.43229166666666607, 7.505752307972846538 ) ) ;
#25273=CARTESIAN_POINT ( 'NONE',  ( 27.95245687107223276, 22.16368083240936215, -0.04044903255042905932 ) ) ;
#25282=CARTESIAN_POINT ( 'NONE',  ( -26.07999730980490583, 49.52604166666666430, -6.988114217767815717 ) ) ;
#25287=CARTESIAN_POINT ( 'NONE',  ( -30.02300923189239867, 16.44569416759064140, -0.04044903254991731589 ) ) ;
#25288=CARTESIAN_POINT ( 'NONE',  ( 7.505752307973351023, 58.69270833333332860, 28.01184896238290278 ) ) ;
#25297=CARTESIAN_POINT ( 'NONE',  ( -26.07999730980477437, 66.42708333333332860, 6.988114217768305103 ) ) ;
#25302=CARTESIAN_POINT ( 'NONE',  ( -24.18731323226248264, 30.48215250092397710, -14.01125832528284931 ) ) ;
#25309=CARTESIAN_POINT ( 'NONE',  ( -20.50609665441004736, 36.06250000000000000, -20.50609665440969565 ) ) ;
#25314=CARTESIAN_POINT ( 'NONE',  ( 7.468012846824281681, 55.82253499907601935, -28.02196122052058058 ) ) ;
#25316=CARTESIAN_POINT ( 'NONE',  ( 26.00068869287367690, 58.26302083333332860, 15.01150461594596486 ) ) ;
#25321=CARTESIAN_POINT ( 'NONE',  ( -27.95245687107222921, 25.32031250000000000, 2.498001805406602216E-13 ) ) ;
#25330=CARTESIAN_POINT ( 'NONE',  ( 14.97647472619900455, 28.46576416574268720, -26.02091320914876960 ) ) ;
#25332=CARTESIAN_POINT ( 'NONE',  ( 14.01125832528330051, 39.92409749907602645, 24.18731323226221974 ) ) ;
#25336=CARTESIAN_POINT ( 'NONE',  ( 6.988114217767829928, 60.69791666666667140, -26.07999730980489872 ) ) ;
#25342=CARTESIAN_POINT ( 'NONE',  ( -2.584737979205441561E-13, 29.61718749999999645, -30.02300923189239512 ) ) ;
#25343=CARTESIAN_POINT ( 'NONE',  ( 20.53372385742072481, 31.48475666759063074, -20.47846945139902175 ) ) ;
#25352=CARTESIAN_POINT ( 'NONE',  ( 26.00068869287340334, 13.00260416666666430, -15.01150461594642316 ) ) ;
#25355=CARTESIAN_POINT ( 'NONE',  ( -30.02300923189239867, 32.19531250000000000, 2.654126918244514854E-13 ) ) ;
#25361=CARTESIAN_POINT ( 'NONE',  ( -24.22776226481266448, 55.10638916574269786, -13.94119854578892514 ) ) ;
#25368=CARTESIAN_POINT ( 'NONE',  ( 27.95245687107223986, 52.53944416759064495, 0.04044903254993640479 ) ) ;
#25375=CARTESIAN_POINT ( 'NONE',  ( 7.543491769121922985, 67.56732666574268364, 28.00173670424535644 ) ) ;
#25381=CARTESIAN_POINT ( 'NONE',  ( -24.20753774853730889, 38.78385416666665719, 13.97622843553633842 ) ) ;
#25386=CARTESIAN_POINT ( 'NONE',  ( -15.01150461594595775, 38.49739583333332860, 26.00068869287368756 ) ) ;
#25389=CARTESIAN_POINT ( 'NONE',  ( -28.00173670424549499, 61.27642333425730925, -7.543491769121417612 ) ) ;
#25390=CARTESIAN_POINT ( 'NONE',  ( 19.06425588902592239, 56.40663166759065206, 19.11951029504763611 ) ) ;
#25392=CARTESIAN_POINT ( 'NONE',  ( 30.02300923189239867, 15.28868083240935505, -0.04044903255044467877 ) ) ;
#25412=CARTESIAN_POINT ( 'NONE',  ( -24.22776226481240514, 23.03423583425731280, 13.94119854578937812 ) ) ;
#25418=CARTESIAN_POINT ( 'NONE',  ( 30.02300923189239867, 49.10194416759064495, 0.04044903254992252006 ) ) ;
#25420=CARTESIAN_POINT ( 'NONE',  ( -15.04653450569338524, 34.76784749907601935, -25.98046417659831775 ) ) ;
#25424=CARTESIAN_POINT ( 'NONE',  ( -14.01125832528328985, 62.26784749907602645, -24.18731323226223040 ) ) ;
#25427=CARTESIAN_POINT ( 'NONE',  ( -15.01150461594642138, 15.58072916666666607, -26.00068869287340334 ) ) ;
#25435=CARTESIAN_POINT ( 'NONE',  ( -15.01150461594595775, 41.93489583333333570, 26.00068869287368756 ) ) ;
#25444=CARTESIAN_POINT ( 'NONE',  ( -15.01150461594642316, 15.58072916666666430, -26.00068869287341045 ) ) ;
#25449=CARTESIAN_POINT ( 'NONE',  ( 26.06988505166722803, 25.45795166574268364, -7.025853678916862854 ) ) ;
#25458=CARTESIAN_POINT ( 'NONE',  ( 26.07999730980477437, 50.95833333333332860, -6.988114217768290004 ) ) ;
#25462=CARTESIAN_POINT ( 'NONE',  ( -26.07999730980477437, 28.61458333333333215, 6.988114217768305103 ) ) ;
#25464=CARTESIAN_POINT ( 'NONE',  ( -28.02196122052045268, 19.73996500092397355, 7.468012846824790607 ) ) ;
#25465=CARTESIAN_POINT ( 'NONE',  ( -2.584737979205441561E-13, 63.99218749999997868, -30.02300923189239512 ) ) ;
#25476=CARTESIAN_POINT ( 'NONE',  ( 14.01125832528286352, 31.34152750092398421, -24.18731323226246843 ) ) ;
#25485=CARTESIAN_POINT ( 'NONE',  ( -15.01150461594642138, 39.64322916666667140, -26.00068869287340334 ) ) ;
#25490=CARTESIAN_POINT ( 'NONE',  ( -20.53372385742107653, 51.81211833240936215, -20.47846945139867003 ) ) ;
#25492=CARTESIAN_POINT ( 'NONE',  ( 7.505752307973351023, 65.56770833333332860, 28.01184896238290278 ) ) ;
#25496=CARTESIAN_POINT ( 'NONE',  ( -6.988114217767819270, 24.60416666666666430, 26.07999730980490583 ) ) ;
#25503=CIRCLE ( 'NONE', #13460, 0.9999999999999988898 ) ;
#25508=CARTESIAN_POINT ( 'NONE',  ( 19.11951029504797006, 32.90586833240934794, 19.06425588902558133 ) ) ;
#25512=CARTESIAN_POINT ( 'NONE',  ( -6.988114217768288228, 60.41145833333332149, -26.07999730980477437 ) ) ;
#25518=CARTESIAN_POINT ( 'NONE',  ( 28.01184896238290278, 33.77083333333333570, -7.505752307973347470 ) ) ;
#25519=CARTESIAN_POINT ( 'NONE',  ( -15.04653450569291984, 29.62277750092397355, 25.98046417659859486 ) ) ;
#25531=CARTESIAN_POINT ( 'NONE',  ( 28.01184896238290278, 13.14583333333332860, -7.505752307973347470 ) ) ;
#25534=CARTESIAN_POINT ( 'NONE',  ( -7.505752307972844761, 28.04166666666666075, 28.01184896238304134 ) ) ;
#25538=CARTESIAN_POINT ( 'NONE',  ( 19.11951029504797006, 56.96836833240936215, 19.06425588902558133 ) ) ;
#25552=CARTESIAN_POINT ( 'NONE',  ( 7.543491769121922985, 60.69232666574269075, 28.00173670424535644 ) ) ;
#25554=CARTESIAN_POINT ( 'NONE',  ( -20.50609665441004736, 67.00000000000000000, -20.50609665440969565 ) ) ;
#25556=CARTESIAN_POINT ( 'NONE',  ( 26.07999730980490227, 37.49479166666666430, 6.988114217767821046 ) ) ;
#25560=CARTESIAN_POINT ( 'NONE',  ( -15.01150461594642138, 36.20572916666666430, -26.00068869287340334 ) ) ;
#25563=CARTESIAN_POINT ( 'NONE',  ( 25.98046417659858420, 59.70090250092397355, 15.04653450569292872 ) ) ;
#25564=CARTESIAN_POINT ( 'NONE',  ( -13.94119854578936923, 61.70611083425731636, -24.22776226481241224 ) ) ;
#25566=CARTESIAN_POINT ( 'NONE',  ( 14.97647472619900455, 18.15326416574268720, -26.02091320914876960 ) ) ;
#25585=CARTESIAN_POINT ( 'NONE',  ( 13.94119854578937812, 18.73736083425731636, 24.22776226481240514 ) ) ;
#25590=CARTESIAN_POINT ( 'NONE',  ( -7.468012846824771955, 44.66184000092397355, -28.02196122052045624 ) ) ;
#25593=CARTESIAN_POINT ( 'NONE',  ( -28.02196122052058413, 41.21315999907602645, -7.468012846824272799 ) ) ;
#25597=CARTESIAN_POINT ( 'NONE',  ( 13.94119854578893580, 62.84076416574269786, -24.22776226481265383 ) ) ;
#25607=CARTESIAN_POINT ( 'NONE',  ( 28.01184896238290278, 40.64583333333332860, -7.505752307973347470 ) ) ;
#25615=CARTESIAN_POINT ( 'NONE',  ( 28.01184896238304134, 16.86979166666666075, 7.505752307972846538 ) ) ;
#25621=CARTESIAN_POINT ( 'NONE',  ( -7.025853678916861966, 21.16107666574269075, -26.06988505166722803 ) ) ;
#25630=CARTESIAN_POINT ( 'NONE',  ( 2.584737979205441561E-13, 51.96093750000000000, 27.95245687107222921 ) ) ;
#25634=CARTESIAN_POINT ( 'NONE',  ( -6.988114217767819270, 31.47916666666666075, 26.07999730980490583 ) ) ;
#25635=CARTESIAN_POINT ( 'NONE',  ( 26.02091320914851025, 21.31548583425730925, -14.97647472619946463 ) ) ;
#25636=CARTESIAN_POINT ( 'NONE',  ( 28.01184896238290278, 64.70833333333334281, -7.505752307973347470 ) ) ;
#25646=CARTESIAN_POINT ( 'NONE',  ( -26.09010956794232428, 43.80246500092398776, 6.950374756619732253 ) ) ;
#25650=CARTESIAN_POINT ( 'NONE',  ( 15.01150461594596308, 12.71614583333333037, -26.00068869287367335 ) ) ;
#25654=CARTESIAN_POINT ( 'NONE',  ( 20.50609665441005092, 37.78124999999999289, 20.50609665440969209 ) ) ;
#25659=CARTESIAN_POINT ( 'NONE',  ( 15.04653450569339945, 50.23659749907603356, 25.98046417659831775 ) ) ;
#25661=CARTESIAN_POINT ( 'NONE',  ( 28.01184896238304134, 64.99479166666665719, 7.505752307972846538 ) ) ;
#25666=CARTESIAN_POINT ( 'NONE',  ( 13.97622843553589966, 23.02864583333332149, -24.20753774853756113 ) ) ;
#25681=CARTESIAN_POINT ( 'NONE',  ( 19.09188309203661049, 64.42187499999998579, -19.09188309203694445 ) ) ;
#25685=CARTESIAN_POINT ( 'NONE',  ( -26.00068869287340334, 31.90885416666666430, 15.01150461594643382 ) ) ;
#25696=CARTESIAN_POINT ( 'NONE',  ( 2.740863092043355209E-13, 14.14843749999999289, 30.02300923189239512 ) ) ;
#25699=CARTESIAN_POINT ( 'NONE',  ( -26.00068869287368756, 35.91927083333332860, -15.01150461594595775 ) ) ;
#25704=CARTESIAN_POINT ( 'NONE',  ( -0.04044903255042732459, 55.67930583240935505, -27.95245687107223986 ) ) ;
#25710=CARTESIAN_POINT ( 'NONE',  ( -13.97622843553588901, 14.43489583333332860, 24.20753774853756823 ) ) ;
#25718=CARTESIAN_POINT ( 'NONE',  ( -24.18731323226221974, 23.59597249907602290, 14.01125832528330406 ) ) ;
#25722=CARTESIAN_POINT ( 'NONE',  ( -6.988114217767819270, 38.35416666666666430, 26.07999730980490583 ) ) ;
#25726=CARTESIAN_POINT ( 'NONE',  ( -20.50609665441004736, 36.06250000000000000, -20.50609665440969565 ) ) ;
#25729=CARTESIAN_POINT ( 'NONE',  ( -28.02196122052045268, 57.55246500092398065, 7.468012846824790607 ) ) ;
#25730=CARTESIAN_POINT ( 'NONE',  ( 7.025853678916403666, 58.69829833425730925, -26.06988505166735237 ) ) ;
#25732=CARTESIAN_POINT ( 'NONE',  ( -20.53372385742107653, 17.43711833240935505, -20.47846945139867003 ) ) ;
#25751=CARTESIAN_POINT ( 'NONE',  ( -19.06425588902591173, 20.31288166759063785, -19.11951029504763611 ) ) ;
#25756=CARTESIAN_POINT ( 'NONE',  ( -20.53372385742071771, 50.39100666759063785, 20.47846945139902530 ) ) ;
#25758=CARTESIAN_POINT ( 'NONE',  ( -20.53372385742107653, 41.49961833240934794, -20.47846945139867003 ) ) ;
#25762=CARTESIAN_POINT ( 'NONE',  ( 14.01125832528330051, 67.42409749907601224, 24.18731323226221974 ) ) ;
#25768=ORIENTED_EDGE ( 'NONE', *, *, #1215, .T. ) ;
#25771=CARTESIAN_POINT ( 'NONE',  ( -7.505752307972844761, 45.22916666666665719, 28.01184896238304134 ) ) ;
#25772=CARTESIAN_POINT ( 'NONE',  ( 30.02300923189239512, 57.97656249999997868, -2.619432448724977703E-13 ) ) ;
#25785=CARTESIAN_POINT ( 'NONE',  ( 26.06988505166722803, 28.89545166574268009, -7.025853678916862854 ) ) ;
#25793=CARTESIAN_POINT ( 'NONE',  ( 19.09188309203661049, 54.10937499999999289, -19.09188309203694445 ) ) ;
#25797=CARTESIAN_POINT ( 'NONE',  ( -19.09188309203660694, 31.76562499999999289, 19.09188309203694800 ) ) ;
#25798=CARTESIAN_POINT ( 'NONE',  ( -30.02300923189239867, 23.32069416759064140, -0.04044903254991731589 ) ) ;
#25799=CARTESIAN_POINT ( 'NONE',  ( -28.01184896238304134, 63.27604166666667140, -7.505752307972844761 ) ) ;
#25806=EDGE_LOOP ( 'NONE', ( #14837, #25768, #27746, #9246 ) ) ;
#25810=CARTESIAN_POINT ( 'NONE',  ( -7.025853678916393008, 39.79204833425731636, 26.06988505166735592 ) ) ;
#25815=CARTESIAN_POINT ( 'NONE',  ( 15.01150461594643204, 13.86197916666666430, 26.00068869287340334 ) ) ;
#25819=CARTESIAN_POINT ( 'NONE',  ( -15.01150461594595775, 35.05989583333332860, 26.00068869287368756 ) ) ;
#25824=CARTESIAN_POINT ( 'NONE',  ( -0.04044903255044120238, 55.67930583240935505, -30.02300923189239867 ) ) ;
#25826=CARTESIAN_POINT ( 'NONE',  ( -15.01150461594642316, 63.70572916666667140, -26.00068869287341045 ) ) ;
#25831=CARTESIAN_POINT ( 'NONE',  ( 6.988114217768294445, 20.88020833333333215, 26.07999730980477437 ) ) ;
#25848=CARTESIAN_POINT ( 'NONE',  ( 7.025853678916403666, 17.44829833425730925, -26.06988505166735237 ) ) ;
#25852=CARTESIAN_POINT ( 'NONE',  ( -15.01150461594642138, 39.64322916666667140, -26.00068869287340334 ) ) ;
#25864=CARTESIAN_POINT ( 'NONE',  ( -7.468012846824771955, 61.84934000092397355, -28.02196122052045624 ) ) ;
#25866=CARTESIAN_POINT ( 'NONE',  ( -30.02300923189239867, 39.07031249999998579, 2.654126918244514854E-13 ) ) ;
#25871=CARTESIAN_POINT ( 'NONE',  ( 13.94119854578893580, 49.09076416574269786, -24.22776226481265383 ) ) ;
#25876=CARTESIAN_POINT ( 'NONE',  ( 19.09188309203694800, 17.15624999999999645, 19.09188309203660694 ) ) ;
#25883=CARTESIAN_POINT ( 'NONE',  ( -27.95245687107223986, 17.00743083240935860, 0.04044903255043252877 ) ) ;
#25887=CARTESIAN_POINT ( 'NONE',  ( 13.97622843553633665, 48.23697916666665719, 24.20753774853730889 ) ) ;
#25890=CARTESIAN_POINT ( 'NONE',  ( 15.01150461594643204, 48.23697916666665719, 26.00068869287340334 ) ) ;
#25892=CARTESIAN_POINT ( 'NONE',  ( 25.98046417659858420, 63.13840250092397355, 15.04653450569292872 ) ) ;
#25893=CARTESIAN_POINT ( 'NONE',  ( 13.94119854578937812, 59.98736083425730925, 24.22776226481240514 ) ) ;
#25899=CARTESIAN_POINT ( 'NONE',  ( 26.02091320914876960, 19.01263916574269075, 14.97647472619900455 ) ) ;
#25904=CARTESIAN_POINT ( 'NONE',  ( -15.01150461594595775, 65.99739583333334281, 26.00068869287368756 ) ) ;
#25919=CARTESIAN_POINT ( 'NONE',  ( -24.18731323226248264, 30.48215250092397710, -14.01125832528284931 ) ) ;
#25926=CARTESIAN_POINT ( 'NONE',  ( 20.47846945139867003, 45.79649333240935505, -20.53372385742107653 ) ) ;
#25930=CARTESIAN_POINT ( 'NONE',  ( -27.95245687107222921, 15.00781249999999467, 2.498001805406602216E-13 ) ) ;
#25933=CARTESIAN_POINT ( 'NONE',  ( 7.505752307973351023, 17.44270833333333215, 28.01184896238290278 ) ) ;
#25940=CARTESIAN_POINT ( 'NONE',  ( 26.00068869287340334, 43.94010416666665719, -15.01150461594642316 ) ) ;
#25941=CARTESIAN_POINT ( 'NONE',  ( 30.02300923189239512, 61.41406250000000711, -2.619432448724977703E-13 ) ) ;
#25956=CARTESIAN_POINT ( 'NONE',  ( 0.04044903255044120238, 29.89805583240935860, 27.95245687107223276 ) ) ;
#25964=CARTESIAN_POINT ( 'NONE',  ( -19.09188309203694445, 56.68749999999998579, -19.09188309203661049 ) ) ;
#25968=CARTESIAN_POINT ( 'NONE',  ( 13.97622843553633842, 44.79947916666667140, 24.20753774853730889 ) ) ;
#25970=CARTESIAN_POINT ( 'NONE',  ( 15.04653450569292872, 17.59152750092397355, -25.98046417659857710 ) ) ;
#25971=CARTESIAN_POINT ( 'NONE',  ( -20.47846945139866648, 16.57774333240934794, 20.53372385742108008 ) ) ;
#25974=AXIS2_PLACEMENT_3D ( 'NONE', #9393, #2714, #10272 ) ;
#25982=CARTESIAN_POINT ( 'NONE',  ( 27.95245687107223986, 38.78944416759064495, 0.04044903254993640479 ) ) ;
#25986=CARTESIAN_POINT ( 'NONE',  ( -15.01150461594595775, 17.87239583333332149, 26.00068869287368756 ) ) ;
#25990=CARTESIAN_POINT ( 'NONE',  ( -20.50609665441004736, 39.49999999999999289, -20.50609665440969565 ) ) ;
#25995=CARTESIAN_POINT ( 'NONE',  ( -25.98046417659831420, 61.40847249907603356, 15.04653450569339945 ) ) ;
#26000=CARTESIAN_POINT ( 'NONE',  ( 19.09188309203661049, 60.98437499999999289, -19.09188309203694445 ) ) ;
#26003=CARTESIAN_POINT ( 'NONE',  ( -6.988114217768288228, 26.03645833333333215, -26.07999730980477437 ) ) ;
#26011=CARTESIAN_POINT ( 'NONE',  ( -19.06425588902591173, 47.81288166759064495, -19.11951029504763611 ) ) ;
#26021=( BOUNDED_CURVE ( )  B_SPLINE_CURVE ( 2, ( #20820, #2096, #5014, #4330, #20130, #23215, #1919, #14803, #33675, #30574, #25268, #12569, #22694, #10173, #33849, #20299, #23040, #20656, #14975, #10001, #31264, #10344, #7759, #27846, #1741, #25444, #12221, #12396, #22867, #33324, #30749, #17727, #28184, #33498, #25615, #28860, #3125, #21486, #24063, #31599, #31933, #15837, #8426, #16007, #26122, #21156, #32559, #18245, #23892, #23722, #18584, #13082, #28692, #6320, #15673, #13597, #18915, #20986, #8258, #29024, #18750, #31765, #529, #29192, #26462, #2954, #10676, #29817, #2619, #5527, #5190, #23556, #5357, #26294, #13424, #22115, #363, #8097, #16175, #10849, #20, #11016, #5698, #21324, #26631, #16796, #27254, #10508, #11631, #31436, #7928, #18414, #3746, #2783, #13249, #14219, #24676, #1149, #189, #22607, #14722, #11968, #22956, #15066, #25182, #1660, #7158, #19867, #33061, #12312, #12135, #11802, #25534, #22439, #17641, #9219, #22784, #6990, #24841, #28102, #9735, #22280, #19703, #9565, #12487, #27760, #30321, #27933, #32886, #20044, #3913, #4417, #25012, #14894, #14382, #30149, #9385, #1319, #1494, #29986, #6491, #25355, #6818, #30489, #32723, #1834, #17299, #33236, #6652, #17133, #4248, #27589, #17473, #16964, #27422, #9058, #4589, #20221, #30661, #2011, #19538, #4078, #14553, #31351, #7509, #9911, #10425, #25699, #20388, #18161, #28273, #20903, #28946, #15411, #28603, #4759, #18502, #10260, #106, #28439, #31012, #2705, #30839, #33769, #10088, #13165, #4930, #15236, #2180, #25866, #12653, #26039, #2533, #10597, #23642, #23123, #7844, #2355, #17993, #5444, #13001, #21074, #12830, #17815, #23472, #33587, #23302, #18333, #20567, #5102, #15925, #20742, #8017, #7331, #15588, #5275, #31184, #31523, #15757, #7675, #28778, #33934, #26211, #26381, #2872, #13341, #33414, #948, #24147, #18671, #21903, #21745, #29110, #617, #5950, #3377, #32021, #32355, #16429, #32191, #26719, #10767, #8346, #11106, #11269, #18835, #3215, #31854, #8517, #26549, #14011, #5614, #23980, #19003, #8849, #19169, #29447, #16262, #26881, #451, #787, #10933, #13847, #27215, #24313, #21575, #16098, #8685, #19330, #5782, #29607, #3045, #29773, #6109, #24473, #29281, #21408, #27045, #16589, #31687, #13683, #3539, #11428, #13517, #6280, #16756, #3706, #23814, #279, #21244, #8181, #3871, #22565, #9179, #22239, #20176, #27720, #33016, #4208, #11931, #22401, #27382, #4036, #1617, #16922, #9341, #9696, #14344, #22742, #22072, #19826, #20003, #29946, #12267, #30450, #6450, #9522, #14680, #32849, #12095, #30278, #19498, #11758, #25316, #14511, #9016, #33193, #6948, #24801, #24970, #6779, #25141, #17258, #30620, #17431, #27892, #17090, #28060, #7116, #4376, #14850, #19663, #27549, #32684, #1789, #1278, #17598, #30106, #6612, #14178, #24635, #1108, #11593, #1452, #32516, #4717, #15545, #13125, #7635, #18117, #21033, #25826, #23433, #28401, #20702, #33372, #33893, #20527, #10385, #9868, #25661, #4890, #20345, #30970, #25492, #1971, #4547, #23600, #10223, #26172, #15717, #7803, #15023, #30795, #2490 ),
 .UNSPECIFIED., .F., .T. ) 
 B_SPLINE_CURVE_WITH_KNOTS ( ( 3, 2, 2, 2, 2, 2, 2, 2, 2, 2, 2, 2, 2, 2, 2, 2, 2, 2, 2, 2, 2, 2, 2, 2, 2, 2, 2, 2, 2, 2, 2, 2, 2, 2, 2, 2, 2, 2, 2, 2, 2, 2, 2, 2, 2, 2, 2, 2, 2, 2, 2, 2, 2, 2, 2, 2, 2, 2, 2, 2, 2, 2, 2, 2, 2, 2, 2, 2, 2, 2, 2, 2, 2, 2, 2, 2, 2, 2, 2, 2, 2, 2, 2, 2, 2, 2, 2, 2, 2, 2, 2, 2, 2, 2, 2, 2, 2, 2, 2, 2, 2, 2, 2, 2, 2, 2, 2, 2, 2, 2, 2, 2, 2, 2, 2, 2, 2, 2, 2, 2, 2, 2, 2, 2, 2, 2, 2, 2, 2, 2, 2, 2, 2, 2, 2, 2, 2, 2, 2, 2, 2, 2, 2, 2, 2, 2, 2, 2, 2, 2, 2, 2, 2, 2, 2, 2, 2, 2, 2, 2, 2, 2, 2, 2, 2, 2, 2, 2, 2, 2, 2, 2, 2, 2, 2, 2, 2, 2, 2, 2, 2, 2, 2, 2, 2, 2, 2, 2, 2, 2, 2, 2, 3 ),
 ( 0.000000000000000000, 0.005208333333333333044, 0.01041666666666666609, 0.01562500000000000000, 0.02083333333333333218, 0.02604166666666666782, 0.03125000000000000000, 0.03645833333333333565, 0.04166666666666666435, 0.04687500000000000000, 0.05208333333333333565, 0.05729166666666666435, 0.06250000000000000000, 0.06770833333333332871, 0.07291666666666667129, 0.07812500000000000000, 0.08333333333333332871, 0.08854166666666667129, 0.09375000000000000000, 0.09895833333333332871, 0.1041666666666666713, 0.1093750000000000000, 0.1145833333333333287, 0.1197916666666666713, 0.1250000000000000000, 0.1302083333333333426, 0.1354166666666666574, 0.1406250000000000000, 0.1458333333333333426, 0.1510416666666666574, 0.1562500000000000000, 0.1614583333333333426, 0.1666666666666666574, 0.1718750000000000000, 0.1770833333333333426, 0.1822916666666666574, 0.1875000000000000000, 0.1927083333333333426, 0.1979166666666666574, 0.2031250000000000000, 0.2083333333333333426, 0.2135416666666666574, 0.2187500000000000000, 0.2239583333333333426, 0.2291666666666666574, 0.2343750000000000000, 0.2395833333333333426, 0.2447916666666666574, 0.2500000000000000000, 0.2552083333333333148, 0.2604166666666666852, 0.2656250000000000000, 0.2708333333333333148, 0.2760416666666666852, 0.2812500000000000000, 0.2864583333333333148, 0.2916666666666666852, 0.2968750000000000000, 0.3020833333333333148, 0.3072916666666666852, 0.3125000000000000000, 0.3177083333333333148, 0.3229166666666666852, 0.3281250000000000000, 0.3333333333333333148, 0.3385416666666666852, 0.3437500000000000000, 0.3489583333333333148, 0.3541666666666666852, 0.3593750000000000000, 0.3645833333333333148, 0.3697916666666666852, 0.3750000000000000000, 0.3802083333333333148, 0.3854166666666666852, 0.3906250000000000000, 0.3958333333333333148, 0.4010416666666666852, 0.4062500000000000000, 0.4114583333333333148, 0.4166666666666666852, 0.4218750000000000000, 0.4270833333333333148, 0.4322916666666666852, 0.4375000000000000000, 0.4427083333333333148, 0.4479166666666666852, 0.4531250000000000000, 0.4583333333333333148, 0.4635416666666666852, 0.4687500000000000000, 0.4739583333333333148, 0.4791666666666666852, 0.4843750000000000000, 0.4895833333333333148, 0.4947916666666666852, 0.5000000000000000000, 0.5052083333333333703, 0.5104166666666666297, 0.5156250000000000000, 0.5208333333333333703, 0.5260416666666666297, 0.5312500000000000000, 0.5364583333333333703, 0.5416666666666666297, 0.5468750000000000000, 0.5520833333333333703, 0.5572916666666666297, 0.5625000000000000000, 0.5677083333333333703, 0.5729166666666666297, 0.5781250000000000000, 0.5833333333333333703, 0.5885416666666666297, 0.5937500000000000000, 0.5989583333333333703, 0.6041666666666666297, 0.6093750000000000000, 0.6145833333333333703, 0.6197916666666666297, 0.6250000000000000000, 0.6302083333333333703, 0.6354166666666666297, 0.6406250000000000000, 0.6458333333333333703, 0.6510416666666666297, 0.6562500000000000000, 0.6614583333333333703, 0.6666666666666666297, 0.6718750000000000000, 0.6770833333333333703, 0.6822916666666666297, 0.6875000000000000000, 0.6927083333333333703, 0.6979166666666666297, 0.7031250000000000000, 0.7083333333333333703, 0.7135416666666666297, 0.7187500000000000000, 0.7239583333333333703, 0.7291666666666666297, 0.7343750000000000000, 0.7395833333333333703, 0.7447916666666666297, 0.7500000000000000000, 0.7552083333333333703, 0.7604166666666666297, 0.7656250000000000000, 0.7708333333333333703, 0.7760416666666666297, 0.7812500000000000000, 0.7864583333333333703, 0.7916666666666666297, 0.7968750000000000000, 0.8020833333333333703, 0.8072916666666666297, 0.8125000000000000000, 0.8177083333333333703, 0.8229166666666666297, 0.8281250000000000000, 0.8333333333333333703, 0.8385416666666666297, 0.8437500000000000000, 0.8489583333333333703, 0.8541666666666666297, 0.8593750000000000000, 0.8645833333333333703, 0.8697916666666666297, 0.8750000000000000000, 0.8802083333333333703, 0.8854166666666666297, 0.8906250000000000000, 0.8958333333333333703, 0.9010416666666666297, 0.9062500000000000000, 0.9114583333333333703, 0.9166666666666666297, 0.9218750000000000000, 0.9270833333333333703, 0.9322916666666666297, 0.9375000000000000000, 0.9427083333333333703, 0.9479166666666666297, 0.9531250000000000000, 0.9583333333333333703, 0.9635416666666666297, 0.9687500000000000000, 0.9739583333333333703, 0.9791666666666666297, 0.9843750000000000000, 0.9895833333333333703, 0.9947916666666666297, 1.000000000000000000 ),
 .UNSPECIFIED. ) 
 CURVE ( )  GEOMETRIC_REPRESENTATION_ITEM ( )  RATIONAL_B_SPLINE_CURVE ( ( 1.000000000000000000, 0.9659258262890683122, 1.000000000000000000, 0.9659258262890683122, 1.000000000000000000, 0.9659258262890683122, 1.000000000000000000, 0.9659258262890683122, 1.000000000000000000, 0.9659258262890683122, 1.000000000000000000, 0.9659258262890683122, 1.000000000000000000, 0.9659258262890683122, 1.000000000000000000, 0.9659258262890683122, 1.000000000000000000, 0.9659258262890683122, 1.000000000000000000, 0.9659258262890683122, 1.000000000000000000, 0.9659258262890683122, 1.000000000000000000, 0.9659258262890683122, 1.000000000000000000, 0.9659258262890683122, 1.000000000000000000, 0.9659258262890683122, 1.000000000000000000, 0.9659258262890683122, 1.000000000000000000, 0.9659258262890683122, 1.000000000000000000, 0.9659258262890683122, 1.000000000000000000, 0.9659258262890683122, 1.000000000000000000, 0.9659258262890683122, 1.000000000000000000, 0.9659258262890683122, 1.000000000000000000, 0.9659258262890683122, 1.000000000000000000, 0.9659258262890683122, 1.000000000000000000, 0.9659258262890683122, 1.000000000000000000, 0.9659258262890683122, 1.000000000000000000, 0.9659258262890683122, 1.000000000000000000, 0.9659258262890683122, 1.000000000000000000, 0.9659258262890683122, 1.000000000000000000, 0.9659258262890683122, 1.000000000000000000, 0.9659258262890683122, 1.000000000000000000, 0.9659258262890683122, 1.000000000000000000, 0.9659258262890683122, 1.000000000000000000, 0.9659258262890683122, 1.000000000000000000, 0.9659258262890683122, 1.000000000000000000, 0.9659258262890683122, 1.000000000000000000, 0.9659258262890683122, 1.000000000000000000, 0.9659258262890683122, 1.000000000000000000, 0.9659258262890683122, 1.000000000000000000, 0.9659258262890683122, 1.000000000000000000, 0.9659258262890683122, 1.000000000000000000, 0.9659258262890683122, 1.000000000000000000, 0.9659258262890683122, 1.000000000000000000, 0.9659258262890683122, 1.000000000000000000, 0.9659258262890683122, 1.000000000000000000, 0.9659258262890683122, 1.000000000000000000, 0.9659258262890683122, 1.000000000000000000, 0.9659258262890683122, 1.000000000000000000, 0.9659258262890683122, 1.000000000000000000, 0.9659258262890683122, 1.000000000000000000, 0.9659258262890683122, 1.000000000000000000, 0.9659258262890683122, 1.000000000000000000, 0.9659258262890683122, 1.000000000000000000, 0.9659258262890683122, 1.000000000000000000, 0.9659258262890683122, 1.000000000000000000, 0.9659258262890683122, 1.000000000000000000, 0.9659258262890683122, 1.000000000000000000, 0.9659258262890683122, 1.000000000000000000, 0.9659258262890683122, 1.000000000000000000, 0.9659258262890683122, 1.000000000000000000, 0.9659258262890683122, 1.000000000000000000, 0.9659258262890683122, 1.000000000000000000, 0.9659258262890683122, 1.000000000000000000, 0.9659258262890683122, 1.000000000000000000, 0.9659258262890683122, 1.000000000000000000, 0.9659258262890683122, 1.000000000000000000, 0.9659258262890683122, 1.000000000000000000, 0.9659258262890683122, 1.000000000000000000, 0.9659258262890683122, 1.000000000000000000, 0.9659258262890683122, 1.000000000000000000, 0.9659258262890683122, 1.000000000000000000, 0.9659258262890683122, 1.000000000000000000, 0.9659258262890683122, 1.000000000000000000, 0.9659258262890683122, 1.000000000000000000, 0.9659258262890683122, 1.000000000000000000, 0.9659258262890683122, 1.000000000000000000, 0.9659258262890683122, 1.000000000000000000, 0.9659258262890683122, 1.000000000000000000, 0.9659258262890683122, 1.000000000000000000, 0.9659258262890683122, 1.000000000000000000, 0.9659258262890683122, 1.000000000000000000, 0.9659258262890683122, 1.000000000000000000, 0.9659258262890683122, 1.000000000000000000, 0.9659258262890683122, 1.000000000000000000, 0.9659258262890683122, 1.000000000000000000, 0.9659258262890683122, 1.000000000000000000, 0.9659258262890683122, 1.000000000000000000, 0.9659258262890683122, 1.000000000000000000, 0.9659258262890683122, 1.000000000000000000, 0.9659258262890683122, 1.000000000000000000, 0.9659258262890683122, 1.000000000000000000, 0.9659258262890683122, 1.000000000000000000, 0.9659258262890683122, 1.000000000000000000, 0.9659258262890683122, 1.000000000000000000, 0.9659258262890683122, 1.000000000000000000, 0.9659258262890683122, 1.000000000000000000, 0.9659258262890683122, 1.000000000000000000, 0.9659258262890683122, 1.000000000000000000, 0.9659258262890683122, 1.000000000000000000, 0.9659258262890683122, 1.000000000000000000, 0.9659258262890683122, 1.000000000000000000, 0.9659258262890683122, 1.000000000000000000, 0.9659258262890683122, 1.000000000000000000, 0.9659258262890683122, 1.000000000000000000, 0.9659258262890683122, 1.000000000000000000, 0.9659258262890683122, 1.000000000000000000, 0.9659258262890683122, 1.000000000000000000, 0.9659258262890683122, 1.000000000000000000, 0.9659258262890683122, 1.000000000000000000, 0.9659258262890683122, 1.000000000000000000, 0.9659258262890683122, 1.000000000000000000, 0.9659258262890683122, 1.000000000000000000, 0.9659258262890683122, 1.000000000000000000, 0.9659258262890683122, 1.000000000000000000, 0.9659258262890683122, 1.000000000000000000, 0.9659258262890683122, 1.000000000000000000, 0.9659258262890683122, 1.000000000000000000, 0.9659258262890683122, 1.000000000000000000, 0.9659258262890683122, 1.000000000000000000, 0.9659258262890683122, 1.000000000000000000, 0.9659258262890683122, 1.000000000000000000, 0.9659258262890683122, 1.000000000000000000, 0.9659258262890683122, 1.000000000000000000, 0.9659258262890683122, 1.000000000000000000, 0.9659258262890683122, 1.000000000000000000, 0.9659258262890683122, 1.000000000000000000, 0.9659258262890683122, 1.000000000000000000, 0.9659258262890683122, 1.000000000000000000, 0.9659258262890683122, 1.000000000000000000, 0.9659258262890683122, 1.000000000000000000, 0.9659258262890683122, 1.000000000000000000, 0.9659258262890683122, 1.000000000000000000, 0.9659258262890683122, 1.000000000000000000, 0.9659258262890683122, 1.000000000000000000, 0.9659258262890683122, 1.000000000000000000, 0.9659258262890683122, 1.000000000000000000, 0.9659258262890683122, 1.000000000000000000, 0.9659258262890683122, 1.000000000000000000, 0.9659258262890683122, 1.000000000000000000, 0.9659258262890683122, 1.000000000000000000, 0.9659258262890683122, 1.000000000000000000, 0.9659258262890683122, 1.000000000000000000, 0.9659258262890683122, 1.000000000000000000, 0.9659258262890683122, 1.000000000000000000, 0.9659258262890683122, 1.000000000000000000, 0.9659258262890683122, 1.000000000000000000, 0.9659258262890683122, 1.000000000000000000, 0.9659258262890683122, 1.000000000000000000, 0.9659258262890683122, 1.000000000000000000, 0.9659258262890683122, 1.000000000000000000, 0.9659258262890683122, 1.000000000000000000, 0.9659258262890683122, 1.000000000000000000, 0.9659258262890683122, 1.000000000000000000, 0.9659258262890683122, 1.000000000000000000, 0.9659258262890683122, 1.000000000000000000, 0.9659258262890683122, 1.000000000000000000, 0.9659258262890683122, 1.000000000000000000, 0.9659258262890683122, 1.000000000000000000, 0.9659258262890683122, 1.000000000000000000, 0.9659258262890683122, 1.000000000000000000, 0.9659258262890683122, 1.000000000000000000, 0.9659258262890683122, 1.000000000000000000, 0.9659258262890683122, 1.000000000000000000, 0.9659258262890683122, 1.000000000000000000, 0.9659258262890683122, 1.000000000000000000, 0.9659258262890683122, 1.000000000000000000, 0.9659258262890683122, 1.000000000000000000, 0.9659258262890683122, 1.000000000000000000, 0.9659258262890683122, 1.000000000000000000, 0.9659258262890683122, 1.000000000000000000, 0.9659258262890683122, 1.000000000000000000, 0.9659258262890683122, 1.000000000000000000, 0.9659258262890683122, 1.000000000000000000, 0.9659258262890683122, 1.000000000000000000, 0.9659258262890683122, 1.000000000000000000, 0.9659258262890683122, 1.000000000000000000, 0.9659258262890683122, 1.000000000000000000, 0.9659258262890683122, 1.000000000000000000, 0.9659258262890683122, 1.000000000000000000, 0.9659258262890683122, 1.000000000000000000, 0.9659258262890683122, 1.000000000000000000, 0.9659258262890683122, 1.000000000000000000, 0.9659258262890683122, 1.000000000000000000, 0.9659258262890683122, 1.000000000000000000, 0.9659258262890683122, 1.000000000000000000, 0.9659258262890683122, 1.000000000000000000, 0.9659258262890683122, 1.000000000000000000, 0.9659258262890683122, 1.000000000000000000, 0.9659258262890683122, 1.000000000000000000, 0.9659258262890683122, 1.000000000000000000, 0.9659258262890683122, 1.000000000000000000, 0.9659258262890683122, 1.000000000000000000, 0.9659258262890683122, 1.000000000000000000, 0.9659258262890683122, 1.000000000000000000 ) ) 
 REPRESENTATION_ITEM ( '' )  );
#26024=CARTESIAN_POINT ( 'NONE',  ( 13.94119854578937812, 11.86236083425730925, 24.22776226481240514 ) ) ;
#26028=CARTESIAN_POINT ( 'NONE',  ( -26.00068869287368756, 42.79427083333331439, -15.01150461594595775 ) ) ;
#26037=CARTESIAN_POINT ( 'NONE',  ( 20.50609665440969565, 12.85937500000000000, -20.50609665441004736 ) ) ;
#26039=CARTESIAN_POINT ( 'NONE',  ( -26.00068869287368756, 39.35677083333333570, -15.01150461594595775 ) ) ;
#26044=STYLED_ITEM ( 'NONE', ( #7908 ), #32186 ) ;
#26047=CARTESIAN_POINT ( 'NONE',  ( -19.06425588902558133, 54.39024333240934794, 19.11951029504797006 ) ) ;
#26061=CARTESIAN_POINT ( 'NONE',  ( 27.95245687107223276, 18.72618083240936215, -0.04044903255042905932 ) ) ;
#26065=CARTESIAN_POINT ( 'NONE',  ( -26.07999730980490583, 46.08854166666666430, -6.988114217767815717 ) ) ;
#26068=CARTESIAN_POINT ( 'NONE',  ( -20.50609665441004736, 46.37500000000000000, -20.50609665440969565 ) ) ;
#26070=CARTESIAN_POINT ( 'NONE',  ( 15.01150461594596308, 16.15364583333333215, -26.00068869287367335 ) ) ;
#26071=CARTESIAN_POINT ( 'NONE',  ( 26.02091320914851025, 17.87798583425730570, -14.97647472619946463 ) ) ;
#26078=CARTESIAN_POINT ( 'NONE',  ( 20.50609665441005092, 65.28125000000000000, 20.50609665440969209 ) ) ;
#26091=CARTESIAN_POINT ( 'NONE',  ( 19.06425588902592239, 32.34413166759064495, 19.11951029504763611 ) ) ;
#26098=CARTESIAN_POINT ( 'NONE',  ( -25.98046417659831420, 51.09597249907602645, 15.04653450569339945 ) ) ;
#26102=CARTESIAN_POINT ( 'NONE',  ( 26.07999730980490227, 20.30729166666666430, 6.988114217767821046 ) ) ;
#26105=CARTESIAN_POINT ( 'NONE',  ( 7.505752307972854531, 22.88541666666666430, -28.01184896238303423 ) ) ;
#26109=CARTESIAN_POINT ( 'NONE',  ( 28.00173670424549499, 42.37017333425730925, 7.543491769121417612 ) ) ;
#26111=CARTESIAN_POINT ( 'NONE',  ( -7.505752307972844761, 41.79166666666666430, 28.01184896238304134 ) ) ;
#26112=CARTESIAN_POINT ( 'NONE',  ( -7.505752307973343918, 63.84895833333332860, -28.01184896238290989 ) ) ;
#26122=CARTESIAN_POINT ( 'NONE',  ( -28.01184896238290278, 18.30208333333332860, 7.505752307973363457 ) ) ;
#26127=CARTESIAN_POINT ( 'NONE',  ( -19.06425588902558133, 33.76524333240934084, 19.11951029504797006 ) ) ;
#26135=CARTESIAN_POINT ( 'NONE',  ( 6.988114217767829928, 57.26041666666666430, -26.07999730980489872 ) ) ;
#26139=CARTESIAN_POINT ( 'NONE',  ( 26.07999730980477437, 44.08333333333332860, -6.988114217768290004 ) ) ;
#26140=CARTESIAN_POINT ( 'NONE',  ( 14.97647472619947351, 25.61236083425731636, 26.02091320914850314 ) ) ;
#26142=CARTESIAN_POINT ( 'NONE',  ( -26.02091320914878025, 17.29388916574268720, -14.97647472619899389 ) ) ;
#26146=CARTESIAN_POINT ( 'NONE',  ( -0.04044903255042732459, 45.36680583240934794, -27.95245687107223986 ) ) ;
#26154=CARTESIAN_POINT ( 'NONE',  ( 13.94119854578937812, 42.79986083425731636, 24.22776226481240514 ) ) ;
#26159=CARTESIAN_POINT ( 'NONE',  ( -2.584737979205441561E-13, 12.42968749999999289, -30.02300923189239512 ) ) ;
#26164=CARTESIAN_POINT ( 'NONE',  ( -26.00068869287368756, 53.10677083333331439, -15.01150461594595775 ) ) ;
#26166=DIRECTION ( 'NONE',  ( 0.7071067811865526798, 0.000000000000000000, 0.7071067811865423547 ) ) ;
#26170=CARTESIAN_POINT ( 'NONE',  ( 0.04044903255045854962, 60.83555583240935505, 30.02300923189239867 ) ) ;
#26172=CARTESIAN_POINT ( 'NONE',  ( -26.00068869287340334, 66.28385416666664298, 15.01150461594643559 ) ) ;
#26175=CARTESIAN_POINT ( 'NONE',  ( 24.20753774853756113, 58.26302083333332860, 13.97622843553589789 ) ) ;
#26178=CARTESIAN_POINT ( 'NONE',  ( -13.97622843553632421, 36.20572916666666430, -24.20753774853731599 ) ) ;
#26183=CARTESIAN_POINT ( 'NONE',  ( -26.09010956794232428, 57.55246500092398065, 6.950374756619732253 ) ) ;
#26194=CARTESIAN_POINT ( 'NONE',  ( 19.06425588902592239, 18.59413166759064140, 19.11951029504763611 ) ) ;
#26199=CARTESIAN_POINT ( 'NONE',  ( 15.01150461594643204, 41.36197916666666430, 26.00068869287340334 ) ) ;
#26203=CARTESIAN_POINT ( 'NONE',  ( 2.740863092043355209E-13, 17.58593749999999645, 30.02300923189239512 ) ) ;
#26209=CARTESIAN_POINT ( 'NONE',  ( 15.04653450569339945, 36.48659749907601935, 25.98046417659831775 ) ) ;
#26211=CARTESIAN_POINT ( 'NONE',  ( 20.50609665440969565, 43.79687500000000000, -20.50609665441004736 ) ) ;
#26218=CARTESIAN_POINT ( 'NONE',  ( 7.025853678916867295, 60.69232666574269075, 26.06988505166722803 ) ) ;
#26224=CARTESIAN_POINT ( 'NONE',  ( -2.428612866367529427E-13, 15.86718749999999822, -27.95245687107223276 ) ) ;
#26233=CARTESIAN_POINT ( 'NONE',  ( 26.06988505166722803, 15.14545166574268897, -7.025853678916862854 ) ) ;
#26237=CARTESIAN_POINT ( 'NONE',  ( -13.97622843553588901, 45.37239583333333570, 24.20753774853756823 ) ) ;
#26242=CARTESIAN_POINT ( 'NONE',  ( -15.01150461594595775, 17.87239583333332149, 26.00068869287368756 ) ) ;
#26243=CARTESIAN_POINT ( 'NONE',  ( -15.04653450569291984, 12.43527750092397532, 25.98046417659859486 ) ) ;
#26262=CARTESIAN_POINT ( 'NONE',  ( -14.01125832528285109, 29.62277750092397355, 24.18731323226248264 ) ) ;
#26269=CARTESIAN_POINT ( 'NONE',  ( -7.468012846824272799, 43.79128499907601935, 28.02196122052058413 ) ) ;
#26273=CARTESIAN_POINT ( 'NONE',  ( 6.988114217767829928, 12.57291666666666252, -26.07999730980489872 ) ) ;
#26276=CARTESIAN_POINT ( 'NONE',  ( -30.02300923189239512, 25.32031250000000000, 2.654126918244515359E-13 ) ) ;
#26280=CARTESIAN_POINT ( 'NONE',  ( -20.53372385742071771, 36.64100666759062364, 20.47846945139902530 ) ) ;
#26282=CARTESIAN_POINT ( 'NONE',  ( -20.50609665441004736, 56.68749999999998579, -20.50609665440969565 ) ) ;
#26294=CARTESIAN_POINT ( 'NONE',  ( -15.01150461594642316, 22.45572916666666430, -26.00068869287341045 ) ) ;
#26299=CARTESIAN_POINT ( 'NONE',  ( -26.09010956794245217, 30.90065999907601579, -6.950374756619243755 ) ) ;
#26306=CARTESIAN_POINT ( 'NONE',  ( 26.07999730980477437, 57.83333333333333570, -6.988114217768290004 ) ) ;
#26310=CARTESIAN_POINT ( 'NONE',  ( -19.09188309203660694, 38.64062500000000000, 19.09188309203694800 ) ) ;
#26311=CARTESIAN_POINT ( 'NONE',  ( 26.02091320914851025, 31.62798583425730925, -14.97647472619946463 ) ) ;
#26312=CARTESIAN_POINT ( 'NONE',  ( -28.02196122052058413, 20.58815999907601935, -7.468012846824272799 ) ) ;
#26316=CARTESIAN_POINT ( 'NONE',  ( 26.09010956794244507, 46.36940999907602645, 6.950374756619249084 ) ) ;
#26323=CARTESIAN_POINT ( 'NONE',  ( -19.11951029504763611, 43.51600666759065206, 19.06425588902592239 ) ) ;
#26327=CARTESIAN_POINT ( 'NONE',  ( 28.01184896238290278, 26.89583333333332860, -7.505752307973347470 ) ) ;
#26331=CARTESIAN_POINT ( 'NONE',  ( -20.50609665440969209, 48.95312500000000000, 20.50609665441005092 ) ) ;
#26332=DIRECTION ( 'NONE',  ( -0.7069718413157907166, -0.01953538259431455287, 0.7069718413158010417 ) ) ;
#26337=CARTESIAN_POINT ( 'NONE',  ( -28.00173670424535644, 58.11420166574269075, 7.543491769121936308 ) ) ;
#26342=CARTESIAN_POINT ( 'NONE',  ( 26.07999730980477437, 57.83333333333333570, -6.988114217768290004 ) ) ;
#26345=CARTESIAN_POINT ( 'NONE',  ( 13.97622843553633665, 31.04947916666666075, 24.20753774853730889 ) ) ;
#26351=CARTESIAN_POINT ( 'NONE',  ( -14.01125832528285109, 57.12277750092398065, 24.18731323226248264 ) ) ;
#26363=CARTESIAN_POINT ( 'NONE',  ( -24.22776226481240514, 12.72173583425731458, 13.94119854578937812 ) ) ;
#26369=CARTESIAN_POINT ( 'NONE',  ( -15.01150461594595775, 41.93489583333333570, 26.00068869287368756 ) ) ;
#26373=CARTESIAN_POINT ( 'NONE',  ( -26.00068869287368756, 22.16927083333332504, -15.01150461594595775 ) ) ;
#26379=CARTESIAN_POINT ( 'NONE',  ( 25.98046417659831775, 39.06472249907601935, -15.04653450569338879 ) ) ;
#26381=CARTESIAN_POINT ( 'NONE',  ( 26.00068869287341045, 43.94010416666665719, -15.01150461594642493 ) ) ;
#26387=CARTESIAN_POINT ( 'NONE',  ( -7.025853678916861966, 62.41107666574269075, -26.06988505166722803 ) ) ;
#26400=CARTESIAN_POINT ( 'NONE',  ( 24.18731323226221974, 21.87722249907602290, -14.01125832528328985 ) ) ;
#26405=CARTESIAN_POINT ( 'NONE',  ( -27.95245687107222921, 45.94531249999997868, 2.498001805406602216E-13 ) ) ;
#26409=CARTESIAN_POINT ( 'NONE',  ( 20.50609665441005092, 13.71874999999999467, 20.50609665440969209 ) ) ;
#26410=CARTESIAN_POINT ( 'NONE',  ( 20.53372385742072481, 14.29725666759064318, -20.47846945139902175 ) ) ;
#26430=CARTESIAN_POINT ( 'NONE',  ( 24.22776226481241224, 31.62798583425730925, -13.94119854578936923 ) ) ;
#26439=CARTESIAN_POINT ( 'NONE',  ( 20.53372385742108008, 50.09336833240935505, 20.47846945139866648 ) ) ;
#26444=CARTESIAN_POINT ( 'NONE',  ( 24.20753774853756113, 17.01302083333332504, 13.97622843553589789 ) ) ;
#26446=CARTESIAN_POINT ( 'NONE',  ( -2.584737979205441561E-13, 26.17968750000000000, -30.02300923189239512 ) ) ;
#26450=CARTESIAN_POINT ( 'NONE',  ( -30.02300923189239867, 40.50819416759064495, -0.04044903254991731589 ) ) ;
#26452=CARTESIAN_POINT ( 'NONE',  ( 7.505752307973351023, 51.81770833333332860, 28.01184896238290278 ) ) ;
#26462=CARTESIAN_POINT ( 'NONE',  ( -7.505752307972844761, 21.16666666666666430, 28.01184896238304134 ) ) ;
#26467=CARTESIAN_POINT ( 'NONE',  ( -14.01125832528328985, 38.20534749907601935, -24.18731323226223040 ) ) ;
#26474=CARTESIAN_POINT ( 'NONE',  ( -6.988114217767819270, 62.41666666666666430, 26.07999730980490583 ) ) ;
#26479=CARTESIAN_POINT ( 'NONE',  ( -26.07999730980490583, 39.21354166666666430, -6.988114217767815717 ) ) ;
#26480=CARTESIAN_POINT ( 'NONE',  ( 20.47846945139902530, 28.90663166759063785, 20.53372385742071771 ) ) ;
#26481=CARTESIAN_POINT ( 'NONE',  ( 26.02091320914876960, 22.45013916574269075, 14.97647472619900455 ) ) ;
#26485=CARTESIAN_POINT ( 'NONE',  ( -24.18731323226221974, 51.09597249907602645, 14.01125832528330406 ) ) ;
#26491=CARTESIAN_POINT ( 'NONE',  ( -27.95245687107223986, 54.25819416759065206, -0.04044903254993292840 ) ) ;
#26496=CARTESIAN_POINT ( 'NONE',  ( 28.01184896238304134, 23.74479166666666430, 7.505752307972846538 ) ) ;
#26500=CARTESIAN_POINT ( 'NONE',  ( 20.50609665441005092, 44.65624999999999289, 20.50609665440969209 ) ) ;
#26507=CARTESIAN_POINT ( 'NONE',  ( -20.53372385742107653, 58.68711833240935505, -20.47846945139867003 ) ) ;
#26512=CARTESIAN_POINT ( 'NONE',  ( 2.584737979205442066E-13, 58.83593750000000711, 27.95245687107223276 ) ) ;
#26515=CARTESIAN_POINT ( 'NONE',  ( -19.09188309203660694, 35.20312500000000000, 19.09188309203694800 ) ) ;
#26520=CARTESIAN_POINT ( 'NONE',  ( -6.950374756619716266, 58.41184000092398065, -26.09010956794232428 ) ) ;
#26533=CARTESIAN_POINT ( 'NONE',  ( -27.95245687107223986, 23.32069416759064140, -0.04044903254993292840 ) ) ;
#26538=CARTESIAN_POINT ( 'NONE',  ( -7.505752307972844761, 41.79166666666666430, 28.01184896238304134 ) ) ;
#26541=CARTESIAN_POINT ( 'NONE',  ( 30.02300923189239512, 23.60156250000000000, -2.619432448724977703E-13 ) ) ;
#26547=CARTESIAN_POINT ( 'NONE',  ( 20.47846945139867003, 35.48399333240935505, -20.53372385742107653 ) ) ;
#26549=CARTESIAN_POINT ( 'NONE',  ( 30.02300923189239867, 47.66406249999999289, -2.619432448724978208E-13 ) ) ;
#26555=CARTESIAN_POINT ( 'NONE',  ( -26.09010956794245217, 58.40065999907601935, -6.950374756619243755 ) ) ;
#26561=CARTESIAN_POINT ( 'NONE',  ( -26.07999730980490583, 22.02604166666666430, -6.988114217767815717 ) ) ;
#26570=CARTESIAN_POINT ( 'NONE',  ( 24.18731323226221974, 25.31472249907601579, -14.01125832528328985 ) ) ;
#26572=CARTESIAN_POINT ( 'NONE',  ( -6.988114217767819270, 41.79166666666666430, 26.07999730980490583 ) ) ;
#26578=CARTESIAN_POINT ( 'NONE',  ( -7.505752307973343918, 12.28645833333333037, -28.01184896238290989 ) ) ;
#26579=CARTESIAN_POINT ( 'NONE',  ( 14.97647472619947351, 18.73736083425731636, 26.02091320914850314 ) ) ;
#26600=CARTESIAN_POINT ( 'NONE',  ( -26.06988505166735237, 26.90142333425731280, -7.025853678916388567 ) ) ;
#26607=CARTESIAN_POINT ( 'NONE',  ( 20.53372385742108008, 43.21836833240935505, 20.47846945139866648 ) ) ;
#26611=CARTESIAN_POINT ( 'NONE',  ( 26.07999730980490227, 16.86979166666666075, 6.988114217767821046 ) ) ;
#26613=CARTESIAN_POINT ( 'NONE',  ( -7.505752307972844761, 17.72916666666666430, 28.01184896238304134 ) ) ;
#26617=CARTESIAN_POINT ( 'NONE',  ( -0.04044903254990864921, 36.21131916759064495, 30.02300923189239867 ) ) ;
#26620=CARTESIAN_POINT ( 'NONE',  ( 15.01150461594643204, 48.23697916666665719, 26.00068869287340334 ) ) ;
#26631=CARTESIAN_POINT ( 'NONE',  ( 20.50609665441005092, 24.03124999999999645, 20.50609665440969209 ) ) ;
#26642=CARTESIAN_POINT ( 'NONE',  ( -27.95245687107222921, 56.25781249999997868, 2.498001805406602216E-13 ) ) ;
#26647=CARTESIAN_POINT ( 'NONE',  ( 13.97622843553589966, 40.21614583333332860, -24.20753774853756113 ) ) ;
#26648=CARTESIAN_POINT ( 'NONE',  ( -0.04044903254990864921, 32.77381916759064495, 30.02300923189239867 ) ) ;
#26649=CARTESIAN_POINT ( 'NONE',  ( 0.04044903255045854962, 16.14805583240936215, 30.02300923189239867 ) ) ;
#26653=CARTESIAN_POINT ( 'NONE',  ( -0.04044903255042732459, 48.80430583240936215, -27.95245687107223986 ) ) ;
#26659=CARTESIAN_POINT ( 'NONE',  ( -24.22776226481240514, 53.97173583425732346, 13.94119854578937812 ) ) ;
#26663=CARTESIAN_POINT ( 'NONE',  ( 2.740863092043355209E-13, 24.46093749999999645, 30.02300923189239512 ) ) ;
#26668=CARTESIAN_POINT ( 'NONE',  ( -26.00068869287368756, 49.66927083333330728, -15.01150461594595775 ) ) ;
#26676=CARTESIAN_POINT ( 'NONE',  ( 30.02300923189239867, 63.41368083240934794, -0.04044903255044467877 ) ) ;
#26680=CARTESIAN_POINT ( 'NONE',  ( -24.20753774853730889, 62.84635416666667140, 13.97622843553634020 ) ) ;
#26683=CARTESIAN_POINT ( 'NONE',  ( -19.09188309203660694, 28.32812499999999645, 19.09188309203694800 ) ) ;
#26688=CARTESIAN_POINT ( 'NONE',  ( -0.04044903254992426173, 53.39881916759064495, 27.95245687107223276 ) ) ;
#26700=CARTESIAN_POINT ( 'NONE',  ( 7.025853678916403666, 27.76079833425730925, -26.06988505166735237 ) ) ;
#26706=CARTESIAN_POINT ( 'NONE',  ( -15.01150461594595775, 55.68489583333332860, 26.00068869287368756 ) ) ;
#26710=CARTESIAN_POINT ( 'NONE',  ( -7.505752307973343918, 22.59895833333332860, -28.01184896238290989 ) ) ;
#26717=CARTESIAN_POINT ( 'NONE',  ( 26.02091320914876960, 32.76263916574268364, 14.97647472619900455 ) ) ;
#26719=CARTESIAN_POINT ( 'NONE',  ( -20.50609665441004736, 46.37500000000000000, -20.50609665440969565 ) ) ;
#26722=CARTESIAN_POINT ( 'NONE',  ( 26.06988505166722803, 59.83295166574269075, -7.025853678916862854 ) ) ;
#26730=CARTESIAN_POINT ( 'NONE',  ( 26.07999730980477437, 26.89583333333332860, -6.988114217768290004 ) ) ;
#26738=CARTESIAN_POINT ( 'NONE',  ( -27.95245687107223986, 23.88243083240935505, 0.04044903255043252877 ) ) ;
#26741=CARTESIAN_POINT ( 'NONE',  ( 26.07999730980490227, 51.24479166666666430, 6.988114217767821046 ) ) ;
#26745=CARTESIAN_POINT ( 'NONE',  ( -15.01150461594642138, 12.14322916666666430, -26.00068869287340334 ) ) ;
#26746=CARTESIAN_POINT ( 'NONE',  ( -7.543491769121417612, 12.29204833425730925, 28.00173670424549499 ) ) ;
#26767=CARTESIAN_POINT ( 'NONE',  ( -0.04044903254992426173, 39.64881916759063074, 27.95245687107223276 ) ) ;
#26776=CARTESIAN_POINT ( 'NONE',  ( 7.468012846824281681, 52.38503499907601224, -28.02196122052058058 ) ) ;
#26779=CARTESIAN_POINT ( 'NONE',  ( -2.428612866367529427E-13, 26.17968750000000000, -27.95245687107222921 ) ) ;
#26781=CARTESIAN_POINT ( 'NONE',  ( 26.00068869287367335, 34.20052083333332860, 15.01150461594596308 ) ) ;
#26784=CARTESIAN_POINT ( 'NONE',  ( -25.98046417659859486, 40.79465250092398065, -15.04653450569291628 ) ) ;
#26786=CARTESIAN_POINT ( 'NONE',  ( -15.01150461594642138, 49.95572916666665009, -26.00068869287340334 ) ) ;
#26806=CARTESIAN_POINT ( 'NONE',  ( -6.988114217767819270, 65.85416666666665719, 26.07999730980490583 ) ) ;
#26811=CARTESIAN_POINT ( 'NONE',  ( -13.97622843553632777, 49.95572916666665009, -24.20753774853731599 ) ) ;
#26812=CARTESIAN_POINT ( 'NONE',  ( -25.98046417659859486, 30.48215250092397710, -15.04653450569291628 ) ) ;
#26813=CARTESIAN_POINT ( 'NONE',  ( -0.04044903255044120238, 24.74180583240935505, -30.02300923189239867 ) ) ;
#26817=CARTESIAN_POINT ( 'NONE',  ( 14.01125832528330051, 43.36159749907602645, 24.18731323226221974 ) ) ;
#26823=CARTESIAN_POINT ( 'NONE',  ( -13.94119854578936923, 51.39361083425730925, -24.22776226481241224 ) ) ;
#26827=CARTESIAN_POINT ( 'NONE',  ( -28.01184896238290278, 25.17708333333332860, 7.505752307973363457 ) ) ;
#26831=CARTESIAN_POINT ( 'NONE',  ( 15.01150461594596308, 57.40364583333333570, -26.00068869287367335 ) ) ;
#26837=CARTESIAN_POINT ( 'NONE',  ( -26.02091320914878025, 68.85638916574269786, -14.97647472619899389 ) ) ;
#26844=CARTESIAN_POINT ( 'NONE',  ( 13.97622843553633665, 34.48697916666667140, 24.20753774853730889 ) ) ;
#26850=CARTESIAN_POINT ( 'NONE',  ( -27.95245687107223986, 61.13319416759063785, -0.04044903254993292840 ) ) ;
#26864=CARTESIAN_POINT ( 'NONE',  ( -26.06988505166735237, 20.02642333425731280, -7.025853678916388567 ) ) ;
#26869=CARTESIAN_POINT ( 'NONE',  ( -20.50609665440969209, 48.95312500000000000, 20.50609665441005092 ) ) ;
#26873=CARTESIAN_POINT ( 'NONE',  ( 28.01184896238290278, 20.02083333333332860, -7.505752307973347470 ) ) ;
#26879=CARTESIAN_POINT ( 'NONE',  ( 28.02196122052058413, 32.61940999907601224, 7.468012846824272799 ) ) ;
#26881=CARTESIAN_POINT ( 'NONE',  ( -20.50609665440969209, 48.95312500000000000, 20.50609665441005092 ) ) ;
#26884=CARTESIAN_POINT ( 'NONE',  ( -0.04044903255042732459, 65.99180583240935505, -27.95245687107223986 ) ) ;
#26890=CARTESIAN_POINT ( 'NONE',  ( 26.07999730980490227, 23.74479166666666430, 6.988114217767821046 ) ) ;
#26896=CARTESIAN_POINT ( 'NONE',  ( -24.22776226481266448, 24.16888916574269075, -13.94119854578892514 ) ) ;
#26900=CARTESIAN_POINT ( 'NONE',  ( -24.20753774853756823, 56.54427083333332149, -13.97622843553588723 ) ) ;
#26904=CARTESIAN_POINT ( 'NONE',  ( 26.00068869287367335, 20.45052083333332504, 15.01150461594596308 ) ) ;
#26905=CARTESIAN_POINT ( 'NONE',  ( 15.04653450569292872, 21.02902750092397710, -25.98046417659857710 ) ) ;
#26925=CARTESIAN_POINT ( 'NONE',  ( -24.22776226481240514, 43.65923583425730925, 13.94119854578937812 ) ) ;
#26932=CARTESIAN_POINT ( 'NONE',  ( -28.00173670424535644, 58.11420166574269075, 7.543491769121936308 ) ) ;
#26936=CARTESIAN_POINT ( 'NONE',  ( -2.428612866367529427E-13, 22.74218749999999645, -27.95245687107222921 ) ) ;
#26939=CARTESIAN_POINT ( 'NONE',  ( 15.01150461594596308, 26.46614583333332149, -26.00068869287367335 ) ) ;
#26942=CARTESIAN_POINT ( 'NONE',  ( 14.97647472619947351, 49.67486083425730925, 26.02091320914850314 ) ) ;
#26944=CARTESIAN_POINT ( 'NONE',  ( -30.02300923189239512, 49.38281249999997868, 2.654126918244515359E-13 ) ) ;
#26945=CARTESIAN_POINT ( 'NONE',  ( -20.50609665440969209, 66.14062500000000000, 20.50609665441005092 ) ) ;
#26963=CARTESIAN_POINT ( 'NONE',  ( -19.06425588902591173, 10.00038166759064140, -19.11951029504763611 ) ) ;
#26968=CARTESIAN_POINT ( 'NONE',  ( -13.97622843553588901, 48.80989583333332860, 24.20753774853756823 ) ) ;
#26969=CARTESIAN_POINT ( 'NONE',  ( 26.02091320914851025, 35.06548583425731636, -14.97647472619946463 ) ) ;
#26970=CARTESIAN_POINT ( 'NONE',  ( -0.04044903255044120238, 31.61680583240936215, -30.02300923189239867 ) ) ;
#26974=CARTESIAN_POINT ( 'NONE',  ( -26.06988505166722803, 54.67670166574269075, 7.025853678916877953 ) ) ;
#26981=CARTESIAN_POINT ( 'NONE',  ( 14.01125832528286352, 51.96652750092398065, -24.18731323226246843 ) ) ;
#26986=CARTESIAN_POINT ( 'NONE',  ( 15.01150461594643204, 20.73697916666666075, 26.00068869287340334 ) ) ;
#26991=CARTESIAN_POINT ( 'NONE',  ( 7.505752307973351023, 55.25520833333333570, 28.01184896238290278 ) ) ;
#26998=CARTESIAN_POINT ( 'NONE',  ( 24.22776226481265383, 15.57513916574268720, 13.94119854578893580 ) ) ;
#27005=CARTESIAN_POINT ( 'NONE',  ( 13.97622843553589966, 43.65364583333332860, -24.20753774853756113 ) ) ;
#27012=CARTESIAN_POINT ( 'NONE',  ( -24.18731323226248264, 64.85715250092397355, -14.01125832528284931 ) ) ;
#27014=CARTESIAN_POINT ( 'NONE',  ( 26.00068869287367335, 54.82552083333331439, 15.01150461594596308 ) ) ;
#27027=CARTESIAN_POINT ( 'NONE',  ( -26.06988505166735237, 26.90142333425731280, -7.025853678916388567 ) ) ;
#27032=CARTESIAN_POINT ( 'NONE',  ( 15.01150461594643204, 51.67447916666665719, 26.00068869287340334 ) ) ;
#27036=CARTESIAN_POINT ( 'NONE',  ( -7.505752307972844761, 28.04166666666666075, 28.01184896238304134 ) ) ;
#27043=CARTESIAN_POINT ( 'NONE',  ( 7.543491769121922985, 43.50482666574268364, 28.00173670424535644 ) ) ;
#27045=CARTESIAN_POINT ( 'NONE',  ( 15.01150461594643382, 51.67447916666665719, 26.00068869287340334 ) ) ;
#27049=CARTESIAN_POINT ( 'NONE',  ( -6.988114217768288228, 12.28645833333333037, -26.07999730980477437 ) ) ;
#27055=CARTESIAN_POINT ( 'NONE',  ( -26.07999730980477437, 21.73958333333332860, 6.988114217768305103 ) ) ;
#27062=CARTESIAN_POINT ( 'NONE',  ( -26.09010956794245217, 27.46315999907601935, -6.950374756619243755 ) ) ;
#27067=CARTESIAN_POINT ( 'NONE',  ( 6.988114217768294445, 51.81770833333332860, 26.07999730980477437 ) ) ;
#27072=CARTESIAN_POINT ( 'NONE',  ( 28.01184896238304134, 20.30729166666666430, 7.505752307972846538 ) ) ;
#27073=CARTESIAN_POINT ( 'NONE',  ( -15.04653450569291984, 26.18527750092397710, 25.98046417659859486 ) ) ;
#27083=CARTESIAN_POINT ( 'NONE',  ( 28.02196122052045268, 52.39621500092398065, -7.468012846824774620 ) ) ;
#27089=CARTESIAN_POINT ( 'NONE',  ( -26.06988505166722803, 37.48920166574269075, 7.025853678916877953 ) ) ;
#27095=CARTESIAN_POINT ( 'NONE',  ( 24.22776226481241224, 38.50298583425730925, -13.94119854578936923 ) ) ;
#27103=CARTESIAN_POINT ( 'NONE',  ( -0.04044903255044120238, 55.67930583240935505, -30.02300923189239867 ) ) ;
#27107=CARTESIAN_POINT ( 'NONE',  ( -6.988114217768288228, 22.59895833333332860, -26.07999730980477437 ) ) ;
#27110=CARTESIAN_POINT ( 'NONE',  ( 7.505752307973351023, 27.75520833333332860, 28.01184896238290278 ) ) ;
#27111=( GEOMETRIC_REPRESENTATION_CONTEXT ( 3 ) GLOBAL_UNCERTAINTY_ASSIGNED_CONTEXT ( ( #10988 ) ) GLOBAL_UNIT_ASSIGNED_CONTEXT ( ( #15818, #32081, #16652 ) ) REPRESENTATION_CONTEXT ( 'NONE', 'WORKASPACE' ) );
#27115=CARTESIAN_POINT ( 'NONE',  ( -7.543491769121417612, 53.54204833425730925, 28.00173670424549499 ) ) ;
#27117=CARTESIAN_POINT ( 'NONE',  ( 7.505752307973351023, 62.13020833333334281, 28.01184896238290278 ) ) ;
#27136=CARTESIAN_POINT ( 'NONE',  ( 13.94119854578937812, 15.29986083425731280, 24.22776226481240514 ) ) ;
#27141=CARTESIAN_POINT ( 'NONE',  ( -19.09188309203694445, 46.37500000000000000, -19.09188309203661049 ) ) ;
#27142=CARTESIAN_POINT ( 'NONE',  ( -0.04044903254990864921, 39.64881916759063074, 30.02300923189239867 ) ) ;
#27143=CARTESIAN_POINT ( 'NONE',  ( -20.53372385742107653, 24.31211833240934794, -20.47846945139867003 ) ) ;
#27147=CARTESIAN_POINT ( 'NONE',  ( 27.95245687107223276, 59.97618083240934794, -0.04044903255042905932 ) ) ;
#27153=CARTESIAN_POINT ( 'NONE',  ( 19.11951029504763611, 48.67225666759065206, -19.06425588902591173 ) ) ;
#27157=CARTESIAN_POINT ( 'NONE',  ( 7.505752307973351023, 38.06770833333332860, 28.01184896238290278 ) ) ;
#27161=CARTESIAN_POINT ( 'NONE',  ( -20.50609665441004736, 60.12500000000000000, -20.50609665440969565 ) ) ;
#27168=CARTESIAN_POINT ( 'NONE',  ( 0.04044903255044120238, 19.58555583240935860, 27.95245687107223276 ) ) ;
#27177=CARTESIAN_POINT ( 'NONE',  ( -27.95245687107222921, 42.50781249999997868, 2.498001805406602216E-13 ) ) ;
#27183=CARTESIAN_POINT ( 'NONE',  ( 14.01125832528286352, 62.27902750092396644, -24.18731323226246843 ) ) ;
#27185=CARTESIAN_POINT ( 'NONE',  ( 20.50609665441005092, 58.40625000000000711, 20.50609665440969209 ) ) ;
#27198=CARTESIAN_POINT ( 'NONE',  ( -13.94119854578936923, 27.33111083425731280, -24.22776226481241224 ) ) ;
#27203=CARTESIAN_POINT ( 'NONE',  ( 15.01150461594643204, 55.11197916666664298, 26.00068869287340334 ) ) ;
#27207=CARTESIAN_POINT ( 'NONE',  ( 7.505752307973351023, 31.19270833333333215, 28.01184896238290278 ) ) ;
#27213=CARTESIAN_POINT ( 'NONE',  ( 7.468012846824281681, 42.07253499907601935, -28.02196122052058058 ) ) ;
#27215=CARTESIAN_POINT ( 'NONE',  ( -26.00068869287368756, 49.66927083333332149, -15.01150461594595775 ) ) ;
#27218=CARTESIAN_POINT ( 'NONE',  ( 24.20753774853731244, 16.44010416666666430, -13.97622843553632599 ) ) ;
#27223=CARTESIAN_POINT ( 'NONE',  ( 19.09188309203694800, 34.34374999999999289, 19.09188309203660694 ) ) ;
#27230=CARTESIAN_POINT ( 'NONE',  ( 25.98046417659831775, 25.31472249907601579, -15.04653450569338879 ) ) ;
#27233=CARTESIAN_POINT ( 'NONE',  ( 19.11951029504797006, 29.46836833240935505, 19.06425588902558133 ) ) ;
#27237=CARTESIAN_POINT ( 'NONE',  ( -13.97622843553632421, 56.83072916666665009, -24.20753774853731599 ) ) ;
#27242=CARTESIAN_POINT ( 'NONE',  ( 30.02300923189239512, 27.03906250000000000, -2.619432448724977703E-13 ) ) ;
#27243=CARTESIAN_POINT ( 'NONE',  ( -25.98046417659859486, 23.60715250092398421, -15.04653450569291628 ) ) ;
#27252=CARTESIAN_POINT ( 'NONE',  ( 20.47846945139902530, 52.96913166759063785, 20.53372385742071771 ) ) ;
#27254=CARTESIAN_POINT ( 'NONE',  ( 7.505752307973351023, 24.31770833333332504, 28.01184896238290278 ) ) ;
#27259=CARTESIAN_POINT ( 'NONE',  ( 7.025853678916867295, 46.94232666574269075, 26.06988505166722803 ) ) ;
#27265=CARTESIAN_POINT ( 'NONE',  ( 7.025853678916403666, 41.51079833425730214, -26.06988505166735237 ) ) ;
#27272=CARTESIAN_POINT ( 'NONE',  ( 14.97647472619900455, 59.40326416574269075, -26.02091320914876960 ) ) ;
#27276=CARTESIAN_POINT ( 'NONE',  ( 2.584737979205441561E-13, 24.46093749999999645, 27.95245687107222921 ) ) ;
#27279=CARTESIAN_POINT ( 'NONE',  ( -7.505752307973343918, 29.47395833333332860, -28.01184896238290989 ) ) ;
#27283=CARTESIAN_POINT ( 'NONE',  ( -20.47846945139902175, 51.25038166759065206, -20.53372385742072481 ) ) ;
#27285=CARTESIAN_POINT ( 'NONE',  ( -28.01184896238290278, 59.55208333333332149, 7.505752307973363457 ) ) ;
#27306=CARTESIAN_POINT ( 'NONE',  ( -26.07999730980477437, 66.42708333333332860, 6.988114217768305103 ) ) ;
#27311=CARTESIAN_POINT ( 'NONE',  ( -6.988114217768288228, 50.09895833333332860, -26.07999730980477437 ) ) ;
#27313=CARTESIAN_POINT ( 'NONE',  ( 28.00173670424549499, 35.49517333425730214, 7.543491769121417612 ) ) ;
#27314=CARTESIAN_POINT ( 'NONE',  ( -0.04044903255044120238, 28.17930583240935860, -30.02300923189239867 ) ) ;
#27318=CARTESIAN_POINT ( 'NONE',  ( 19.06425588902558133, 52.67149333240935505, -19.11951029504797006 ) ) ;
#27328=CARTESIAN_POINT ( 'NONE',  ( 2.740863092043355209E-13, 38.21093750000000000, 30.02300923189239512 ) ) ;
#27333=CARTESIAN_POINT ( 'NONE',  ( -7.505752307972844761, 58.97916666666666430, 28.01184896238304134 ) ) ;
#27341=CARTESIAN_POINT ( 'NONE',  ( 7.543491769121922985, 67.56732666574268364, 28.00173670424535644 ) ) ;
#27349=CARTESIAN_POINT ( 'NONE',  ( -13.97622843553632421, 39.64322916666667140, -24.20753774853731599 ) ) ;
#27355=CARTESIAN_POINT ( 'NONE',  ( 27.95245687107223986, 62.85194416759064495, 0.04044903254993640479 ) ) ;
#27356=CARTESIAN_POINT ( 'NONE',  ( 20.50609665440969565, 50.67187500000000000, -20.50609665441004736 ) ) ;
#27367=CARTESIAN_POINT ( 'NONE',  ( 24.22776226481241224, 35.06548583425731636, -13.94119854578936923 ) ) ;
#27372=CARTESIAN_POINT ( 'NONE',  ( -26.00068869287340334, 52.53385416666666430, 15.01150461594643382 ) ) ;
#27375=CARTESIAN_POINT ( 'NONE',  ( 15.01150461594596308, 26.46614583333332149, -26.00068869287367335 ) ) ;
#27380=CARTESIAN_POINT ( 'NONE',  ( 26.02091320914876960, 43.07513916574269786, 14.97647472619900455 ) ) ;
#27382=CARTESIAN_POINT ( 'NONE',  ( 15.01150461594643382, 55.11197916666665719, 26.00068869287340334 ) ) ;
#27386=CARTESIAN_POINT ( 'NONE',  ( -13.94119854578892514, 67.99701416574269786, 24.22776226481266448 ) ) ;
#27392=CARTESIAN_POINT ( 'NONE',  ( 26.07999730980477437, 33.77083333333333570, -6.988114217768290004 ) ) ;
#27397=CARTESIAN_POINT ( 'NONE',  ( -15.04653450569338524, 27.89284749907601935, -25.98046417659831775 ) ) ;
#27399=CARTESIAN_POINT ( 'NONE',  ( -26.06988505166722803, 40.92670166574268364, 7.025853678916877953 ) ) ;
#27404=CARTESIAN_POINT ( 'NONE',  ( 13.97622843553589966, 57.40364583333333570, -24.20753774853756113 ) ) ;
#27410=CARTESIAN_POINT ( 'NONE',  ( -26.00068869287340334, 28.47135416666666075, 15.01150461594643382 ) ) ;
#27411=CARTESIAN_POINT ( 'NONE',  ( 0.04044903254992426173, 20.74256916759064495, -30.02300923189239867 ) ) ;
#27419=CARTESIAN_POINT ( 'NONE',  ( 0.04044903254992426173, 58.55506916759063785, -30.02300923189239867 ) ) ;
#27422=CARTESIAN_POINT ( 'NONE',  ( 28.01184896238304134, 34.05729166666666430, 7.505752307972846538 ) ) ;
#27426=CARTESIAN_POINT ( 'NONE',  ( -27.95245687107223986, 47.94493083240935505, 0.04044903255043252877 ) ) ;
#27432=CARTESIAN_POINT ( 'NONE',  ( -24.18731323226248264, 40.79465250092398065, -14.01125832528284931 ) ) ;
#27439=CARTESIAN_POINT ( 'NONE',  ( -20.47846945139866648, 54.39024333240934794, 20.53372385742108008 ) ) ;
#27443=CARTESIAN_POINT ( 'NONE',  ( 19.09188309203661049, 30.04687500000000000, -19.09188309203694445 ) ) ;
#27446=CARTESIAN_POINT ( 'NONE',  ( -26.00068869287368756, 29.04427083333332504, -15.01150461594595775 ) ) ;
#27450=CARTESIAN_POINT ( 'NONE',  ( -30.02300923189239867, 54.25819416759065206, -0.04044903254991731589 ) ) ;
#27452=CARTESIAN_POINT ( 'NONE',  ( -26.00068869287368756, 63.41927083333333570, -15.01150461594595775 ) ) ;
#27460=DIRECTION ( 'NONE',  ( 0.000000000000000000, 0.000000000000000000, 1.000000000000000000 ) ) ;
#27474=CARTESIAN_POINT ( 'NONE',  ( 27.95245687107223986, 14.72694416759064318, 0.04044903254993640479 ) ) ;
#27479=CARTESIAN_POINT ( 'NONE',  ( 26.07999730980490227, 51.24479166666666430, 6.988114217767821046 ) ) ;
#27480=CARTESIAN_POINT ( 'NONE',  ( 25.98046417659858420, 35.63840250092398065, 15.04653450569292872 ) ) ;
#27481=CARTESIAN_POINT ( 'NONE',  ( -7.468012846824272799, 26.60378499907601579, 28.02196122052058413 ) ) ;
#27484=CARTESIAN_POINT ( 'NONE',  ( -27.95245687107223986, 58.25743083240935505, 0.04044903255043252877 ) ) ;
#27493=CARTESIAN_POINT ( 'NONE',  ( -20.50609665441004736, 36.06250000000000000, -20.50609665440969565 ) ) ;
#27498=CARTESIAN_POINT ( 'NONE',  ( 26.00068869287340334, 54.25260416666666430, -15.01150461594642316 ) ) ;
#27506=CARTESIAN_POINT ( 'NONE',  ( 24.18731323226221974, 15.00222249907602112, -14.01125832528328985 ) ) ;
#27515=CARTESIAN_POINT ( 'NONE',  ( 24.20753774853756113, 44.51302083333331439, 13.97622843553589789 ) ) ;
#27521=CARTESIAN_POINT ( 'NONE',  ( 20.47846945139902530, 11.71913166759064318, 20.53372385742071771 ) ) ;
#27522=CARTESIAN_POINT ( 'NONE',  ( 20.50609665440969565, 54.10937499999999289, -20.50609665441004736 ) ) ;
#27532=CARTESIAN_POINT ( 'NONE',  ( -26.09010956794232428, 30.05246500092397000, 6.950374756619732253 ) ) ;
#27538=CARTESIAN_POINT ( 'NONE',  ( 7.505752307973351023, 62.13020833333334281, 28.01184896238290278 ) ) ;
#27542=CARTESIAN_POINT ( 'NONE',  ( -28.01184896238304134, 28.90104166666666785, -7.505752307972844761 ) ) ;
#27547=CARTESIAN_POINT ( 'NONE',  ( 28.02196122052058413, 46.36940999907602645, 7.468012846824272799 ) ) ;
#27549=CARTESIAN_POINT ( 'NONE',  ( 20.50609665440969565, 60.98437499999999289, -20.50609665441004736 ) ) ;
#27553=CARTESIAN_POINT ( 'NONE',  ( -24.20753774853730889, 14.72135416666666607, 13.97622843553633842 ) ) ;
#27560=CARTESIAN_POINT ( 'NONE',  ( 19.09188309203661049, 33.48437500000000000, -19.09188309203694445 ) ) ;
#27565=CARTESIAN_POINT ( 'NONE',  ( -30.02300923189239867, 27.31993083240935505, 0.04044903255044988294 ) ) ;
#27567=CARTESIAN_POINT ( 'NONE',  ( -26.06988505166722803, 37.48920166574269075, 7.025853678916877953 ) ) ;
#27571=CARTESIAN_POINT ( 'NONE',  ( 13.97622843553589966, 60.84114583333332860, -24.20753774853756113 ) ) ;
#27576=CARTESIAN_POINT ( 'NONE',  ( 28.01184896238290278, 37.20833333333332860, -7.505752307973347470 ) ) ;
#27577=CARTESIAN_POINT ( 'NONE',  ( -20.47846945139902175, 34.06288166759063785, -20.53372385742072481 ) ) ;
#27586=CARTESIAN_POINT ( 'NONE',  ( -0.04044903254990864921, 56.83631916759064495, 30.02300923189239867 ) ) ;
#27589=CARTESIAN_POINT ( 'NONE',  ( 26.00068869287341045, 33.62760416666666430, -15.01150461594642493 ) ) ;
#27593=CARTESIAN_POINT ( 'NONE',  ( -6.950374756619247307, 40.35378499907601935, 26.09010956794245217 ) ) ;
#27599=CARTESIAN_POINT ( 'NONE',  ( -13.94119854578936923, 51.39361083425730925, -24.22776226481241224 ) ) ;
#27610=CARTESIAN_POINT ( 'NONE',  ( 0.04044903255045854962, 67.71055583240935505, 30.02300923189239867 ) ) ;
#27615=CARTESIAN_POINT ( 'NONE',  ( 19.09188309203661049, 36.92187499999999289, -19.09188309203694445 ) ) ;
#27619=CARTESIAN_POINT ( 'NONE',  ( 20.50609665441005092, 37.78124999999999289, 20.50609665440969209 ) ) ;
#27622=CARTESIAN_POINT ( 'NONE',  ( 15.04653450569292872, 48.52902750092398065, -25.98046417659857710 ) ) ;
#27624=CARTESIAN_POINT ( 'NONE',  ( 15.01150461594643204, 65.42447916666667140, 26.00068869287340334 ) ) ;
#27644=CARTESIAN_POINT ( 'NONE',  ( 26.09010956794232428, 21.45871500092397355, -6.950374756619718042 ) ) ;
#27649=CARTESIAN_POINT ( 'NONE',  ( -26.07999730980477437, 56.11458333333332860, 6.988114217768305103 ) ) ;
#27650=CARTESIAN_POINT ( 'NONE',  ( -7.468012846824771955, 41.22434000092397355, -28.02196122052045624 ) ) ;
#27651=CARTESIAN_POINT ( 'NONE',  ( -28.02196122052058413, 34.33815999907601224, -7.468012846824272799 ) ) ;
#27654=CARTESIAN_POINT ( 'NONE',  ( -7.025853678916861966, 52.09857666574269075, -26.06988505166722803 ) ) ;
#27656=CARTESIAN_POINT ( 'NONE',  ( -7.505752307973343918, 12.28645833333333037, -28.01184896238290989 ) ) ;
#27663=CARTESIAN_POINT ( 'NONE',  ( 2.740863092043355209E-13, 34.77343750000000000, 30.02300923189239512 ) ) ;
#27668=CARTESIAN_POINT ( 'NONE',  ( -20.50609665440969209, 66.14062500000000000, 20.50609665441005092 ) ) ;
#27677=CARTESIAN_POINT ( 'NONE',  ( -26.06988505166722803, 23.73920166574268364, 7.025853678916877953 ) ) ;
#27685=CARTESIAN_POINT ( 'NONE',  ( -19.09188309203660694, 45.51562500000000000, 19.09188309203694800 ) ) ;
#27690=CARTESIAN_POINT ( 'NONE',  ( 7.468012846824777284, 15.44309000092397355, 28.02196122052045268 ) ) ;
#27691=CARTESIAN_POINT ( 'NONE',  ( 7.505752307972854531, 53.82291666666666430, -28.01184896238303423 ) ) ;
#27702=CARTESIAN_POINT ( 'NONE',  ( -6.950374756619716266, 30.91184000092396644, -26.09010956794232428 ) ) ;
#27708=CARTESIAN_POINT ( 'NONE',  ( -7.505752307972844761, 62.41666666666666430, 28.01184896238304134 ) ) ;
#27712=CARTESIAN_POINT ( 'NONE',  ( -7.505752307973343918, 32.91145833333332860, -28.01184896238290989 ) ) ;
#27718=CARTESIAN_POINT ( 'NONE',  ( 28.02196122052058413, 53.24440999907603356, 7.468012846824272799 ) ) ;
#27720=CARTESIAN_POINT ( 'NONE',  ( 28.01184896238290278, 54.39583333333332860, -7.505752307973347470 ) ) ;
#27725=CARTESIAN_POINT ( 'NONE',  ( -26.07999730980477437, 14.86458333333333037, 6.988114217768305103 ) ) ;
#27736=CARTESIAN_POINT ( 'NONE',  ( -30.02300923189239867, 23.88243083240935505, 0.04044903255044988294 ) ) ;
#27737=CARTESIAN_POINT ( 'NONE',  ( -26.09010956794245217, 34.33815999907601224, -6.950374756619243755 ) ) ;
#27740=CARTESIAN_POINT ( 'NONE',  ( 6.988114217767829928, 64.13541666666667140, -26.07999730980489872 ) ) ;
#27746=ORIENTED_EDGE ( 'NONE', *, *, #6975, .T. ) ;
#27747=CARTESIAN_POINT ( 'NONE',  ( 7.505752307972854531, 33.19791666666665719, -28.01184896238303423 ) ) ;
#27748=CARTESIAN_POINT ( 'NONE',  ( -0.04044903254990864921, 32.77381916759064495, 30.02300923189239867 ) ) ;
#27757=CARTESIAN_POINT ( 'NONE',  ( -20.53372385742071771, 53.82850666759064495, 20.47846945139902530 ) ) ;
#27760=CARTESIAN_POINT ( 'NONE',  ( 15.01150461594596486, 29.90364583333332860, -26.00068869287367690 ) ) ;
#27767=CARTESIAN_POINT ( 'NONE',  ( 7.025853678916867295, 40.06732666574268364, 26.06988505166722803 ) ) ;
#27773=CARTESIAN_POINT ( 'NONE',  ( 6.950374756619721595, 49.81809000092397355, 26.09010956794232428 ) ) ;
#27780=CARTESIAN_POINT ( 'NONE',  ( -7.468012846824272799, 60.97878499907603356, 28.02196122052058413 ) ) ;
#27785=CARTESIAN_POINT ( 'NONE',  ( 19.09188309203694800, 30.90624999999999645, 19.09188309203660694 ) ) ;
#27789=CARTESIAN_POINT ( 'NONE',  ( 30.02300923189239512, 44.22656249999997868, -2.619432448724977703E-13 ) ) ;
#27792=CARTESIAN_POINT ( 'NONE',  ( 20.47846945139902530, 59.84413166759065206, 20.53372385742071771 ) ) ;
#27793=CARTESIAN_POINT ( 'NONE',  ( 26.06988505166735592, 59.55767333425731636, 7.025853678916393896 ) ) ;
#27796=CARTESIAN_POINT ( 'NONE',  ( -20.50609665441004736, 60.12500000000000000, -20.50609665440969565 ) ) ;
#27815=CARTESIAN_POINT ( 'NONE',  ( 0.04044903254993986036, 24.18006916759064140, -27.95245687107223986 ) ) ;
#27821=CARTESIAN_POINT ( 'NONE',  ( -20.47846945139902175, 44.37538166759063785, -20.53372385742072481 ) ) ;
#27823=CARTESIAN_POINT ( 'NONE',  ( 7.468012846824281681, 38.63503499907601224, -28.02196122052058058 ) ) ;
#27826=CARTESIAN_POINT ( 'NONE',  ( -19.09188309203694445, 11.99999999999999645, -19.09188309203661049 ) ) ;
#27829=CARTESIAN_POINT ( 'NONE',  ( 26.00068869287340334, 13.00260416666666430, -15.01150461594642316 ) ) ;
#27836=CARTESIAN_POINT ( 'NONE',  ( 28.01184896238290278, 37.20833333333332860, -7.505752307973347470 ) ) ;
#27846=CARTESIAN_POINT ( 'NONE',  ( -26.00068869287368756, 15.29427083333332860, -15.01150461594595775 ) ) ;
#27852=CARTESIAN_POINT ( 'NONE',  ( 13.94119854578893580, 28.46576416574268720, -24.22776226481265383 ) ) ;
#27860=CARTESIAN_POINT ( 'NONE',  ( -13.97622843553632421, 46.51822916666666430, -24.20753774853731599 ) ) ;
#27865=CARTESIAN_POINT ( 'NONE',  ( -20.47846945139902175, 16.87538166759064140, -20.53372385742072481 ) ) ;
#27866=CARTESIAN_POINT ( 'NONE',  ( 28.01184896238290278, 61.27083333333332860, -7.505752307973347470 ) ) ;
#27877=CARTESIAN_POINT ( 'NONE',  ( -0.04044903254992426173, 29.33631916759064850, 27.95245687107223276 ) ) ;
#27882=CARTESIAN_POINT ( 'NONE',  ( -28.01184896238290278, 59.55208333333332149, 7.505752307973363457 ) ) ;
#27885=CARTESIAN_POINT ( 'NONE',  ( 28.01184896238304134, 40.93229166666666430, 7.505752307972846538 ) ) ;
#27890=CARTESIAN_POINT ( 'NONE',  ( -7.468012846824272799, 50.66628499907601935, 28.02196122052058413 ) ) ;
#27892=CARTESIAN_POINT ( 'NONE',  ( -26.00068869287368756, 59.98177083333332860, -15.01150461594595775 ) ) ;
#27897=CARTESIAN_POINT ( 'NONE',  ( -13.97622843553632421, 25.89322916666666430, -24.20753774853731599 ) ) ;
#27909=CARTESIAN_POINT ( 'NONE',  ( -0.04044903255044120238, 28.17930583240935860, -30.02300923189239867 ) ) ;
#27911=CARTESIAN_POINT ( 'NONE',  ( -19.06425588902558133, 40.64024333240936215, 19.11951029504797006 ) ) ;
#27915=CARTESIAN_POINT ( 'NONE',  ( 13.97622843553589966, 64.27864583333332860, -24.20753774853756113 ) ) ;
#27920=CARTESIAN_POINT ( 'NONE',  ( -20.50609665441004736, 32.62500000000000000, -20.50609665440969565 ) ) ;
#27921=CARTESIAN_POINT ( 'NONE',  ( -7.543491769121417612, 32.91704833425729504, 28.00173670424549499 ) ) ;
#27930=CARTESIAN_POINT ( 'NONE',  ( 15.04653450569292872, 62.27902750092396644, -25.98046417659857710 ) ) ;
#27933=CARTESIAN_POINT ( 'NONE',  ( 26.00068869287341045, 30.19010416666665719, -15.01150461594642493 ) ) ;
#27939=CARTESIAN_POINT ( 'NONE',  ( 24.22776226481265383, 46.51263916574269786, 13.94119854578893580 ) ) ;
#27946=CARTESIAN_POINT ( 'NONE',  ( -14.01125832528285109, 50.24777750092398065, 24.18731323226248264 ) ) ;
#27953=CARTESIAN_POINT ( 'NONE',  ( 7.468012846824281681, 62.69753499907601224, -28.02196122052058058 ) ) ;
#27957=CARTESIAN_POINT ( 'NONE',  ( -13.97622843553632421, 39.64322916666667140, -24.20753774853731599 ) ) ;
#27960=CARTESIAN_POINT ( 'NONE',  ( -28.01184896238290278, 38.92708333333333570, 7.505752307973363457 ) ) ;
#27963=CARTESIAN_POINT ( 'NONE',  ( 7.468012846824777284, 60.13059000092398065, 28.02196122052045268 ) ) ;
#27964=CARTESIAN_POINT ( 'NONE',  ( 27.95245687107223986, 59.41444416759064495, 0.04044903254993640479 ) ) ;
#27966=CARTESIAN_POINT ( 'NONE',  ( 28.02196122052058413, 18.86940999907601935, 7.468012846824272799 ) ) ;
#27985=CARTESIAN_POINT ( 'NONE',  ( 24.18731323226247554, 21.88840250092397710, 14.01125832528285997 ) ) ;
#27990=CARTESIAN_POINT ( 'NONE',  ( 26.02091320914851025, 45.37798583425732346, -14.97647472619946463 ) ) ;
#27992=CARTESIAN_POINT ( 'NONE',  ( 28.02196122052058413, 36.05690999907600514, 7.468012846824272799 ) ) ;
#27995=CARTESIAN_POINT ( 'NONE',  ( -24.18731323226221974, 68.28347249907602645, 14.01125832528330406 ) ) ;
#27998=CARTESIAN_POINT ( 'NONE',  ( -26.00068869287368756, 15.29427083333332504, -15.01150461594595775 ) ) ;
#28005=CARTESIAN_POINT ( 'NONE',  ( 28.01184896238290278, 47.52083333333332860, -7.505752307973347470 ) ) ;
#28017=CARTESIAN_POINT ( 'NONE',  ( 24.22776226481265383, 29.32513916574269075, 13.94119854578893580 ) ) ;
#28026=CARTESIAN_POINT ( 'NONE',  ( 13.97622843553633665, 55.11197916666664298, 24.20753774853730889 ) ) ;
#28031=CARTESIAN_POINT ( 'NONE',  ( -26.02091320914849959, 23.03423583425731280, 14.97647472619947528 ) ) ;
#28033=CARTESIAN_POINT ( 'NONE',  ( -28.01184896238290278, 62.98958333333332149, 7.505752307973363457 ) ) ;
#28046=CARTESIAN_POINT ( 'NONE',  ( -24.18731323226248264, 37.35715250092397355, -14.01125832528284931 ) ) ;
#28053=CARTESIAN_POINT ( 'NONE',  ( 7.505752307972854531, 43.51041666666666430, -28.01184896238303423 ) ) ;
#28058=CARTESIAN_POINT ( 'NONE',  ( -30.02300923189239867, 51.38243083240936215, 0.04044903255044988294 ) ) ;
#28060=CARTESIAN_POINT ( 'NONE',  ( -15.01150461594642316, 60.26822916666665719, -26.00068869287341045 ) ) ;
#28065=CARTESIAN_POINT ( 'NONE',  ( -27.95245687107222921, 21.88281249999999645, 2.498001805406602216E-13 ) ) ;
#28077=CARTESIAN_POINT ( 'NONE',  ( -27.95245687107223986, 37.63243083240935505, 0.04044903255043252877 ) ) ;
#28081=CARTESIAN_POINT ( 'NONE',  ( -2.428612866367529427E-13, 60.55468749999999289, -27.95245687107222921 ) ) ;
#28082=ORIENTED_EDGE ( 'NONE', *, *, #6975, .F. ) ;
#28087=CARTESIAN_POINT ( 'NONE',  ( -15.01150461594595775, 35.05989583333332860, 26.00068869287368756 ) ) ;
#28088=CARTESIAN_POINT ( 'NONE',  ( 20.47846945139902530, 35.78163166759063074, 20.53372385742071771 ) ) ;
#28099=CARTESIAN_POINT ( 'NONE',  ( 25.98046417659858420, 63.13840250092397355, 15.04653450569292872 ) ) ;
#28102=CARTESIAN_POINT ( 'NONE',  ( -26.00068869287368756, 29.04427083333332860, -15.01150461594595775 ) ) ;
#28107=CARTESIAN_POINT ( 'NONE',  ( 24.18731323226221974, 52.81472249907603356, -14.01125832528328985 ) ) ;
#28120=CARTESIAN_POINT ( 'NONE',  ( -28.02196122052058413, 65.27565999907601224, -7.468012846824272799 ) ) ;
#28124=CARTESIAN_POINT ( 'NONE',  ( 2.584737979205441561E-13, 31.33593749999999289, 27.95245687107222921 ) ) ;
#28128=CARTESIAN_POINT ( 'NONE',  ( 30.02300923189239512, 40.78906249999998579, -2.619432448724977703E-13 ) ) ;
#28132=CARTESIAN_POINT ( 'NONE',  ( -26.02091320914849959, 60.84673583425731636, 14.97647472619947528 ) ) ;
#28133=CARTESIAN_POINT ( 'NONE',  ( -26.06988505166735237, 57.83892333425730214, -7.025853678916388567 ) ) ;
#28136=CARTESIAN_POINT ( 'NONE',  ( -7.543491769121917656, 17.72357666574268720, -28.00173670424536354 ) ) ;
#28156=CARTESIAN_POINT ( 'NONE',  ( 7.025853678916403666, 20.88579833425730925, -26.06988505166735237 ) ) ;
#28161=CARTESIAN_POINT ( 'NONE',  ( 25.98046417659858420, 49.38840250092398776, 15.04653450569292872 ) ) ;
#28163=CARTESIAN_POINT ( 'NONE',  ( 7.543491769121922985, 36.62982666574267654, 28.00173670424535644 ) ) ;
#28167=CARTESIAN_POINT ( 'NONE',  ( -24.18731323226221974, 64.84597249907602645, 14.01125832528330406 ) ) ;
#28176=CARTESIAN_POINT ( 'NONE',  ( 26.00068869287340334, 40.50260416666666430, -15.01150461594642316 ) ) ;
#28184=CARTESIAN_POINT ( 'NONE',  ( 28.01184896238290278, 16.58333333333333215, -7.505752307973347470 ) ) ;
#28189=CARTESIAN_POINT ( 'NONE',  ( 6.950374756619257965, 21.44753499907601579, -26.09010956794244507 ) ) ;
#28198=CARTESIAN_POINT ( 'NONE',  ( -24.20753774853730889, 49.09635416666665719, 13.97622843553633842 ) ) ;
#28203=CARTESIAN_POINT ( 'NONE',  ( -13.97622843553632777, 29.33072916666665719, -24.20753774853731599 ) ) ;
#28204=CARTESIAN_POINT ( 'NONE',  ( -0.04044903254990864921, 19.02381916759064495, 30.02300923189239867 ) ) ;
#28205=CARTESIAN_POINT ( 'NONE',  ( -30.02300923189239512, 59.69531250000000711, 2.654126918244515359E-13 ) ) ;
#28211=ORIENTED_EDGE ( 'NONE', *, *, #33703, .T. ) ;
#28214=CARTESIAN_POINT ( 'NONE',  ( 7.025853678916403666, 44.94829833425730925, -26.06988505166735237 ) ) ;
#28218=CARTESIAN_POINT ( 'NONE',  ( -26.00068869287368756, 18.73177083333332149, -15.01150461594595775 ) ) ;
#28223=CARTESIAN_POINT ( 'NONE',  ( 20.50609665440969565, 43.79687500000000000, -20.50609665441004736 ) ) ;
#28229=CARTESIAN_POINT ( 'NONE',  ( -7.543491769121917656, 52.09857666574269075, -28.00173670424536354 ) ) ;
#28236=CARTESIAN_POINT ( 'NONE',  ( -26.07999730980490583, 25.46354166666666430, -6.988114217767815717 ) ) ;
#28250=CARTESIAN_POINT ( 'NONE',  ( -19.11951029504797006, 48.37461833240936215, -19.06425588902558133 ) ) ;
#28254=CARTESIAN_POINT ( 'NONE',  ( -19.09188309203660694, 62.70312500000000000, 19.09188309203694800 ) ) ;
#28258=CARTESIAN_POINT ( 'NONE',  ( 20.50609665441005092, 30.90624999999999645, 20.50609665440969209 ) ) ;
#28259=CARTESIAN_POINT ( 'NONE',  ( 14.97647472619947351, 35.92486083425730214, 26.02091320914850314 ) ) ;
#28270=CARTESIAN_POINT ( 'NONE',  ( -28.02196122052045268, 64.42746500092397355, 7.468012846824790607 ) ) ;
#28273=CARTESIAN_POINT ( 'NONE',  ( -7.505752307973343918, 36.34895833333333570, -28.01184896238290989 ) ) ;
#28277=CARTESIAN_POINT ( 'NONE',  ( -26.06988505166722803, 51.23920166574269786, 7.025853678916877953 ) ) ;
#28283=CARTESIAN_POINT ( 'NONE',  ( -24.20753774853730889, 14.72135416666666607, 13.97622843553634020 ) ) ;
#28290=CARTESIAN_POINT ( 'NONE',  ( -19.11951029504797006, 13.99961833240935327, -19.06425588902558133 ) ) ;
#28294=CARTESIAN_POINT ( 'NONE',  ( -6.988114217767819270, 34.91666666666666430, 26.07999730980490583 ) ) ;
#28298=CARTESIAN_POINT ( 'NONE',  ( -20.50609665441004736, 42.93750000000000000, -20.50609665440969565 ) ) ;
#28301=CARTESIAN_POINT ( 'NONE',  ( -14.97647472619946285, 54.83111083425730214, -26.02091320914851025 ) ) ;
#28302=CARTESIAN_POINT ( 'NONE',  ( 19.11951029504763611, 62.42225666759065206, -19.06425588902591173 ) ) ;
#28304=CARTESIAN_POINT ( 'NONE',  ( -28.01184896238290278, 66.42708333333332860, 7.505752307973363457 ) ) ;
#28323=CARTESIAN_POINT ( 'NONE',  ( -24.18731323226248264, 20.16965250092397355, -14.01125832528284931 ) ) ;
#28329=CARTESIAN_POINT ( 'NONE',  ( 15.04653450569292872, 48.52902750092398065, -25.98046417659857710 ) ) ;
#28333=CARTESIAN_POINT ( 'NONE',  ( 15.04653450569339945, 36.48659749907601935, 25.98046417659831775 ) ) ;
#28337=CARTESIAN_POINT ( 'NONE',  ( 26.06988505166722803, 63.27045166574269075, -7.025853678916862854 ) ) ;
#28341=CARTESIAN_POINT ( 'NONE',  ( 15.01150461594596308, 12.71614583333333037, -26.00068869287367335 ) ) ;
#28347=CARTESIAN_POINT ( 'NONE',  ( 7.505752307973351023, 44.94270833333332860, 28.01184896238290278 ) ) ;
#28362=CARTESIAN_POINT ( 'NONE',  ( -19.06425588902558133, 26.89024333240934439, 19.11951029504797006 ) ) ;
#28370=CARTESIAN_POINT ( 'NONE',  ( -13.97622843553588901, 48.80989583333332860, 24.20753774853756823 ) ) ;
#28374=CARTESIAN_POINT ( 'NONE',  ( 26.07999730980477437, 30.33333333333332860, -6.988114217768290004 ) ) ;
#28375=CARTESIAN_POINT ( 'NONE',  ( 20.53372385742072481, 17.73475666759064140, -20.47846945139902175 ) ) ;
#28376=CARTESIAN_POINT ( 'NONE',  ( 15.01150461594643204, 61.98697916666665009, 26.00068869287340334 ) ) ;
#28386=CARTESIAN_POINT ( 'NONE',  ( 19.06425588902592239, 39.21913166759063785, 19.11951029504763611 ) ) ;
#28394=CARTESIAN_POINT ( 'NONE',  ( 28.01184896238290278, 44.08333333333332860, -7.505752307973347470 ) ) ;
#28399=CARTESIAN_POINT ( 'NONE',  ( 20.47846945139867003, 56.10899333240935505, -20.53372385742107653 ) ) ;
#28401=CARTESIAN_POINT ( 'NONE',  ( -2.584737979205442066E-13, 63.99218749999997868, -30.02300923189239867 ) ) ;
#28406=CARTESIAN_POINT ( 'NONE',  ( -6.988114217768288228, 19.16145833333332860, -26.07999730980477437 ) ) ;
#28423=CARTESIAN_POINT ( 'NONE',  ( -7.025853678916393008, 15.72954833425730925, 26.06988505166735592 ) ) ;
#28427=CARTESIAN_POINT ( 'NONE',  ( 15.01150461594596308, 43.65364583333332860, -26.00068869287367335 ) ) ;
#28437=CARTESIAN_POINT ( 'NONE',  ( 26.00068869287340334, 16.44010416666666430, -15.01150461594642316 ) ) ;
#28439=CARTESIAN_POINT ( 'NONE',  ( 26.00068869287367690, 37.63802083333331439, 15.01150461594596486 ) ) ;
#28444=CARTESIAN_POINT ( 'NONE',  ( -24.22776226481266448, 51.66888916574269075, -13.94119854578892514 ) ) ;
#28449=CARTESIAN_POINT ( 'NONE',  ( -6.988114217768288228, 15.72395833333332860, -26.07999730980477437 ) ) ;
#28458=CARTESIAN_POINT ( 'NONE',  ( -26.06988505166722803, 20.30170166574269075, 7.025853678916877953 ) ) ;
#28462=CARTESIAN_POINT ( 'NONE',  ( -24.20753774853756823, 42.79427083333331439, -13.97622843553588723 ) ) ;
#28465=CARTESIAN_POINT ( 'NONE',  ( 26.00068869287340334, 47.37760416666666430, -15.01150461594642316 ) ) ;
#28467=CARTESIAN_POINT ( 'NONE',  ( 28.02196122052045268, 59.27121500092397355, -7.468012846824774620 ) ) ;
#28468=CARTESIAN_POINT ( 'NONE',  ( 0.04044903254993986036, 61.99256916759065206, -27.95245687107223986 ) ) ;
#28471=CARTESIAN_POINT ( 'NONE',  ( 15.04653450569339945, 19.29909749907602290, 25.98046417659831775 ) ) ;
#28488=CARTESIAN_POINT ( 'NONE',  ( 26.06988505166735592, 28.62017333425730925, 7.025853678916393896 ) ) ;
#28494=CARTESIAN_POINT ( 'NONE',  ( 28.02196122052058413, 42.93190999907601935, 7.468012846824272799 ) ) ;
#28498=CARTESIAN_POINT ( 'NONE',  ( -6.950374756619247307, 64.41628499907602645, 26.09010956794245217 ) ) ;
#28500=CARTESIAN_POINT ( 'NONE',  ( -20.50609665440969209, 21.45312499999999645, 20.50609665441005092 ) ) ;
#28506=CARTESIAN_POINT ( 'NONE',  ( 2.740863092043355209E-13, 41.64843750000000000, 30.02300923189239512 ) ) ;
#28507=CARTESIAN_POINT ( 'NONE',  ( 30.02300923189239512, 64.85156249999998579, -2.619432448724977703E-13 ) ) ;
#28524=CARTESIAN_POINT ( 'NONE',  ( -24.22776226481266448, 31.04388916574268364, -13.94119854578892514 ) ) ;
#28532=CARTESIAN_POINT ( 'NONE',  ( 13.97622843553633665, 51.67447916666665719, 24.20753774853730889 ) ) ;
#28536=CARTESIAN_POINT ( 'NONE',  ( -6.988114217768288228, 43.22395833333332860, -26.07999730980477437 ) ) ;
#28537=CARTESIAN_POINT ( 'NONE',  ( -20.53372385742071771, 22.89100666759064495, 20.47846945139902530 ) ) ;
#28538=CARTESIAN_POINT ( 'NONE',  ( -0.04044903255044120238, 14.42930583240935505, -30.02300923189239867 ) ) ;
#28548=CARTESIAN_POINT ( 'NONE',  ( -7.025853678916393008, 46.66704833425730925, 26.06988505166735592 ) ) ;
#28552=CARTESIAN_POINT ( 'NONE',  ( 7.505752307972854531, 12.57291666666666252, -28.01184896238303423 ) ) ;
#28557=CARTESIAN_POINT ( 'NONE',  ( 15.01150461594643204, 41.36197916666666430, 26.00068869287340334 ) ) ;
#28563=CARTESIAN_POINT ( 'NONE',  ( 20.53372385742108008, 60.40586833240935505, 20.47846945139866648 ) ) ;
#28567=CARTESIAN_POINT ( 'NONE',  ( -24.20753774853756823, 63.41927083333333570, -13.97622843553588723 ) ) ;
#28570=CARTESIAN_POINT ( 'NONE',  ( 6.988114217768294445, 24.31770833333332504, 26.07999730980477437 ) ) ;
#28577=CARTESIAN_POINT ( 'NONE',  ( 26.09010956794232428, 45.52121500092397355, -6.950374756619718042 ) ) ;
#28587=CARTESIAN_POINT ( 'NONE',  ( 19.11951029504763611, 10.85975666759064318, -19.06425588902591173 ) ) ;
#28591=CARTESIAN_POINT ( 'NONE',  ( -2.584737979205441561E-13, 39.92968750000000000, -30.02300923189239512 ) ) ;
#28601=CARTESIAN_POINT ( 'NONE',  ( -30.02300923189239867, 64.57069416759065916, -0.04044903254991731589 ) ) ;
#28603=CARTESIAN_POINT ( 'NONE',  ( 20.50609665440969565, 36.92187499999999289, -20.50609665441004736 ) ) ;
#28609=CARTESIAN_POINT ( 'NONE',  ( 6.950374756619257965, 52.38503499907601224, -26.09010956794244507 ) ) ;
#28615=CARTESIAN_POINT ( 'NONE',  ( 26.07999730980477437, 13.14583333333332860, -6.988114217768290004 ) ) ;
#28624=CARTESIAN_POINT ( 'NONE',  ( 13.94119854578893580, 14.71576416574268720, -24.22776226481265383 ) ) ;
#28628=CARTESIAN_POINT ( 'NONE',  ( 24.20753774853731244, 43.94010416666665719, -13.97622843553632599 ) ) ;
#28631=CARTESIAN_POINT ( 'NONE',  ( -26.00068869287340334, 45.65885416666666430, 15.01150461594643382 ) ) ;
#28633=CARTESIAN_POINT ( 'NONE',  ( 15.01150461594643204, 13.86197916666666430, 26.00068869287340334 ) ) ;
#28634=CARTESIAN_POINT ( 'NONE',  ( 0.04044903254992426173, 17.30506916759064140, -30.02300923189239867 ) ) ;
#28646=SURFACE_STYLE_FILL_AREA ( #10972 ) ;
#28659=CARTESIAN_POINT ( 'NONE',  ( -7.025853678916393008, 29.47954833425730570, 26.06988505166735592 ) ) ;
#28669=CARTESIAN_POINT ( 'NONE',  ( 20.47846945139867003, 42.35899333240935505, -20.53372385742107653 ) ) ;
#28672=CARTESIAN_POINT ( 'NONE',  ( -2.428612866367529427E-13, 19.30468749999999645, -27.95245687107222921 ) ) ;
#28675=CARTESIAN_POINT ( 'NONE',  ( 20.50609665440969565, 23.17187499999999289, -20.50609665441004736 ) ) ;
#28679=CARTESIAN_POINT ( 'NONE',  ( -26.02091320914849959, 43.65923583425730925, 14.97647472619947528 ) ) ;
#28681=CARTESIAN_POINT ( 'NONE',  ( -20.50609665440969209, 45.51562500000000000, 20.50609665441005092 ) ) ;
#28682=CARTESIAN_POINT ( 'NONE',  ( -28.01184896238290278, 62.98958333333332149, 7.505752307973363457 ) ) ;
#28692=CARTESIAN_POINT ( 'NONE',  ( 7.505752307972854531, 19.44791666666666075, -28.01184896238303423 ) ) ;
#28697=CARTESIAN_POINT ( 'NONE',  ( 24.22776226481265383, 36.20013916574269075, 13.94119854578893580 ) ) ;
#28704=CARTESIAN_POINT ( 'NONE',  ( 6.988114217768294445, 55.25520833333333570, 26.07999730980477437 ) ) ;
#28708=CARTESIAN_POINT ( 'NONE',  ( -2.428612866367529427E-13, 39.92968750000000000, -27.95245687107223276 ) ) ;
#28709=CARTESIAN_POINT ( 'NONE',  ( 28.00173670424549499, 28.62017333425730925, 7.543491769121417612 ) ) ;
#28710=CARTESIAN_POINT ( 'NONE',  ( 28.00173670424535644, 15.14545166574268897, -7.543491769121920321 ) ) ;
#28714=CIRCLE ( 'NONE', #25974, 0.9999999999999988898 ) ;
#28722=CARTESIAN_POINT ( 'NONE',  ( -0.04044903254992426173, 39.64881916759063074, 27.95245687107223276 ) ) ;
#28726=CARTESIAN_POINT ( 'NONE',  ( 28.01184896238304134, 16.86979166666666075, 7.505752307972846538 ) ) ;
#28730=CARTESIAN_POINT ( 'NONE',  ( -7.505752307972844761, 45.22916666666665719, 28.01184896238304134 ) ) ;
#28735=CARTESIAN_POINT ( 'NONE',  ( -15.04653450569338524, 58.83034749907602645, -25.98046417659831775 ) ) ;
#28740=CARTESIAN_POINT ( 'NONE',  ( -2.428612866367529427E-13, 60.55468749999998579, -27.95245687107223276 ) ) ;
#28743=CARTESIAN_POINT ( 'NONE',  ( -19.09188309203694445, 32.62500000000000000, -19.09188309203661049 ) ) ;
#28749=CARTESIAN_POINT ( 'NONE',  ( -19.06425588902591173, 51.25038166759065206, -19.11951029504763611 ) ) ;
#28762=CARTESIAN_POINT ( 'NONE',  ( -26.06988505166735237, 13.15142333425730925, -7.025853678916388567 ) ) ;
#28766=CARTESIAN_POINT ( 'NONE',  ( -20.50609665440969209, 45.51562500000000000, 20.50609665441005092 ) ) ;
#28770=CARTESIAN_POINT ( 'NONE',  ( -2.584737979205441561E-13, 19.30468749999999645, -30.02300923189239512 ) ) ;
#28776=CARTESIAN_POINT ( 'NONE',  ( -28.00173670424535644, 37.48920166574269075, 7.543491769121936308 ) ) ;
#28778=CARTESIAN_POINT ( 'NONE',  ( 7.505752307972854531, 43.51041666666666430, -28.01184896238303423 ) ) ;
#28783=CARTESIAN_POINT ( 'NONE',  ( 6.950374756619257965, 66.13503499907601224, -26.09010956794244507 ) ) ;
#28788=CARTESIAN_POINT ( 'NONE',  ( 13.97622843553633842, 13.86197916666666252, 24.20753774853730889 ) ) ;
#28796=CARTESIAN_POINT ( 'NONE',  ( -19.06425588902558133, 16.57774333240934794, 19.11951029504797006 ) ) ;
#28799=EDGE_CURVE ( 'NONE', #21772, #32341, #26021, .T. ) ;
#28802=CARTESIAN_POINT ( 'NONE',  ( -13.97622843553632421, 46.51822916666666430, -24.20753774853731599 ) ) ;
#28807=CARTESIAN_POINT ( 'NONE',  ( -26.00068869287368756, 18.73177083333332149, -15.01150461594595775 ) ) ;
#28808=CARTESIAN_POINT ( 'NONE',  ( 7.468012846824777284, 12.00559000092397532, 28.02196122052045268 ) ) ;
#28828=CARTESIAN_POINT ( 'NONE',  ( 24.22776226481241224, 28.19048583425731636, -13.94119854578936923 ) ) ;
#28835=CARTESIAN_POINT ( 'NONE',  ( -30.02300923189239867, 44.50743083240935505, 0.04044903255044988294 ) ) ;
#28839=CARTESIAN_POINT ( 'NONE',  ( -19.09188309203660694, 21.45312499999999645, 19.09188309203694800 ) ) ;
#28842=CARTESIAN_POINT ( 'NONE',  ( -15.01150461594595775, 24.74739583333332504, 26.00068869287368756 ) ) ;
#28846=CARTESIAN_POINT ( 'NONE',  ( -7.468012846824771955, 44.66184000092397355, -28.02196122052045624 ) ) ;
#28848=CARTESIAN_POINT ( 'NONE',  ( -15.01150461594595775, 48.80989583333332860, 26.00068869287368756 ) ) ;
#28860=CARTESIAN_POINT ( 'NONE',  ( 26.00068869287367690, 17.01302083333332504, 15.01150461594596486 ) ) ;
#28865=CARTESIAN_POINT ( 'NONE',  ( -0.04044903255042732459, 31.61680583240936215, -27.95245687107223986 ) ) ;
#28873=CARTESIAN_POINT ( 'NONE',  ( -27.95245687107222921, 63.13281250000000000, 2.498001805406602216E-13 ) ) ;
#28877=CARTESIAN_POINT ( 'NONE',  ( 26.07999730980477437, 40.64583333333332860, -6.988114217768290004 ) ) ;
#28878=CARTESIAN_POINT ( 'NONE',  ( 25.98046417659858420, 28.76340250092398065, 15.04653450569292872 ) ) ;
#28879=CARTESIAN_POINT ( 'NONE',  ( -28.00173670424535644, 16.86420166574268720, 7.543491769121936308 ) ) ;
#28883=CARTESIAN_POINT ( 'NONE',  ( 7.025853678916867295, 50.37982666574269075, 26.06988505166722803 ) ) ;
#28888=CARTESIAN_POINT ( 'NONE',  ( 26.06988505166735592, 42.37017333425730925, 7.025853678916393896 ) ) ;
#28895=CARTESIAN_POINT ( 'NONE',  ( 7.505752307973351023, 51.81770833333332860, 28.01184896238290278 ) ) ;
#28902=CARTESIAN_POINT ( 'NONE',  ( 7.468012846824281681, 66.13503499907601224, -28.02196122052058058 ) ) ;
#28906=CARTESIAN_POINT ( 'NONE',  ( 24.20753774853731244, 57.69010416666666430, -13.97622843553633132 ) ) ;
#28909=CARTESIAN_POINT ( 'NONE',  ( 6.988114217767829928, 33.19791666666665719, -26.07999730980489872 ) ) ;
#28915=CARTESIAN_POINT ( 'NONE',  ( 26.09010956794232428, 59.27121500092397355, -6.950374756619718042 ) ) ;
#28928=CARTESIAN_POINT ( 'NONE',  ( 13.94119854578937812, 18.73736083425731636, 24.22776226481240514 ) ) ;
#28933=CARTESIAN_POINT ( 'NONE',  ( -28.01184896238290278, 45.80208333333333570, 7.505752307973363457 ) ) ;
#28937=CARTESIAN_POINT ( 'NONE',  ( 26.00068869287367335, 23.88802083333331794, 15.01150461594596308 ) ) ;
#28944=CARTESIAN_POINT ( 'NONE',  ( 0.04044903255045854962, 36.77305583240936215, 30.02300923189239867 ) ) ;
#28946=CARTESIAN_POINT ( 'NONE',  ( 7.505752307972854531, 36.63541666666666430, -28.01184896238303423 ) ) ;
#28954=CARTESIAN_POINT ( 'NONE',  ( -6.950374756619247307, 60.97878499907603356, 26.09010956794245217 ) ) ;
#28967=CARTESIAN_POINT ( 'NONE',  ( -24.18731323226221974, 20.15847249907602290, 14.01125832528330406 ) ) ;
#28971=CARTESIAN_POINT ( 'NONE',  ( 26.07999730980477437, 47.52083333333332860, -6.988114217768290004 ) ) ;
#28975=CARTESIAN_POINT ( 'NONE',  ( 2.740863092043355209E-13, 14.14843749999999289, 30.02300923189239512 ) ) ;
#28976=CARTESIAN_POINT ( 'NONE',  ( 20.47846945139902530, 15.15663166759064495, 20.53372385742071771 ) ) ;
#28995=CARTESIAN_POINT ( 'NONE',  ( -14.01125832528285109, 26.18527750092397710, 24.18731323226248264 ) ) ;
#29002=CARTESIAN_POINT ( 'NONE',  ( -20.53372385742107653, 48.37461833240936215, -20.47846945139867003 ) ) ;
#29006=CARTESIAN_POINT ( 'NONE',  ( 19.09188309203661049, 12.85937500000000000, -19.09188309203694445 ) ) ;
#29009=CARTESIAN_POINT ( 'NONE',  ( 28.01184896238290278, 20.02083333333332860, -7.505752307973347470 ) ) ;
#29013=CARTESIAN_POINT ( 'NONE',  ( -15.04653450569291984, 43.37277750092397355, 25.98046417659859486 ) ) ;
#29015=CARTESIAN_POINT ( 'NONE',  ( 7.505752307973351023, 48.38020833333332860, 28.01184896238290278 ) ) ;
#29024=CARTESIAN_POINT ( 'NONE',  ( 26.00068869287367690, 20.45052083333332860, 15.01150461594596486 ) ) ;
#29029=CARTESIAN_POINT ( 'NONE',  ( 26.06988505166722803, 35.77045166574266943, -7.025853678916862854 ) ) ;
#29036=CARTESIAN_POINT ( 'NONE',  ( 19.09188309203661049, 60.98437499999999289, -19.09188309203694445 ) ) ;
#29040=CARTESIAN_POINT ( 'NONE',  ( -13.97622843553588901, 41.93489583333333570, 24.20753774853756823 ) ) ;
#29041=CARTESIAN_POINT ( 'NONE',  ( -7.468012846824771955, 27.47434000092397000, -28.02196122052045624 ) ) ;
#29042=CARTESIAN_POINT ( 'NONE',  ( 28.00173670424535644, 22.02045166574269075, -7.543491769121920321 ) ) ;
#29046=CARTESIAN_POINT ( 'NONE',  ( -13.94119854578892514, 47.37201416574269786, 24.22776226481266448 ) ) ;
#29052=CARTESIAN_POINT ( 'NONE',  ( 19.06425588902592239, 49.53163166759063785, 19.11951029504763611 ) ) ;
#29056=CARTESIAN_POINT ( 'NONE',  ( 26.00068869287367335, 27.32552083333332860, 15.01150461594596308 ) ) ;
#29060=CARTESIAN_POINT ( 'NONE',  ( 30.02300923189239512, 44.22656249999997868, -2.619432448724977703E-13 ) ) ;
#29066=CARTESIAN_POINT ( 'NONE',  ( -20.47846945139866648, 64.70274333240935505, 20.53372385742108008 ) ) ;
#29072=CARTESIAN_POINT ( 'NONE',  ( 6.988114217767829928, 60.69791666666667140, -26.07999730980489872 ) ) ;
#29075=CARTESIAN_POINT ( 'NONE',  ( 6.988114217767829928, 36.63541666666666430, -26.07999730980489872 ) ) ;
#29080=CARTESIAN_POINT ( 'NONE',  ( 24.22776226481241224, 55.69048583425730925, -13.94119854578936923 ) ) ;
#29092=CARTESIAN_POINT ( 'NONE',  ( 13.94119854578937812, 15.29986083425731280, 24.22776226481240514 ) ) ;
#29097=CARTESIAN_POINT ( 'NONE',  ( 28.01184896238304134, 40.93229166666666430, 7.505752307972846538 ) ) ;
#29101=CARTESIAN_POINT ( 'NONE',  ( -20.50609665440969209, 21.45312499999999645, 20.50609665441005092 ) ) ;
#29107=CARTESIAN_POINT ( 'NONE',  ( 20.47846945139867003, 32.04649333240934084, -20.53372385742107653 ) ) ;
#29110=CARTESIAN_POINT ( 'NONE',  ( -7.505752307972844761, 45.22916666666665719, 28.01184896238304134 ) ) ;
#29116=CARTESIAN_POINT ( 'NONE',  ( 13.94119854578893580, 66.27826416574268364, -24.22776226481265383 ) ) ;
#29123=CARTESIAN_POINT ( 'NONE',  ( 19.09188309203694800, 20.59374999999999645, 19.09188309203660694 ) ) ;
#29130=CARTESIAN_POINT ( 'NONE',  ( 13.94119854578893580, 21.59076416574269430, -24.22776226481265383 ) ) ;
#29134=CARTESIAN_POINT ( 'NONE',  ( -26.07999730980477437, 42.36458333333332860, 6.988114217768305103 ) ) ;
#29138=CARTESIAN_POINT ( 'NONE',  ( -25.98046417659859486, 64.85715250092397355, -15.04653450569291628 ) ) ;
#29139=CARTESIAN_POINT ( 'NONE',  ( 7.543491769121427382, 14.01079833425730747, -28.00173670424548433 ) ) ;
#29158=CARTESIAN_POINT ( 'NONE',  ( -19.06425588902591173, 30.62538166759064495, -19.11951029504763611 ) ) ;
#29166=CARTESIAN_POINT ( 'NONE',  ( -26.02091320914878025, 44.79388916574269075, -14.97647472619899389 ) ) ;
#29172=CARTESIAN_POINT ( 'NONE',  ( 24.20753774853756113, 20.45052083333332504, 13.97622843553589789 ) ) ;
#29176=CARTESIAN_POINT ( 'NONE',  ( -26.00068869287340334, 18.15885416666666075, 15.01150461594643382 ) ) ;
#29180=CARTESIAN_POINT ( 'NONE',  ( -26.02091320914849959, 40.22173583425730925, 14.97647472619947528 ) ) ;
#29182=CARTESIAN_POINT ( 'NONE',  ( -7.505752307973343918, 56.97395833333333570, -28.01184896238290989 ) ) ;
#29192=CARTESIAN_POINT ( 'NONE',  ( 2.740863092043355209E-13, 21.02343750000000000, 30.02300923189239867 ) ) ;
#29205=CARTESIAN_POINT ( 'NONE',  ( -2.428612866367529427E-13, 63.99218749999997868, -27.95245687107222921 ) ) ;
#29209=CARTESIAN_POINT ( 'NONE',  ( 24.20753774853731244, 40.50260416666666430, -13.97622843553633132 ) ) ;
#29210=CARTESIAN_POINT ( 'NONE',  ( -0.04044903254990864921, 25.89881916759064140, 30.02300923189239867 ) ) ;
#29211=CARTESIAN_POINT ( 'NONE',  ( -15.04653450569338524, 21.01784749907601579, -25.98046417659831775 ) ) ;
#29215=CARTESIAN_POINT ( 'NONE',  ( -6.950374756619247307, 43.79128499907601935, 26.09010956794245217 ) ) ;
#29221=CARTESIAN_POINT ( 'NONE',  ( -13.94119854578936923, 47.95611083425732346, -24.22776226481241224 ) ) ;
#29226=CARTESIAN_POINT ( 'NONE',  ( -15.01150461594642138, 29.33072916666665719, -26.00068869287340334 ) ) ;
#29230=CARTESIAN_POINT ( 'NONE',  ( -28.01184896238304134, 49.52604166666666430, -7.505752307972844761 ) ) ;
#29237=CARTESIAN_POINT ( 'NONE',  ( 26.02091320914876960, 63.70013916574268364, 14.97647472619900455 ) ) ;
#29241=CARTESIAN_POINT ( 'NONE',  ( -19.09188309203660694, 62.70312500000000000, 19.09188309203694800 ) ) ;
#29244=CARTESIAN_POINT ( 'NONE',  ( 26.07999730980477437, 30.33333333333332860, -6.988114217768290004 ) ) ;
#29249=CARTESIAN_POINT ( 'NONE',  ( -26.09010956794232428, 54.11496500092397355, 6.950374756619732253 ) ) ;
#29261=CARTESIAN_POINT ( 'NONE',  ( 6.950374756619721595, 22.31809000092397000, 26.09010956794232428 ) ) ;
#29267=CARTESIAN_POINT ( 'NONE',  ( -20.50609665441004736, 49.81249999999999289, -20.50609665440969565 ) ) ;
#29272=CARTESIAN_POINT ( 'NONE',  ( 30.02300923189239512, 16.72656249999999645, -2.619432448724977703E-13 ) ) ;
#29279=CARTESIAN_POINT ( 'NONE',  ( -7.543491769121917656, 38.34857666574267654, -28.00173670424536354 ) ) ;
#29281=CARTESIAN_POINT ( 'NONE',  ( 26.00068869287367690, 51.38802083333332860, 15.01150461594596486 ) ) ;
#29285=CARTESIAN_POINT ( 'NONE',  ( 24.22776226481265383, 60.26263916574269786, 13.94119854578893580 ) ) ;
#29292=CARTESIAN_POINT ( 'NONE',  ( 19.09188309203661049, 26.60937499999999645, -19.09188309203694445 ) ) ;
#29300=CARTESIAN_POINT ( 'NONE',  ( 19.06425588902558133, 32.04649333240934084, -19.11951029504797006 ) ) ;
#29303=CARTESIAN_POINT ( 'NONE',  ( -19.09188309203694445, 53.25000000000000000, -19.09188309203661049 ) ) ;
#29307=CARTESIAN_POINT ( 'NONE',  ( -28.01184896238290278, 18.30208333333332860, 7.505752307973363457 ) ) ;
#29308=CARTESIAN_POINT ( 'NONE',  ( 7.543491769121427382, 10.57329833425730747, -28.00173670424548433 ) ) ;
#29330=CARTESIAN_POINT ( 'NONE',  ( 6.950374756619721595, 36.06809000092397355, 26.09010956794232428 ) ) ;
#29338=CARTESIAN_POINT ( 'NONE',  ( 30.02300923189239867, 53.10118083240936215, -0.04044903255044467877 ) ) ;
#29343=CARTESIAN_POINT ( 'NONE',  ( -13.97622843553588901, 17.87239583333332149, 24.20753774853756823 ) ) ;
#29345=CARTESIAN_POINT ( 'NONE',  ( 28.01184896238290278, 33.77083333333333570, -7.505752307973347470 ) ) ;
#29348=CARTESIAN_POINT ( 'NONE',  ( 28.00173670424549499, 38.93267333425729504, 7.543491769121417612 ) ) ;
#29351=CARTESIAN_POINT ( 'NONE',  ( -2.584737979205441561E-13, 50.24218750000000711, -30.02300923189239512 ) ) ;
#29373=CARTESIAN_POINT ( 'NONE',  ( 26.09010956794232428, 11.14621500092397532, -6.950374756619718042 ) ) ;
#29379=CARTESIAN_POINT ( 'NONE',  ( -27.95245687107223276, 52.82031249999998579, 2.498001805406602216E-13 ) ) ;
#29380=CARTESIAN_POINT ( 'NONE',  ( -28.00173670424549499, 33.77642333425730214, -7.543491769121417612 ) ) ;
#29381=CARTESIAN_POINT ( 'NONE',  ( -20.47846945139866648, 30.32774333240935150, 20.53372385742108008 ) ) ;
#29385=CARTESIAN_POINT ( 'NONE',  ( 26.06988505166722803, 42.64545166574268364, -7.025853678916862854 ) ) ;
#29391=CARTESIAN_POINT ( 'NONE',  ( 27.95245687107223986, 52.53944416759064495, 0.04044903254993640479 ) ) ;
#29395=CARTESIAN_POINT ( 'NONE',  ( -7.505752307973343918, 22.59895833333332860, -28.01184896238290989 ) ) ;
#29399=CARTESIAN_POINT ( 'NONE',  ( 26.00068869287340334, 50.81510416666667140, -15.01150461594642316 ) ) ;
#29405=CARTESIAN_POINT ( 'NONE',  ( -24.18731323226221974, 20.15847249907602290, 14.01125832528330406 ) ) ;
#29412=CARTESIAN_POINT ( 'NONE',  ( 27.95245687107222921, 33.91406249999997158, -2.463307335887066074E-13 ) ) ;
#29418=CARTESIAN_POINT ( 'NONE',  ( -7.025853678916393008, 60.41704833425730214, 26.06988505166735592 ) ) ;
#29430=CARTESIAN_POINT ( 'NONE',  ( 26.09010956794232428, 28.33371500092397355, -6.950374756619718042 ) ) ;
#29435=CARTESIAN_POINT ( 'NONE',  ( 7.505752307973351023, 51.81770833333332860, 28.01184896238290278 ) ) ;
#29439=CARTESIAN_POINT ( 'NONE',  ( -30.02300923189239512, 25.32031250000000000, 2.654126918244515359E-13 ) ) ;
#29445=CARTESIAN_POINT ( 'NONE',  ( -30.02300923189239867, 34.19493083240935505, 0.04044903255044988294 ) ) ;
#29447=CARTESIAN_POINT ( 'NONE',  ( -7.505752307972844761, 48.66666666666666430, 28.01184896238304134 ) ) ;
#29450=CARTESIAN_POINT ( 'NONE',  ( -27.95245687107223986, 65.13243083240935505, 0.04044903255043252877 ) ) ;
#29456=CARTESIAN_POINT ( 'NONE',  ( -27.95245687107223276, 21.88281249999999289, 2.498001805406602216E-13 ) ) ;
#29463=CARTESIAN_POINT ( 'NONE',  ( 13.94119854578893580, 28.46576416574268720, -24.22776226481265383 ) ) ;
#29466=CARTESIAN_POINT ( 'NONE',  ( -24.20753774853730889, 55.97135416666665719, 13.97622843553633842 ) ) ;
#29470=CARTESIAN_POINT ( 'NONE',  ( -28.01184896238290278, 28.61458333333333215, 7.505752307973363457 ) ) ;
#29471=CARTESIAN_POINT ( 'NONE',  ( 14.97647472619947351, 22.17486083425730925, 26.02091320914850314 ) ) ;
#29490=CARTESIAN_POINT ( 'NONE',  ( -19.11951029504763611, 36.64100666759062364, 19.06425588902592239 ) ) ;
#29498=CARTESIAN_POINT ( 'NONE',  ( 15.04653450569339945, 53.67409749907601935, 25.98046417659831775 ) ) ;
#29501=CARTESIAN_POINT ( 'NONE',  ( 6.988114217768294445, 27.75520833333332860, 26.07999730980477437 ) ) ;
#29504=CARTESIAN_POINT ( 'NONE',  ( 26.00068869287340334, 33.62760416666665719, -15.01150461594642316 ) ) ;
#29508=CARTESIAN_POINT ( 'NONE',  ( 7.468012846824777284, 46.38059000092397355, 28.02196122052045268 ) ) ;
#29510=CARTESIAN_POINT ( 'NONE',  ( 7.505752307972854531, 53.82291666666666430, -28.01184896238303423 ) ) ;
#29529=CARTESIAN_POINT ( 'NONE',  ( -24.20753774853756823, 66.85677083333334281, -13.97622843553588723 ) ) ;
#29534=CARTESIAN_POINT ( 'NONE',  ( -26.07999730980477437, 45.80208333333333570, 6.988114217768305103 ) ) ;
#29535=CARTESIAN_POINT ( 'NONE',  ( -28.00173670424549499, 40.65142333425730214, -7.543491769121417612 ) ) ;
#29536=CARTESIAN_POINT ( 'NONE',  ( 20.47846945139867003, 28.60899333240935150, -20.53372385742107653 ) ) ;
#29539=CARTESIAN_POINT ( 'NONE',  ( -19.11951029504797006, 51.81211833240936215, -19.06425588902558133 ) ) ;
#29546=CARTESIAN_POINT ( 'NONE',  ( -19.11951029504763611, 53.82850666759064495, 19.06425588902592239 ) ) ;
#29551=CARTESIAN_POINT ( 'NONE',  ( -7.505752307973343918, 26.03645833333333215, -28.01184896238290989 ) ) ;
#29555=CARTESIAN_POINT ( 'NONE',  ( 2.740863092043355209E-13, 62.27343749999999289, 30.02300923189239512 ) ) ;
#29561=CARTESIAN_POINT ( 'NONE',  ( 26.02091320914876960, 67.13763916574266943, 14.97647472619900455 ) ) ;
#29568=CARTESIAN_POINT ( 'NONE',  ( -6.988114217768288228, 39.78645833333332860, -26.07999730980477437 ) ) ;
#29574=CARTESIAN_POINT ( 'NONE',  ( -0.04044903254992426173, 60.27381916759065206, 27.95245687107223276 ) ) ;
#29576=CARTESIAN_POINT ( 'NONE',  ( 26.00068869287340334, 54.25260416666666430, -15.01150461594642316 ) ) ;
#29588=CARTESIAN_POINT ( 'NONE',  ( 19.11951029504763611, 21.17225666759064850, -19.06425588902591173 ) ) ;
#29594=CARTESIAN_POINT ( 'NONE',  ( -7.505752307973343918, 53.53645833333332860, -28.01184896238290989 ) ) ;
#29598=CARTESIAN_POINT ( 'NONE',  ( 15.01150461594643204, 31.04947916666666075, 26.00068869287340334 ) ) ;
#29605=CARTESIAN_POINT ( 'NONE',  ( 28.02196122052058413, 42.93190999907601935, 7.468012846824272799 ) ) ;
#29607=CARTESIAN_POINT ( 'NONE',  ( 20.50609665440969565, 50.67187500000000000, -20.50609665441004736 ) ) ;
#29609=CARTESIAN_POINT ( 'NONE',  ( 13.97622843553633665, 17.29947916666666430, 24.20753774853730889 ) ) ;
#29615=CARTESIAN_POINT ( 'NONE',  ( -19.09188309203660694, 24.89062500000000000, 19.09188309203694800 ) ) ;
#29622=CARTESIAN_POINT ( 'NONE',  ( 27.95245687107223276, 29.03868083240935505, -0.04044903255042905932 ) ) ;
#29626=CARTESIAN_POINT ( 'NONE',  ( -13.97622843553588901, 52.24739583333332860, 24.20753774853756823 ) ) ;
#29630=CARTESIAN_POINT ( 'NONE',  ( -26.00068869287368756, 25.60677083333332149, -15.01150461594595775 ) ) ;
#29631=CARTESIAN_POINT ( 'NONE',  ( -0.04044903254990864921, 25.89881916759064140, 30.02300923189239867 ) ) ;
#29640=CARTESIAN_POINT ( 'NONE',  ( -7.543491769121417612, 56.97954833425730925, 28.00173670424549499 ) ) ;
#29646=CARTESIAN_POINT ( 'NONE',  ( 19.06425588902558133, 38.92149333240934794, -19.11951029504797006 ) ) ;
#29652=CARTESIAN_POINT ( 'NONE',  ( 27.95245687107223986, 42.22694416759065206, 0.04044903254993640479 ) ) ;
#29661=CARTESIAN_POINT ( 'NONE',  ( 28.02196122052058413, 60.11940999907602645, 7.468012846824272799 ) ) ;
#29665=CARTESIAN_POINT ( 'NONE',  ( -19.09188309203694445, 22.31250000000000000, -19.09188309203661049 ) ) ;
#29667=CARTESIAN_POINT ( 'NONE',  ( 2.740863092043355209E-13, 34.77343750000000000, 30.02300923189239512 ) ) ;
#29670=CARTESIAN_POINT ( 'NONE',  ( -15.04653450569291984, 46.81027750092398776, 25.98046417659859486 ) ) ;
#29673=CARTESIAN_POINT ( 'NONE',  ( -15.01150461594595775, 59.12239583333333570, 26.00068869287368756 ) ) ;
#29693=CARTESIAN_POINT ( 'NONE',  ( 14.01125832528286352, 14.15402750092397532, -24.18731323226246843 ) ) ;
#29699=CARTESIAN_POINT ( 'NONE',  ( -26.07999730980490583, 46.08854166666666430, -6.988114217767815717 ) ) ;
#29701=CARTESIAN_POINT ( 'NONE',  ( -20.53372385742071771, 36.64100666759062364, 20.47846945139902530 ) ) ;
#29702=CARTESIAN_POINT ( 'NONE',  ( 26.02091320914876960, 29.32513916574269075, 14.97647472619900455 ) ) ;
#29706=CARTESIAN_POINT ( 'NONE',  ( -26.06988505166722803, 51.23920166574269786, 7.025853678916877953 ) ) ;
#29712=CARTESIAN_POINT ( 'NONE',  ( -24.18731323226248264, 54.54465250092398776, -14.01125832528284931 ) ) ;
#29716=CARTESIAN_POINT ( 'NONE',  ( 28.01184896238304134, 27.18229166666666430, 7.505752307972846538 ) ) ;
#29721=CARTESIAN_POINT ( 'NONE',  ( 7.505752307973351023, 62.13020833333334281, 28.01184896238290278 ) ) ;
#29728=CARTESIAN_POINT ( 'NONE',  ( 19.11951029504797006, 19.15586833240934794, 19.06425588902558133 ) ) ;
#29736=CARTESIAN_POINT ( 'NONE',  ( 13.97622843553633665, 44.79947916666667140, 24.20753774853730889 ) ) ;
#29743=CARTESIAN_POINT ( 'NONE',  ( -0.04044903254992426173, 63.71131916759064495, 27.95245687107223276 ) ) ;
#29744=CARTESIAN_POINT ( 'NONE',  ( 7.505752307973351023, 55.25520833333333570, 28.01184896238290278 ) ) ;
#29756=CARTESIAN_POINT ( 'NONE',  ( 19.11951029504763611, 24.60975666759063785, -19.06425588902591173 ) ) ;
#29761=CARTESIAN_POINT ( 'NONE',  ( 7.505752307972854531, 50.38541666666666430, -28.01184896238303423 ) ) ;
#29765=CARTESIAN_POINT ( 'NONE',  ( -20.50609665441004736, 29.18749999999999645, -20.50609665440969565 ) ) ;
#29770=CARTESIAN_POINT ( 'NONE',  ( -28.00173670424535644, 47.80170166574269786, 7.543491769121936308 ) ) ;
#29773=CARTESIAN_POINT ( 'NONE',  ( 28.01184896238290278, 50.95833333333332860, -7.505752307973347470 ) ) ;
#29777=CARTESIAN_POINT ( 'NONE',  ( 19.11951029504797006, 67.28086833240935505, 19.06425588902558133 ) ) ;
#29785=CARTESIAN_POINT ( 'NONE',  ( -2.428612866367529427E-13, 19.30468749999999645, -27.95245687107223276 ) ) ;
#29791=CARTESIAN_POINT ( 'NONE',  ( 30.02300923189239867, 29.03868083240935505, -0.04044903255044467877 ) ) ;
#29793=CARTESIAN_POINT ( 'NONE',  ( -19.11951029504797006, 27.74961833240935505, -19.06425588902558133 ) ) ;
#29798=CARTESIAN_POINT ( 'NONE',  ( -6.988114217767819270, 55.54166666666667140, 26.07999730980490583 ) ) ;
#29805=CARTESIAN_POINT ( 'NONE',  ( -26.00068869287340334, 21.59635416666666785, 15.01150461594643382 ) ) ;
#29806=CARTESIAN_POINT ( 'NONE',  ( 7.543491769121427382, 20.88579833425730925, -28.00173670424548433 ) ) ;
#29815=CARTESIAN_POINT ( 'NONE',  ( -26.02091320914849959, 57.40923583425731636, 14.97647472619947528 ) ) ;
#29817=CARTESIAN_POINT ( 'NONE',  ( -26.00068869287340334, 21.59635416666666430, 15.01150461594643559 ) ) ;
#29822=CARTESIAN_POINT ( 'NONE',  ( -6.950374756619247307, 43.79128499907601935, 26.09010956794245217 ) ) ;
#29830=CARTESIAN_POINT ( 'NONE',  ( -27.95245687107223986, 40.50819416759064495, -0.04044903254993292840 ) ) ;
#29837=CARTESIAN_POINT ( 'NONE',  ( 28.00173670424535644, 56.39545166574268364, -7.543491769121920321 ) ) ;
#29840=CARTESIAN_POINT ( 'NONE',  ( 6.988114217767829928, 26.32291666666666075, -26.07999730980489872 ) ) ;
#29844=CARTESIAN_POINT ( 'NONE',  ( -15.01150461594595775, 31.62239583333332860, 26.00068869287368756 ) ) ;
#29845=( BOUNDED_CURVE ( )  B_SPLINE_CURVE ( 2, ( #15598, #17826, #31196, #7686, #12664, #33599, #2546, #33780, #28615, #13013, #33425, #23484, #23133, #28788, #20399, #9922, #5287, #25710, #15769, #28283, #20578, #4770, #7520, #33945, #15247, #10437, #28449, #26224, #4940, #7855, #15422, #18343, #116, #21086, #2190, #31535, #25876, #2369, #5456, #15937, #12498, #24157, #291, #19178, #24323, #13528, #21914, #19341, #3548, #8357, #31701, #29785, #5958, #796, #21256, #13858, #32364, #8858, #11437, #11279, #29123, #3057, #8528, #14020, #3224, #5791, #16765, #16602, #27055, #29456, #26561, #11117, #21756, #8193, #24483, #32201, #23992, #16438, #18684, #627, #32031, #19013, #26890, #31863, #463, #3388, #21585, #8694, #957, #6289, #29615, #6117, #2886, #13352, #23826, #13692, #10779, #5626, #16110, #10946, #21421, #18845, #29292, #16272, #26730, #30119, #15168, #4862, #7437, #10020, #7256, #11602, #4517, #6622, #14992, #33342, #25462, #17743, #1937, #24643, #20491, #28203, #10192, #17923, #22885, #15342, #9839, #20317, #28374, #4689, #1117, #12415, #17101, #9028, #14354, #30942, #25634, #12761, #25797, #2113, #19509, #30766, #12586, #23233, #23056, #16934, #33515, #2286, #33693, #20675, #27560, #31114, #27392, #7608, #11768, #9189, #27223, #3717, #32694, #14187, #22084, #32527, #29956, #6460, #3881, #24813, #1289, #22251, #19673, #18765, #10526, #13614, #18600, #31282, #18262, #5715, #23741, #24079, #21003, #16024, #18433, #7775, #15854, #2636, #37, #5373, #26310, #23572, #16193, #31452, #26479, #5031, #2799, #7945, #23909, #28708, #31949, #26647, #20837, #29209, #28877, #5206, #5543, #15690, #13266, #2972, #21174, #13442, #2462, #29040, #544, #3141, #11032, #380, #10359, #18088, #205, #21501, #28536, #12928, #10866, #31781, #8273, #10693, #26139, #31616, #21340, #23405, #15517, #25968, #13099, #8113, #33866, #6204, #3635, #8613, #29534, #11519, #29699, #16684, #27141, #16854, #22171, #32615, #14109, #24566, #22335, #8948, #1039, #19258, #21999, #17019, #16356, #6037, #32447, #3306, #29876, #26968, #11687, #3469, #19426, #19593, #9112, #24731, #6376, #26811, #27311, #21837, #3802, #14274, #1206, #30041, #6546, #5878, #27479, #3968, #19096, #14441, #24896, #1382, #13939, #11856, #8442, #18933, #13771, #29379, #32282, #24241, #16516, #712, #11198, #21669, #32115, #24403, #879, #8775, #11359, #1549, #32780, #12025, #9274, #6709, #14612, #19758, #4137, #25068, #30207, #17191, #27649, #23773, #20866, #5407, #16057, #2493, #21371, #5576, #7806, #241, #12962, #28906, #26342, #13300, #10727, #26175, #18295, #21204, #18462, #26512, #10898, #31815, #15886, #31648, #11067, #8146, #18635, #7976, #2831, #5745, #5063, #28740, #29072, #15720, #26000, #5236, #16226, #69, #3005, #8306, #18797, #13478, #23943, #15548, #412, #10555, #29241, #26680, #3176, #13645, #24109, #28567, #577, #31147, #7638, #18120, #23436, #33897, #10388, #31312, #2669, #13128, #23602, #21036, #31486, #17580, #7268, #5040, #15002, #4355, #22543, #12594, #25297, #23065, #20683, #19981, #15352 ),
 .UNSPECIFIED., .F., .T. ) 
 B_SPLINE_CURVE_WITH_KNOTS ( ( 3, 2, 2, 2, 2, 2, 2, 2, 2, 2, 2, 2, 2, 2, 2, 2, 2, 2, 2, 2, 2, 2, 2, 2, 2, 2, 2, 2, 2, 2, 2, 2, 2, 2, 2, 2, 2, 2, 2, 2, 2, 2, 2, 2, 2, 2, 2, 2, 2, 2, 2, 2, 2, 2, 2, 2, 2, 2, 2, 2, 2, 2, 2, 2, 2, 2, 2, 2, 2, 2, 2, 2, 2, 2, 2, 2, 2, 2, 2, 2, 2, 2, 2, 2, 2, 2, 2, 2, 2, 2, 2, 2, 2, 2, 2, 2, 2, 2, 2, 2, 2, 2, 2, 2, 2, 2, 2, 2, 2, 2, 2, 2, 2, 2, 2, 2, 2, 2, 2, 2, 2, 2, 2, 2, 2, 2, 2, 2, 2, 2, 2, 2, 2, 2, 2, 2, 2, 2, 2, 2, 2, 2, 2, 2, 2, 2, 2, 2, 2, 2, 2, 2, 2, 2, 2, 2, 2, 2, 2, 2, 2, 2, 2, 2, 2, 2, 2, 2, 2, 2, 2, 2, 2, 2, 2, 2, 2, 2, 2, 2, 2, 2, 2, 2, 2, 2, 2, 2, 2, 2, 2, 2, 3 ),
 ( 0.000000000000000000, 0.005208333333333333044, 0.01041666666666666609, 0.01562500000000000000, 0.02083333333333333218, 0.02604166666666666782, 0.03125000000000000000, 0.03645833333333333565, 0.04166666666666666435, 0.04687500000000000000, 0.05208333333333333565, 0.05729166666666666435, 0.06250000000000000000, 0.06770833333333332871, 0.07291666666666667129, 0.07812500000000000000, 0.08333333333333332871, 0.08854166666666667129, 0.09375000000000000000, 0.09895833333333332871, 0.1041666666666666713, 0.1093750000000000000, 0.1145833333333333287, 0.1197916666666666713, 0.1250000000000000000, 0.1302083333333333426, 0.1354166666666666574, 0.1406250000000000000, 0.1458333333333333426, 0.1510416666666666574, 0.1562500000000000000, 0.1614583333333333426, 0.1666666666666666574, 0.1718750000000000000, 0.1770833333333333426, 0.1822916666666666574, 0.1875000000000000000, 0.1927083333333333426, 0.1979166666666666574, 0.2031250000000000000, 0.2083333333333333426, 0.2135416666666666574, 0.2187500000000000000, 0.2239583333333333426, 0.2291666666666666574, 0.2343750000000000000, 0.2395833333333333426, 0.2447916666666666574, 0.2500000000000000000, 0.2552083333333333148, 0.2604166666666666852, 0.2656250000000000000, 0.2708333333333333148, 0.2760416666666666852, 0.2812500000000000000, 0.2864583333333333148, 0.2916666666666666852, 0.2968750000000000000, 0.3020833333333333148, 0.3072916666666666852, 0.3125000000000000000, 0.3177083333333333148, 0.3229166666666666852, 0.3281250000000000000, 0.3333333333333333148, 0.3385416666666666852, 0.3437500000000000000, 0.3489583333333333148, 0.3541666666666666852, 0.3593750000000000000, 0.3645833333333333148, 0.3697916666666666852, 0.3750000000000000000, 0.3802083333333333148, 0.3854166666666666852, 0.3906250000000000000, 0.3958333333333333148, 0.4010416666666666852, 0.4062500000000000000, 0.4114583333333333148, 0.4166666666666666852, 0.4218750000000000000, 0.4270833333333333148, 0.4322916666666666852, 0.4375000000000000000, 0.4427083333333333148, 0.4479166666666666852, 0.4531250000000000000, 0.4583333333333333148, 0.4635416666666666852, 0.4687500000000000000, 0.4739583333333333148, 0.4791666666666666852, 0.4843750000000000000, 0.4895833333333333148, 0.4947916666666666852, 0.5000000000000000000, 0.5052083333333333703, 0.5104166666666666297, 0.5156250000000000000, 0.5208333333333333703, 0.5260416666666666297, 0.5312500000000000000, 0.5364583333333333703, 0.5416666666666666297, 0.5468750000000000000, 0.5520833333333333703, 0.5572916666666666297, 0.5625000000000000000, 0.5677083333333333703, 0.5729166666666666297, 0.5781250000000000000, 0.5833333333333333703, 0.5885416666666666297, 0.5937500000000000000, 0.5989583333333333703, 0.6041666666666666297, 0.6093750000000000000, 0.6145833333333333703, 0.6197916666666666297, 0.6250000000000000000, 0.6302083333333333703, 0.6354166666666666297, 0.6406250000000000000, 0.6458333333333333703, 0.6510416666666666297, 0.6562500000000000000, 0.6614583333333333703, 0.6666666666666666297, 0.6718750000000000000, 0.6770833333333333703, 0.6822916666666666297, 0.6875000000000000000, 0.6927083333333333703, 0.6979166666666666297, 0.7031250000000000000, 0.7083333333333333703, 0.7135416666666666297, 0.7187500000000000000, 0.7239583333333333703, 0.7291666666666666297, 0.7343750000000000000, 0.7395833333333333703, 0.7447916666666666297, 0.7500000000000000000, 0.7552083333333333703, 0.7604166666666666297, 0.7656250000000000000, 0.7708333333333333703, 0.7760416666666666297, 0.7812500000000000000, 0.7864583333333333703, 0.7916666666666666297, 0.7968750000000000000, 0.8020833333333333703, 0.8072916666666666297, 0.8125000000000000000, 0.8177083333333333703, 0.8229166666666666297, 0.8281250000000000000, 0.8333333333333333703, 0.8385416666666666297, 0.8437500000000000000, 0.8489583333333333703, 0.8541666666666666297, 0.8593750000000000000, 0.8645833333333333703, 0.8697916666666666297, 0.8750000000000000000, 0.8802083333333333703, 0.8854166666666666297, 0.8906250000000000000, 0.8958333333333333703, 0.9010416666666666297, 0.9062500000000000000, 0.9114583333333333703, 0.9166666666666666297, 0.9218750000000000000, 0.9270833333333333703, 0.9322916666666666297, 0.9375000000000000000, 0.9427083333333333703, 0.9479166666666666297, 0.9531250000000000000, 0.9583333333333333703, 0.9635416666666666297, 0.9687500000000000000, 0.9739583333333333703, 0.9791666666666666297, 0.9843750000000000000, 0.9895833333333333703, 0.9947916666666666297, 1.000000000000000000 ),
 .UNSPECIFIED. ) 
 CURVE ( )  GEOMETRIC_REPRESENTATION_ITEM ( )  RATIONAL_B_SPLINE_CURVE ( ( 1.000000000000000000, 0.9659258262890683122, 1.000000000000000000, 0.9659258262890683122, 1.000000000000000000, 0.9659258262890683122, 1.000000000000000000, 0.9659258262890683122, 1.000000000000000000, 0.9659258262890683122, 1.000000000000000000, 0.9659258262890683122, 1.000000000000000000, 0.9659258262890683122, 1.000000000000000000, 0.9659258262890683122, 1.000000000000000000, 0.9659258262890683122, 1.000000000000000000, 0.9659258262890683122, 1.000000000000000000, 0.9659258262890683122, 1.000000000000000000, 0.9659258262890683122, 1.000000000000000000, 0.9659258262890683122, 1.000000000000000000, 0.9659258262890683122, 1.000000000000000000, 0.9659258262890683122, 1.000000000000000000, 0.9659258262890683122, 1.000000000000000000, 0.9659258262890683122, 1.000000000000000000, 0.9659258262890683122, 1.000000000000000000, 0.9659258262890683122, 1.000000000000000000, 0.9659258262890683122, 1.000000000000000000, 0.9659258262890683122, 1.000000000000000000, 0.9659258262890683122, 1.000000000000000000, 0.9659258262890683122, 1.000000000000000000, 0.9659258262890683122, 1.000000000000000000, 0.9659258262890683122, 1.000000000000000000, 0.9659258262890683122, 1.000000000000000000, 0.9659258262890683122, 1.000000000000000000, 0.9659258262890683122, 1.000000000000000000, 0.9659258262890683122, 1.000000000000000000, 0.9659258262890683122, 1.000000000000000000, 0.9659258262890683122, 1.000000000000000000, 0.9659258262890683122, 1.000000000000000000, 0.9659258262890683122, 1.000000000000000000, 0.9659258262890683122, 1.000000000000000000, 0.9659258262890683122, 1.000000000000000000, 0.9659258262890683122, 1.000000000000000000, 0.9659258262890683122, 1.000000000000000000, 0.9659258262890683122, 1.000000000000000000, 0.9659258262890683122, 1.000000000000000000, 0.9659258262890683122, 1.000000000000000000, 0.9659258262890683122, 1.000000000000000000, 0.9659258262890683122, 1.000000000000000000, 0.9659258262890683122, 1.000000000000000000, 0.9659258262890683122, 1.000000000000000000, 0.9659258262890683122, 1.000000000000000000, 0.9659258262890683122, 1.000000000000000000, 0.9659258262890683122, 1.000000000000000000, 0.9659258262890683122, 1.000000000000000000, 0.9659258262890683122, 1.000000000000000000, 0.9659258262890683122, 1.000000000000000000, 0.9659258262890683122, 1.000000000000000000, 0.9659258262890683122, 1.000000000000000000, 0.9659258262890683122, 1.000000000000000000, 0.9659258262890683122, 1.000000000000000000, 0.9659258262890683122, 1.000000000000000000, 0.9659258262890683122, 1.000000000000000000, 0.9659258262890683122, 1.000000000000000000, 0.9659258262890683122, 1.000000000000000000, 0.9659258262890683122, 1.000000000000000000, 0.9659258262890683122, 1.000000000000000000, 0.9659258262890683122, 1.000000000000000000, 0.9659258262890683122, 1.000000000000000000, 0.9659258262890683122, 1.000000000000000000, 0.9659258262890683122, 1.000000000000000000, 0.9659258262890683122, 1.000000000000000000, 0.9659258262890683122, 1.000000000000000000, 0.9659258262890683122, 1.000000000000000000, 0.9659258262890683122, 1.000000000000000000, 0.9659258262890683122, 1.000000000000000000, 0.9659258262890683122, 1.000000000000000000, 0.9659258262890683122, 1.000000000000000000, 0.9659258262890683122, 1.000000000000000000, 0.9659258262890683122, 1.000000000000000000, 0.9659258262890683122, 1.000000000000000000, 0.9659258262890683122, 1.000000000000000000, 0.9659258262890683122, 1.000000000000000000, 0.9659258262890683122, 1.000000000000000000, 0.9659258262890683122, 1.000000000000000000, 0.9659258262890683122, 1.000000000000000000, 0.9659258262890683122, 1.000000000000000000, 0.9659258262890683122, 1.000000000000000000, 0.9659258262890683122, 1.000000000000000000, 0.9659258262890683122, 1.000000000000000000, 0.9659258262890683122, 1.000000000000000000, 0.9659258262890683122, 1.000000000000000000, 0.9659258262890683122, 1.000000000000000000, 0.9659258262890683122, 1.000000000000000000, 0.9659258262890683122, 1.000000000000000000, 0.9659258262890683122, 1.000000000000000000, 0.9659258262890683122, 1.000000000000000000, 0.9659258262890683122, 1.000000000000000000, 0.9659258262890683122, 1.000000000000000000, 0.9659258262890683122, 1.000000000000000000, 0.9659258262890683122, 1.000000000000000000, 0.9659258262890683122, 1.000000000000000000, 0.9659258262890683122, 1.000000000000000000, 0.9659258262890683122, 1.000000000000000000, 0.9659258262890683122, 1.000000000000000000, 0.9659258262890683122, 1.000000000000000000, 0.9659258262890683122, 1.000000000000000000, 0.9659258262890683122, 1.000000000000000000, 0.9659258262890683122, 1.000000000000000000, 0.9659258262890683122, 1.000000000000000000, 0.9659258262890683122, 1.000000000000000000, 0.9659258262890683122, 1.000000000000000000, 0.9659258262890683122, 1.000000000000000000, 0.9659258262890683122, 1.000000000000000000, 0.9659258262890683122, 1.000000000000000000, 0.9659258262890683122, 1.000000000000000000, 0.9659258262890683122, 1.000000000000000000, 0.9659258262890683122, 1.000000000000000000, 0.9659258262890683122, 1.000000000000000000, 0.9659258262890683122, 1.000000000000000000, 0.9659258262890683122, 1.000000000000000000, 0.9659258262890683122, 1.000000000000000000, 0.9659258262890683122, 1.000000000000000000, 0.9659258262890683122, 1.000000000000000000, 0.9659258262890683122, 1.000000000000000000, 0.9659258262890683122, 1.000000000000000000, 0.9659258262890683122, 1.000000000000000000, 0.9659258262890683122, 1.000000000000000000, 0.9659258262890683122, 1.000000000000000000, 0.9659258262890683122, 1.000000000000000000, 0.9659258262890683122, 1.000000000000000000, 0.9659258262890683122, 1.000000000000000000, 0.9659258262890683122, 1.000000000000000000, 0.9659258262890683122, 1.000000000000000000, 0.9659258262890683122, 1.000000000000000000, 0.9659258262890683122, 1.000000000000000000, 0.9659258262890683122, 1.000000000000000000, 0.9659258262890683122, 1.000000000000000000, 0.9659258262890683122, 1.000000000000000000, 0.9659258262890683122, 1.000000000000000000, 0.9659258262890683122, 1.000000000000000000, 0.9659258262890683122, 1.000000000000000000, 0.9659258262890683122, 1.000000000000000000, 0.9659258262890683122, 1.000000000000000000, 0.9659258262890683122, 1.000000000000000000, 0.9659258262890683122, 1.000000000000000000, 0.9659258262890683122, 1.000000000000000000, 0.9659258262890683122, 1.000000000000000000, 0.9659258262890683122, 1.000000000000000000, 0.9659258262890683122, 1.000000000000000000, 0.9659258262890683122, 1.000000000000000000, 0.9659258262890683122, 1.000000000000000000, 0.9659258262890683122, 1.000000000000000000, 0.9659258262890683122, 1.000000000000000000, 0.9659258262890683122, 1.000000000000000000, 0.9659258262890683122, 1.000000000000000000, 0.9659258262890683122, 1.000000000000000000, 0.9659258262890683122, 1.000000000000000000, 0.9659258262890683122, 1.000000000000000000, 0.9659258262890683122, 1.000000000000000000, 0.9659258262890683122, 1.000000000000000000, 0.9659258262890683122, 1.000000000000000000, 0.9659258262890683122, 1.000000000000000000, 0.9659258262890683122, 1.000000000000000000, 0.9659258262890683122, 1.000000000000000000, 0.9659258262890683122, 1.000000000000000000, 0.9659258262890683122, 1.000000000000000000, 0.9659258262890683122, 1.000000000000000000, 0.9659258262890683122, 1.000000000000000000, 0.9659258262890683122, 1.000000000000000000, 0.9659258262890683122, 1.000000000000000000, 0.9659258262890683122, 1.000000000000000000, 0.9659258262890683122, 1.000000000000000000, 0.9659258262890683122, 1.000000000000000000, 0.9659258262890683122, 1.000000000000000000, 0.9659258262890683122, 1.000000000000000000, 0.9659258262890683122, 1.000000000000000000, 0.9659258262890683122, 1.000000000000000000, 0.9659258262890683122, 1.000000000000000000, 0.9659258262890683122, 1.000000000000000000, 0.9659258262890683122, 1.000000000000000000, 0.9659258262890683122, 1.000000000000000000, 0.9659258262890683122, 1.000000000000000000, 0.9659258262890683122, 1.000000000000000000, 0.9659258262890683122, 1.000000000000000000, 0.9659258262890683122, 1.000000000000000000, 0.9659258262890683122, 1.000000000000000000, 0.9659258262890683122, 1.000000000000000000, 0.9659258262890683122, 1.000000000000000000, 0.9659258262890683122, 1.000000000000000000, 0.9659258262890683122, 1.000000000000000000, 0.9659258262890683122, 1.000000000000000000, 0.9659258262890683122, 1.000000000000000000, 0.9659258262890683122, 1.000000000000000000, 0.9659258262890683122, 1.000000000000000000, 0.9659258262890683122, 1.000000000000000000, 0.9659258262890683122, 1.000000000000000000, 0.9659258262890683122, 1.000000000000000000, 0.9659258262890683122, 1.000000000000000000 ) ) 
 REPRESENTATION_ITEM ( '' )  );
#29849=CARTESIAN_POINT ( 'NONE',  ( -7.543491769121417612, 50.10454833425731636, 28.00173670424549499 ) ) ;
#29851=CARTESIAN_POINT ( 'NONE',  ( 15.01150461594596308, 64.27864583333332860, -26.00068869287367335 ) ) ;
#29871=CARTESIAN_POINT ( 'NONE',  ( 14.01125832528286352, 10.71652750092397888, -24.18731323226246843 ) ) ;
#29876=CARTESIAN_POINT ( 'NONE',  ( -6.988114217767819270, 48.66666666666666430, 26.07999730980490583 ) ) ;
#29877=CARTESIAN_POINT ( 'NONE',  ( 30.02300923189239867, 42.22694416759065206, 0.04044903254992252006 ) ) ;
#29878=CARTESIAN_POINT ( 'NONE',  ( -7.468012846824272799, 30.04128499907601224, 28.02196122052058413 ) ) ;
#29881=CARTESIAN_POINT ( 'NONE',  ( 24.22776226481265383, 53.38763916574269786, 13.94119854578893580 ) ) ;
#29889=CARTESIAN_POINT ( 'NONE',  ( 28.01184896238304134, 37.49479166666666430, 7.505752307972846538 ) ) ;
#29894=CARTESIAN_POINT ( 'NONE',  ( -7.505752307972844761, 55.54166666666667140, 28.01184896238304134 ) ) ;
#29902=CARTESIAN_POINT ( 'NONE',  ( -24.18731323226221974, 16.72097249907602290, 14.01125832528330406 ) ) ;
#29911=CARTESIAN_POINT ( 'NONE',  ( 2.584737979205441561E-13, 38.21093750000000000, 27.95245687107222921 ) ) ;
#29918=CARTESIAN_POINT ( 'NONE',  ( -30.02300923189239867, 13.00819416759064318, -0.04044903254991731589 ) ) ;
#29919=CARTESIAN_POINT ( 'NONE',  ( -2.584737979205441561E-13, 57.11718750000000711, -30.02300923189239512 ) ) ;
#29930=CARTESIAN_POINT ( 'NONE',  ( 7.025853678916403666, 24.32329833425730214, -26.06988505166735237 ) ) ;
#29935=CARTESIAN_POINT ( 'NONE',  ( -30.02300923189239512, 52.82031249999997868, 2.654126918244515359E-13 ) ) ;
#29939=CARTESIAN_POINT ( 'NONE',  ( 7.505752307973351023, 27.75520833333332860, 28.01184896238290278 ) ) ;
#29944=CARTESIAN_POINT ( 'NONE',  ( 14.97647472619900455, 42.21576416574269075, -26.02091320914876960 ) ) ;
#29946=CARTESIAN_POINT ( 'NONE',  ( -20.50609665441004736, 56.68749999999998579, -20.50609665440969565 ) ) ;
#29950=CARTESIAN_POINT ( 'NONE',  ( -26.09010956794245217, 68.71315999907601224, -6.950374756619243755 ) ) ;
#29956=CARTESIAN_POINT ( 'NONE',  ( -19.09188309203660694, 35.20312500000000000, 19.09188309203694800 ) ) ;
#29961=CARTESIAN_POINT ( 'NONE',  ( 7.468012846824281681, 21.44753499907601579, -28.02196122052058058 ) ) ;
#29963=CARTESIAN_POINT ( 'NONE',  ( -24.18731323226221974, 40.78347249907601935, 14.01125832528330406 ) ) ;
#29967=CARTESIAN_POINT ( 'NONE',  ( 2.584737979205441561E-13, 55.39843749999999289, 27.95245687107222921 ) ) ;
#29973=CARTESIAN_POINT ( 'NONE',  ( 15.01150461594643204, 24.17447916666666785, 26.00068869287340334 ) ) ;
#29974=CARTESIAN_POINT ( 'NONE',  ( 7.543491769121427382, 24.32329833425730214, -28.00173670424548433 ) ) ;
#29983=CARTESIAN_POINT ( 'NONE',  ( 14.97647472619947351, 53.11236083425731636, 26.02091320914850314 ) ) ;
#29986=CARTESIAN_POINT ( 'NONE',  ( -26.00068869287340334, 31.90885416666666785, 15.01150461594643559 ) ) ;
#29991=CARTESIAN_POINT ( 'NONE',  ( -19.06425588902558133, 47.51524333240936215, 19.11951029504797006 ) ) ;
#29997=CARTESIAN_POINT ( 'NONE',  ( -19.06425588902591173, 37.50038166759063074, -19.11951029504763611 ) ) ;
#30004=CARTESIAN_POINT ( 'NONE',  ( -20.53372385742107653, 51.81211833240936215, -20.47846945139867003 ) ) ;
#30009=CARTESIAN_POINT ( 'NONE',  ( -19.09188309203694445, 29.18749999999999645, -19.09188309203661049 ) ) ;
#30011=CARTESIAN_POINT ( 'NONE',  ( 20.50609665441005092, 30.90624999999999645, 20.50609665440969209 ) ) ;
#30016=CARTESIAN_POINT ( 'NONE',  ( 28.02196122052045268, 48.95871500092396644, -7.468012846824774620 ) ) ;
#30018=CARTESIAN_POINT ( 'NONE',  ( -15.01150461594595775, 62.55989583333332860, 26.00068869287368756 ) ) ;
#30036=CARTESIAN_POINT ( 'NONE',  ( 24.22776226481241224, 11.00298583425731103, -13.94119854578936923 ) ) ;
#30041=CARTESIAN_POINT ( 'NONE',  ( 24.20753774853731244, 50.81510416666666430, -13.97622843553633132 ) ) ;
#30042=CARTESIAN_POINT ( 'NONE',  ( 7.543491769121427382, 41.51079833425730214, -28.00173670424548433 ) ) ;
#30043=CARTESIAN_POINT ( 'NONE',  ( 30.02300923189239867, 25.60118083240935860, -0.04044903255044467877 ) ) ;
#30046=CARTESIAN_POINT ( 'NONE',  ( 26.09010956794244507, 56.68190999907602645, 6.950374756619249084 ) ) ;
#30054=CARTESIAN_POINT ( 'NONE',  ( 15.01150461594596308, 29.90364583333332504, -26.00068869287367335 ) ) ;
#30058=CARTESIAN_POINT ( 'NONE',  ( -28.01184896238304134, 59.83854166666666430, -7.505752307972844761 ) ) ;
#30065=CARTESIAN_POINT ( 'NONE',  ( 24.22776226481265383, 19.01263916574269075, 13.94119854578893580 ) ) ;
#30073=CARTESIAN_POINT ( 'NONE',  ( -2.428612866367529427E-13, 43.36718749999999289, -27.95245687107222921 ) ) ;
#30078=CARTESIAN_POINT ( 'NONE',  ( 20.53372385742072481, 10.85975666759064318, -20.47846945139902175 ) ) ;
#30079=CARTESIAN_POINT ( 'NONE',  ( -2.584737979205441561E-13, 53.67968750000000000, -30.02300923189239512 ) ) ;
#30089=CARTESIAN_POINT ( 'NONE',  ( -26.09010956794232428, 33.48996500092397355, 6.950374756619732253 ) ) ;
#30094=CARTESIAN_POINT ( 'NONE',  ( -26.00068869287368756, 56.54427083333332149, -15.01150461594595775 ) ) ;
#30098=CARTESIAN_POINT ( 'NONE',  ( -20.50609665440969209, 28.32812499999999645, 20.50609665441005092 ) ) ;
#30104=CARTESIAN_POINT ( 'NONE',  ( 20.47846945139867003, 45.79649333240935505, -20.53372385742107653 ) ) ;
#30106=CARTESIAN_POINT ( 'NONE',  ( 26.00068869287367690, 61.70052083333332860, 15.01150461594596486 ) ) ;
#30112=CARTESIAN_POINT ( 'NONE',  ( -2.428612866367529427E-13, 12.42968749999999289, -27.95245687107222921 ) ) ;
#30119=CARTESIAN_POINT ( 'NONE',  ( 27.95245687107223276, 27.03906250000000000, -2.463307335887066074E-13 ) ) ;
#30124=CARTESIAN_POINT ( 'NONE',  ( 20.47846945139867003, 21.73399333240935505, -20.53372385742107653 ) ) ;
#30126=CARTESIAN_POINT ( 'NONE',  ( -27.95245687107223986, 34.19493083240935505, 0.04044903255043252877 ) ) ;
#30130=CARTESIAN_POINT ( 'NONE',  ( -13.97622843553588901, 59.12239583333333570, 24.20753774853756823 ) ) ;
#30135=CARTESIAN_POINT ( 'NONE',  ( -7.505752307972844761, 21.16666666666666430, 28.01184896238304134 ) ) ;
#30136=CARTESIAN_POINT ( 'NONE',  ( 20.53372385742072481, 28.04725666759063429, -20.47846945139902175 ) ) ;
#30145=CARTESIAN_POINT ( 'NONE',  ( 28.00173670424549499, 56.12017333425732346, 7.543491769121417612 ) ) ;
#30149=CARTESIAN_POINT ( 'NONE',  ( 2.740863092043355209E-13, 31.33593749999999289, 30.02300923189239867 ) ) ;
#30153=CARTESIAN_POINT ( 'NONE',  ( -19.06425588902558133, 40.64024333240936215, 19.11951029504797006 ) ) ;
#30159=CARTESIAN_POINT ( 'NONE',  ( 24.18731323226247554, 45.95090250092398065, 14.01125832528285997 ) ) ;
#30167=CARTESIAN_POINT ( 'NONE',  ( -20.53372385742107653, 62.12461833240934794, -20.47846945139867003 ) ) ;
#30172=CARTESIAN_POINT ( 'NONE',  ( -27.95245687107222921, 25.32031250000000000, 2.498001805406602216E-13 ) ) ;
#30175=CARTESIAN_POINT ( 'NONE',  ( 26.00068869287367335, 41.07552083333331439, 15.01150461594596308 ) ) ;
#30178=CARTESIAN_POINT ( 'NONE',  ( 0.04044903254992426173, 51.68006916759063785, -30.02300923189239867 ) ) ;
#30180=CARTESIAN_POINT ( 'NONE',  ( -2.584737979205441561E-13, 60.55468749999999289, -30.02300923189239512 ) ) ;
#30201=CARTESIAN_POINT ( 'NONE',  ( -7.025853678916393008, 22.60454833425730925, 26.06988505166735592 ) ) ;
#30207=CARTESIAN_POINT ( 'NONE',  ( -19.09188309203660694, 55.82812499999999289, 19.09188309203694800 ) ) ;
#30208=CARTESIAN_POINT ( 'NONE',  ( -30.02300923189239867, 40.50819416759064495, -0.04044903254991731589 ) ) ;
#30210=CARTESIAN_POINT ( 'NONE',  ( -7.543491769121917656, 38.34857666574267654, -28.00173670424536354 ) ) ;
#30213=CARTESIAN_POINT ( 'NONE',  ( -13.94119854578892514, 54.24701416574269075, 24.22776226481266448 ) ) ;
#30222=CARTESIAN_POINT ( 'NONE',  ( 26.00068869287367335, 30.76302083333332504, 15.01150461594596308 ) ) ;
#30226=CARTESIAN_POINT ( 'NONE',  ( 28.01184896238304134, 61.55729166666666430, 7.505752307972846538 ) ) ;
#30232=CARTESIAN_POINT ( 'NONE',  ( 14.01125832528330051, 26.17409749907601935, 24.18731323226221974 ) ) ;
#30240=CARTESIAN_POINT ( 'NONE',  ( -13.97622843553588901, 45.37239583333333570, 24.20753774853756823 ) ) ;
#30245=CARTESIAN_POINT ( 'NONE',  ( 30.02300923189239867, 14.72694416759064318, 0.04044903254992252006 ) ) ;
#30247=CARTESIAN_POINT ( 'NONE',  ( 20.50609665441005092, 51.53124999999999289, 20.50609665440969209 ) ) ;
#30260=CARTESIAN_POINT ( 'NONE',  ( -19.06425588902591173, 30.62538166759064495, -19.11951029504763611 ) ) ;
#30267=CARTESIAN_POINT ( 'NONE',  ( -28.01184896238304134, 59.83854166666666430, -7.505752307972844761 ) ) ;
#30271=CARTESIAN_POINT ( 'NONE',  ( 7.505752307973351023, 34.63020833333332860, 28.01184896238290278 ) ) ;
#30276=CARTESIAN_POINT ( 'NONE',  ( -30.02300923189239867, 44.50743083240935505, 0.04044903255044988294 ) ) ;
#30278=CARTESIAN_POINT ( 'NONE',  ( 28.01184896238290278, 57.83333333333333570, -7.505752307973347470 ) ) ;
#30282=CARTESIAN_POINT ( 'NONE',  ( 24.20753774853756113, 17.01302083333332504, 13.97622843553589789 ) ) ;
#30293=CARTESIAN_POINT ( 'NONE',  ( -15.04653450569338524, 24.45534749907602290, -25.98046417659831775 ) ) ;
#30295=CARTESIAN_POINT ( 'NONE',  ( -24.18731323226221974, 33.90847249907601935, 14.01125832528330406 ) ) ;
#30299=CARTESIAN_POINT ( 'NONE',  ( -24.20753774853730889, 59.40885416666666430, 13.97622843553633842 ) ) ;
#30306=CARTESIAN_POINT ( 'NONE',  ( -15.01150461594642138, 32.76822916666666430, -26.00068869287340334 ) ) ;
#30307=CARTESIAN_POINT ( 'NONE',  ( 26.02091320914851025, 31.62798583425730925, -14.97647472619946463 ) ) ;
#30317=CARTESIAN_POINT ( 'NONE',  ( -20.50609665441004736, 11.99999999999999645, -20.50609665440969565 ) ) ;
#30318=CARTESIAN_POINT ( 'NONE',  ( 28.02196122052045268, 59.27121500092397355, -7.468012846824774620 ) ) ;
#30321=CARTESIAN_POINT ( 'NONE',  ( 20.50609665440969565, 30.04687500000000000, -20.50609665441004736 ) ) ;
#30326=CARTESIAN_POINT ( 'NONE',  ( 0.04044903255044120238, 40.21055583240935505, 27.95245687107223276 ) ) ;
#30332=CARTESIAN_POINT ( 'NONE',  ( -14.01125832528285109, 46.81027750092398776, 24.18731323226248264 ) ) ;
#30340=CARTESIAN_POINT ( 'NONE',  ( -26.02091320914878025, 68.85638916574269786, -14.97647472619899389 ) ) ;
#30343=CARTESIAN_POINT ( 'NONE',  ( 26.07999730980477437, 37.20833333333332860, -6.988114217768290004 ) ) ;
#30346=CARTESIAN_POINT ( 'NONE',  ( -15.01150461594642138, 39.64322916666667140, -26.00068869287340334 ) ) ;
#30349=CARTESIAN_POINT ( 'NONE',  ( -0.04044903254990864921, 60.27381916759065206, 30.02300923189239867 ) ) ;
#30350=CARTESIAN_POINT ( 'NONE',  ( -27.95245687107223986, 64.57069416759065916, -0.04044903254993292840 ) ) ;
#30352=CARTESIAN_POINT ( 'NONE',  ( -15.01150461594642138, 60.26822916666665009, -26.00068869287340334 ) ) ;
#30371=CARTESIAN_POINT ( 'NONE',  ( -24.22776226481240514, 19.59673583425730925, 13.94119854578937812 ) ) ;
#30376=CARTESIAN_POINT ( 'NONE',  ( -28.02196122052045268, 47.23996500092398065, 7.468012846824790607 ) ) ;
#30377=CARTESIAN_POINT ( 'NONE',  ( 0.04044903255045854962, 36.77305583240936215, 30.02300923189239867 ) ) ;
#30381=CARTESIAN_POINT ( 'NONE',  ( 7.025853678916867295, 60.69232666574269075, 26.06988505166722803 ) ) ;
#30390=CARTESIAN_POINT ( 'NONE',  ( 28.01184896238290278, 33.77083333333333570, -7.505752307973347470 ) ) ;
#30397=CARTESIAN_POINT ( 'NONE',  ( 7.505752307973351023, 65.56770833333332860, 28.01184896238290278 ) ) ;
#30408=CARTESIAN_POINT ( 'NONE',  ( 19.11951029504797006, 29.46836833240935505, 19.06425588902558133 ) ) ;
#30415=CARTESIAN_POINT ( 'NONE',  ( 13.97622843553589966, 50.52864583333333570, -24.20753774853756113 ) ) ;
#30420=CARTESIAN_POINT ( 'NONE',  ( -14.97647472619946285, 20.45611083425730925, -26.02091320914851025 ) ) ;
#30421=CARTESIAN_POINT ( 'NONE',  ( 28.01184896238304134, 61.55729166666666430, 7.505752307972846538 ) ) ;
#30433=CARTESIAN_POINT ( 'NONE',  ( 7.025853678916403666, 34.63579833425730925, -26.06988505166735237 ) ) ;
#30439=CARTESIAN_POINT ( 'NONE',  ( -26.00068869287340334, 59.40885416666666430, 15.01150461594643382 ) ) ;
#30443=CARTESIAN_POINT ( 'NONE',  ( 26.00068869287367335, 41.07552083333331439, 15.01150461594596308 ) ) ;
#30448=CARTESIAN_POINT ( 'NONE',  ( 26.02091320914876960, 53.38763916574269786, 14.97647472619900455 ) ) ;
#30450=CARTESIAN_POINT ( 'NONE',  ( -7.505752307973343918, 56.97395833333333570, -28.01184896238290989 ) ) ;
#30455=CARTESIAN_POINT ( 'NONE',  ( 26.07999730980477437, 26.89583333333332860, -6.988114217768290004 ) ) ;
#30465=CARTESIAN_POINT ( 'NONE',  ( 7.543491769121922985, 22.87982666574268720, 28.00173670424535644 ) ) ;
#30467=CARTESIAN_POINT ( 'NONE',  ( -19.06425588902558133, 37.20274333240935505, 19.11951029504797006 ) ) ;
#30471=CARTESIAN_POINT ( 'NONE',  ( 24.20753774853731244, 64.56510416666667140, -13.97622843553632599 ) ) ;
#30476=CARTESIAN_POINT ( 'NONE',  ( 30.02300923189239512, 37.35156249999997868, -2.619432448724977703E-13 ) ) ;
#30477=CARTESIAN_POINT ( 'NONE',  ( -14.97647472619946285, 30.76861083425731280, -26.02091320914851025 ) ) ;
#30486=CARTESIAN_POINT ( 'NONE',  ( -26.00068869287340334, 14.72135416666666607, 15.01150461594643382 ) ) ;
#30489=CARTESIAN_POINT ( 'NONE',  ( -26.00068869287368756, 32.48177083333332860, -15.01150461594595775 ) ) ;
#30494=CARTESIAN_POINT ( 'NONE',  ( 19.06425588902558133, 42.35899333240935505, -19.11951029504797006 ) ) ;
#30501=CARTESIAN_POINT ( 'NONE',  ( -6.950374756619716266, 48.09934000092398065, -26.09010956794232428 ) ) ;
#30509=CARTESIAN_POINT ( 'NONE',  ( 15.04653450569339945, 60.54909749907603356, 25.98046417659831775 ) ) ;
#30514=CARTESIAN_POINT ( 'NONE',  ( -26.07999730980490583, 39.21354166666666430, -6.988114217767815717 ) ) ;
#30517=CARTESIAN_POINT ( 'NONE',  ( -26.00068869287340334, 38.78385416666665719, 15.01150461594643382 ) ) ;
#30520=CARTESIAN_POINT ( 'NONE',  ( -20.47846945139902175, 58.12538166759063785, -20.53372385742072481 ) ) ;
#30521=CARTESIAN_POINT ( 'NONE',  ( -20.47846945139902175, 10.00038166759064140, -20.53372385742072481 ) ) ;
#30524=CARTESIAN_POINT ( 'NONE',  ( -26.02091320914878025, 17.29388916574268720, -14.97647472619899389 ) ) ;
#30546=CARTESIAN_POINT ( 'NONE',  ( -24.18731323226248264, 16.73215250092398065, -14.01125832528284931 ) ) ;
#30551=CARTESIAN_POINT ( 'NONE',  ( -28.02196122052045268, 50.67746500092398065, 7.468012846824790607 ) ) ;
#30553=CARTESIAN_POINT ( 'NONE',  ( -28.00173670424535644, 40.92670166574268364, 7.543491769121936308 ) ) ;
#30556=CARTESIAN_POINT ( 'NONE',  ( -27.95245687107223986, 65.13243083240935505, 0.04044903255043252877 ) ) ;
#30559=CARTESIAN_POINT ( 'NONE',  ( -7.505752307972844761, 14.29166666666666430, 28.01184896238304134 ) ) ;
#30566=CARTESIAN_POINT ( 'NONE',  ( 28.01184896238304134, 30.61979166666666075, 7.505752307972846538 ) ) ;
#30574=CARTESIAN_POINT ( 'NONE',  ( 30.02300923189239867, 13.28906249999999467, -2.619432448724978208E-13 ) ) ;
#30580=CARTESIAN_POINT ( 'NONE',  ( -14.01125832528328985, 27.89284749907601935, -24.18731323226223040 ) ) ;
#30588=CARTESIAN_POINT ( 'NONE',  ( -6.988114217768288228, 53.53645833333332860, -26.07999730980477437 ) ) ;
#30593=CARTESIAN_POINT ( 'NONE',  ( 26.02091320914851025, 17.87798583425730570, -14.97647472619946463 ) ) ;
#30594=CARTESIAN_POINT ( 'NONE',  ( -15.01150461594595775, 65.99739583333334281, 26.00068869287368756 ) ) ;
#30606=CARTESIAN_POINT ( 'NONE',  ( 27.95245687107223986, 35.35194416759064495, 0.04044903254993640479 ) ) ;
#30613=CARTESIAN_POINT ( 'NONE',  ( -26.00068869287340334, 38.78385416666665719, 15.01150461594643382 ) ) ;
#30618=CARTESIAN_POINT ( 'NONE',  ( 7.543491769121922985, 57.25482666574269075, 28.00173670424535644 ) ) ;
#30620=CARTESIAN_POINT ( 'NONE',  ( -30.02300923189239867, 59.69531250000000711, 2.654126918244514854E-13 ) ) ;
#30625=CARTESIAN_POINT ( 'NONE',  ( -19.09188309203694445, 18.87499999999999645, -19.09188309203661049 ) ) ;
#30639=CARTESIAN_POINT ( 'NONE',  ( -27.95245687107223986, 41.06993083240934794, 0.04044903255043252877 ) ) ;
#30642=CARTESIAN_POINT ( 'NONE',  ( -26.07999730980490583, 66.71354166666665719, -6.988114217767815717 ) ) ;
#30647=CARTESIAN_POINT ( 'NONE',  ( 15.01150461594596308, 33.34114583333332860, -26.00068869287367335 ) ) ;
#30648=CARTESIAN_POINT ( 'NONE',  ( 20.47846945139902530, 32.34413166759064495, 20.53372385742071771 ) ) ;
#30658=CARTESIAN_POINT ( 'NONE',  ( -26.02091320914849959, 60.84673583425731636, 14.97647472619947528 ) ) ;
#30661=CARTESIAN_POINT ( 'NONE',  ( 7.505752307973351023, 34.63020833333332860, 28.01184896238290278 ) ) ;
#30666=CARTESIAN_POINT ( 'NONE',  ( -14.01125832528328985, 55.39284749907604066, -24.18731323226223040 ) ) ;
#30673=CARTESIAN_POINT ( 'NONE',  ( 13.94119854578937812, 49.67486083425730925, 24.22776226481240514 ) ) ;
#30680=CARTESIAN_POINT ( 'NONE',  ( -28.00173670424535644, 68.42670166574269786, 7.543491769121936308 ) ) ;
#30685=CARTESIAN_POINT ( 'NONE',  ( -26.07999730980490583, 35.77604166666666430, -6.988114217767815717 ) ) ;
#30689=CARTESIAN_POINT ( 'NONE',  ( 20.50609665440969565, 36.92187499999999289, -20.50609665441004736 ) ) ;
#30692=CARTESIAN_POINT ( 'NONE',  ( -25.98046417659859486, 57.98215250092397355, -15.04653450569291628 ) ) ;
#30693=CARTESIAN_POINT ( 'NONE',  ( -13.94119854578936923, 58.26861083425732346, -24.22776226481241224 ) ) ;
#30696=CARTESIAN_POINT ( 'NONE',  ( 7.543491769121922985, 19.44232666574268364, 28.00173670424535644 ) ) ;
#30718=CARTESIAN_POINT ( 'NONE',  ( 19.11951029504763611, 17.73475666759064140, -19.06425588902591173 ) ) ;
#30723=CARTESIAN_POINT ( 'NONE',  ( 28.02196122052045268, 45.52121500092397355, -7.468012846824774620 ) ) ;
#30725=CARTESIAN_POINT ( 'NONE',  ( 15.04653450569339945, 39.92409749907602645, 25.98046417659831775 ) ) ;
#30728=CARTESIAN_POINT ( 'NONE',  ( -6.950374756619247307, 67.85378499907602645, 26.09010956794245217 ) ) ;
#30732=CARTESIAN_POINT ( 'NONE',  ( -30.02300923189239512, 15.00781249999999467, 2.654126918244515359E-13 ) ) ;
#30739=CARTESIAN_POINT ( 'NONE',  ( 30.02300923189239512, 44.22656249999997868, -2.619432448724977703E-13 ) ) ;
#30749=CARTESIAN_POINT ( 'NONE',  ( 20.50609665440969565, 16.29687499999999645, -20.50609665441004736 ) ) ;
#30754=CARTESIAN_POINT ( 'NONE',  ( -6.950374756619247307, 26.60378499907601579, 26.09010956794245217 ) ) ;
#30762=CARTESIAN_POINT ( 'NONE',  ( 13.97622843553633665, 48.23697916666665719, 24.20753774853730889 ) ) ;
#30766=CARTESIAN_POINT ( 'NONE',  ( -27.95245687107223276, 32.19531250000000000, 2.498001805406602216E-13 ) ) ;
#30768=CARTESIAN_POINT ( 'NONE',  ( 20.47846945139902530, 18.59413166759064140, 20.53372385742071771 ) ) ;
#30769=CARTESIAN_POINT ( 'NONE',  ( 15.01150461594596308, 64.27864583333332860, -26.00068869287367335 ) ) ;
#30780=CARTESIAN_POINT ( 'NONE',  ( -27.95245687107223986, 33.63319416759063785, -0.04044903254993292840 ) ) ;
#30784=CARTESIAN_POINT ( 'NONE',  ( 26.00068869287367335, 17.01302083333332504, 15.01150461594596308 ) ) ;
#30788=CARTESIAN_POINT ( 'NONE',  ( 28.01184896238304134, 37.49479166666666430, 7.505752307972846538 ) ) ;
#30793=CARTESIAN_POINT ( 'NONE',  ( 28.00173670424535644, 49.52045166574269075, -7.543491769121920321 ) ) ;
#30795=CARTESIAN_POINT ( 'NONE',  ( -26.00068869287368756, 66.85677083333332860, -15.01150461594595775 ) ) ;
#30800=CARTESIAN_POINT ( 'NONE',  ( -26.07999730980490583, 18.58854166666666430, -6.988114217767815717 ) ) ;
#30813=CARTESIAN_POINT ( 'NONE',  ( -27.95245687107223986, 44.50743083240935505, 0.04044903255043252877 ) ) ;
#30818=CARTESIAN_POINT ( 'NONE',  ( -26.07999730980490583, 59.83854166666666430, -6.988114217767815717 ) ) ;
#30822=CARTESIAN_POINT ( 'NONE',  ( 28.01184896238290278, 30.33333333333332860, -7.505752307973347470 ) ) ;
#30823=CARTESIAN_POINT ( 'NONE',  ( 0.04044903254992426173, 34.49256916759064495, -30.02300923189239867 ) ) ;
#30836=CARTESIAN_POINT ( 'NONE',  ( -20.53372385742071771, 60.70350666759063785, 20.47846945139902530 ) ) ;
#30839=CARTESIAN_POINT ( 'NONE',  ( 7.505752307973351023, 38.06770833333332860, 28.01184896238290278 ) ) ;
#30845=CARTESIAN_POINT ( 'NONE',  ( 19.11951029504797006, 50.09336833240935505, 19.06425588902558133 ) ) ;
#30857=CARTESIAN_POINT ( 'NONE',  ( -30.02300923189239867, 68.56993083240934084, 0.04044903255044988294 ) ) ;
#30861=CARTESIAN_POINT ( 'NONE',  ( 27.95245687107222921, 33.91406249999997158, -2.463307335887066074E-13 ) ) ;
#30865=CARTESIAN_POINT ( 'NONE',  ( 7.505752307972854531, 40.07291666666666430, -28.01184896238303423 ) ) ;
#30868=CARTESIAN_POINT ( 'NONE',  ( -7.543491769121417612, 56.97954833425730925, 28.00173670424549499 ) ) ;
#30869=CARTESIAN_POINT ( 'NONE',  ( 7.025853678916403666, 62.13579833425730925, -26.06988505166735237 ) ) ;
#30871=CARTESIAN_POINT ( 'NONE',  ( 14.97647472619900455, 14.71576416574268720, -26.02091320914876960 ) ) ;
#30893=CARTESIAN_POINT ( 'NONE',  ( 26.09010956794232428, 24.89621500092397710, -6.950374756619718042 ) ) ;
#30898=CARTESIAN_POINT ( 'NONE',  ( -28.00173670424549499, 47.52642333425731636, -7.543491769121417612 ) ) ;
#30899=EDGE_CURVE ( 'NONE', #21772, #11003, #18305, .T. ) ;
#30901=CARTESIAN_POINT ( 'NONE',  ( 25.98046417659831775, 35.62722249907602645, -15.04653450569338879 ) ) ;
#30905=CARTESIAN_POINT ( 'NONE',  ( -19.06425588902558133, 68.14024333240935505, 19.11951029504797006 ) ) ;
#30914=CARTESIAN_POINT ( 'NONE',  ( 20.50609665440969565, 43.79687500000000000, -20.50609665441004736 ) ) ;
#30930=CARTESIAN_POINT ( 'NONE',  ( 19.06425588902558133, 28.60899333240935150, -19.11951029504797006 ) ) ;
#30938=CARTESIAN_POINT ( 'NONE',  ( -19.09188309203660694, 48.95312500000000000, 19.09188309203694800 ) ) ;
#30942=CARTESIAN_POINT ( 'NONE',  ( 2.584737979205442066E-13, 31.33593749999999289, 27.95245687107223276 ) ) ;
#30943=CARTESIAN_POINT ( 'NONE',  ( -0.04044903254990864921, 22.46131916759064850, 30.02300923189239867 ) ) ;
#30944=CARTESIAN_POINT ( 'NONE',  ( 7.505752307972854531, 60.69791666666667140, -28.01184896238303423 ) ) ;
#30954=CARTESIAN_POINT ( 'NONE',  ( 26.06988505166735592, 45.80767333425730925, 7.025853678916393896 ) ) ;
#30958=CARTESIAN_POINT ( 'NONE',  ( 28.01184896238290278, 16.58333333333333215, -7.505752307973347470 ) ) ;
#30963=CARTESIAN_POINT ( 'NONE',  ( -28.01184896238290278, 38.92708333333333570, 7.505752307973363457 ) ) ;
#30968=CARTESIAN_POINT ( 'NONE',  ( -20.53372385742107653, 55.24961833240936926, -20.47846945139867003 ) ) ;
#30970=CARTESIAN_POINT ( 'NONE',  ( 15.01150461594643382, 65.42447916666665719, 26.00068869287340334 ) ) ;
#30975=CARTESIAN_POINT ( 'NONE',  ( -24.20753774853756823, 25.60677083333332149, -13.97622843553588723 ) ) ;
#30993=CARTESIAN_POINT ( 'NONE',  ( -19.06425588902591173, 16.87538166759064140, -19.11951029504763611 ) ) ;
#30998=CARTESIAN_POINT ( 'NONE',  ( -15.01150461594595775, 31.62239583333332860, 26.00068869287368756 ) ) ;
#31009=CARTESIAN_POINT ( 'NONE',  ( -25.98046417659859486, 64.85715250092397355, -15.04653450569291628 ) ) ;
#31012=CARTESIAN_POINT ( 'NONE',  ( 20.50609665441005092, 37.78124999999999289, 20.50609665440969209 ) ) ;
#31016=CARTESIAN_POINT ( 'NONE',  ( 7.025853678916867295, 57.25482666574269075, 26.06988505166722803 ) ) ;
#31031=CARTESIAN_POINT ( 'NONE',  ( 0.04044903255044120238, 19.58555583240935860, 27.95245687107223276 ) ) ;
#31036=CARTESIAN_POINT ( 'NONE',  ( -19.09188309203660694, 48.95312500000000000, 19.09188309203694800 ) ) ;
#31040=CARTESIAN_POINT ( 'NONE',  ( -15.01150461594595775, 45.37239583333333570, 26.00068869287368756 ) ) ;
#31043=CARTESIAN_POINT ( 'NONE',  ( 25.98046417659858420, 56.26340250092398065, 15.04653450569292872 ) ) ;
#31044=CARTESIAN_POINT ( 'NONE',  ( -7.025853678916393008, 63.85454833425732346, 26.06988505166735592 ) ) ;
#31047=CARTESIAN_POINT ( 'NONE',  ( 25.98046417659831775, 15.00222249907602112, -15.04653450569338879 ) ) ;
#31053=CARTESIAN_POINT ( 'NONE',  ( -2.584737979205441561E-13, 63.99218749999997868, -30.02300923189239512 ) ) ;
#31065=CARTESIAN_POINT ( 'NONE',  ( -24.22776226481240514, 29.90923583425730925, 13.94119854578937812 ) ) ;
#31072=CARTESIAN_POINT ( 'NONE',  ( -28.02196122052058413, 48.08815999907601935, -7.468012846824272799 ) ) ;
#31076=CARTESIAN_POINT ( 'NONE',  ( 24.22776226481265383, 63.70013916574268364, 13.94119854578893580 ) ) ;
#31080=CARTESIAN_POINT ( 'NONE',  ( -26.00068869287368756, 25.60677083333332149, -15.01150461594595775 ) ) ;
#31086=CARTESIAN_POINT ( 'NONE',  ( 2.740863092043355209E-13, 45.08593750000000711, 30.02300923189239512 ) ) ;
#31087=CARTESIAN_POINT ( 'NONE',  ( 28.01184896238290278, 64.70833333333334281, -7.505752307973347470 ) ) ;
#31101=CARTESIAN_POINT ( 'NONE',  ( -6.950374756619247307, 36.91628499907601224, 26.09010956794245217 ) ) ;
#31110=CARTESIAN_POINT ( 'NONE',  ( -24.20753774853756823, 46.23177083333331439, -13.97622843553588723 ) ) ;
#31114=CARTESIAN_POINT ( 'NONE',  ( 24.20753774853731244, 33.62760416666666430, -13.97622843553633132 ) ) ;
#31116=CARTESIAN_POINT ( 'NONE',  ( 0.04044903254992426173, 24.18006916759064140, -30.02300923189239867 ) ) ;
#31117=CARTESIAN_POINT ( 'NONE',  ( 2.740863092043355209E-13, 65.71093749999997158, 30.02300923189239512 ) ) ;
#31128=CARTESIAN_POINT ( 'NONE',  ( -0.04044903254992426173, 46.52381916759065206, 27.95245687107223276 ) ) ;
#31132=CARTESIAN_POINT ( 'NONE',  ( -26.00068869287368756, 15.29427083333332504, -15.01150461594595775 ) ) ;
#31137=CARTESIAN_POINT ( 'NONE',  ( 26.00068869287367335, 37.63802083333331439, 15.01150461594596308 ) ) ;
#31142=CARTESIAN_POINT ( 'NONE',  ( 15.04653450569339945, 57.11159749907603356, 25.98046417659831775 ) ) ;
#31147=CARTESIAN_POINT ( 'NONE',  ( -13.97622843553632777, 63.70572916666667140, -24.20753774853731599 ) ) ;
#31150=CARTESIAN_POINT ( 'NONE',  ( -19.09188309203694445, 22.31250000000000000, -19.09188309203661049 ) ) ;
#31165=CARTESIAN_POINT ( 'NONE',  ( -0.04044903254992426173, 19.02381916759064495, 27.95245687107223276 ) ) ;
#31170=CARTESIAN_POINT ( 'NONE',  ( 7.505752307973351023, 38.06770833333332860, 28.01184896238290278 ) ) ;
#31182=CARTESIAN_POINT ( 'NONE',  ( 0.04044903254992426173, 61.99256916759065206, -30.02300923189239867 ) ) ;
#31184=CARTESIAN_POINT ( 'NONE',  ( -20.50609665441004736, 42.93750000000000000, -20.50609665440969565 ) ) ;
#31191=CARTESIAN_POINT ( 'NONE',  ( -19.11951029504797006, 51.81211833240936215, -19.06425588902558133 ) ) ;
#31196=CARTESIAN_POINT ( 'NONE',  ( -6.988114217768288228, 12.28645833333333037, -26.07999730980477437 ) ) ;
#31204=CARTESIAN_POINT ( 'NONE',  ( 27.95245687107223276, 22.16368083240936215, -0.04044903255042905932 ) ) ;
#31208=CARTESIAN_POINT ( 'NONE',  ( 26.07999730980490227, 40.93229166666666430, 6.988114217767821046 ) ) ;
#31211=CARTESIAN_POINT ( 'NONE',  ( -20.50609665440969209, 45.51562500000000000, 20.50609665441005092 ) ) ;
#31213=CARTESIAN_POINT ( 'NONE',  ( -7.505752307973343918, 15.72395833333332860, -28.01184896238290989 ) ) ;
#31214=CARTESIAN_POINT ( 'NONE',  ( 28.00173670424549499, 18.30767333425730214, 7.543491769121417612 ) ) ;
#31235=CARTESIAN_POINT ( 'NONE',  ( -13.94119854578936923, 27.33111083425731280, -24.22776226481241224 ) ) ;
#31241=CARTESIAN_POINT ( 'NONE',  ( 0.04044903255045854962, 50.52305583240934794, 30.02300923189239867 ) ) ;
#31245=CARTESIAN_POINT ( 'NONE',  ( -6.988114217768288228, 19.16145833333332860, -26.07999730980477437 ) ) ;
#31248=CARTESIAN_POINT ( 'NONE',  ( 30.02300923189239512, 20.16406249999999645, -2.619432448724977703E-13 ) ) ;
#31254=CARTESIAN_POINT ( 'NONE',  ( -20.50609665440969209, 42.07812499999999289, 20.50609665441005092 ) ) ;
#31255=CARTESIAN_POINT ( 'NONE',  ( -15.01150461594595775, 62.55989583333332860, 26.00068869287368756 ) ) ;
#31264=CARTESIAN_POINT ( 'NONE',  ( -28.01184896238290278, 14.86458333333333037, 7.505752307973363457 ) ) ;
#31270=CARTESIAN_POINT ( 'NONE',  ( 27.95245687107223276, 35.91368083240935505, -0.04044903255042905932 ) ) ;
#31278=CARTESIAN_POINT ( 'NONE',  ( 19.09188309203694800, 61.84374999999998579, 19.09188309203660694 ) ) ;
#31282=CARTESIAN_POINT ( 'NONE',  ( 13.97622843553589966, 36.77864583333332860, -24.20753774853756113 ) ) ;
#31283=CARTESIAN_POINT ( 'NONE',  ( 0.04044903254992426173, 27.61756916759064140, -30.02300923189239867 ) ) ;
#31284=CARTESIAN_POINT ( 'NONE',  ( -20.47846945139866648, 20.01524333240935505, 20.53372385742108008 ) ) ;
#31294=CARTESIAN_POINT ( 'NONE',  ( 19.06425588902592239, 42.65663166759063785, 19.11951029504763611 ) ) ;
#31298=CARTESIAN_POINT ( 'NONE',  ( 7.505752307973351023, 14.00520833333333215, 28.01184896238290278 ) ) ;
#31302=CARTESIAN_POINT ( 'NONE',  ( -15.01150461594595775, 52.24739583333332860, 26.00068869287368756 ) ) ;
#31307=CARTESIAN_POINT ( 'NONE',  ( -20.47846945139866648, 61.26524333240935505, 20.53372385742108008 ) ) ;
#31312=CARTESIAN_POINT ( 'NONE',  ( 24.20753774853731244, 64.56510416666667140, -13.97622843553633132 ) ) ;
#31317=CARTESIAN_POINT ( 'NONE',  ( -6.988114217768288228, 32.91145833333332860, -26.07999730980477437 ) ) ;
#31324=CARTESIAN_POINT ( 'NONE',  ( 0.04044903254993986036, 48.24256916759064495, -27.95245687107223986 ) ) ;
#31335=CARTESIAN_POINT ( 'NONE',  ( -19.06425588902591173, 13.43788166759064140, -19.11951029504763611 ) ) ;
#31339=CARTESIAN_POINT ( 'NONE',  ( -7.505752307972844761, 45.22916666666665719, 28.01184896238304134 ) ) ;
#31343=CARTESIAN_POINT ( 'NONE',  ( 7.505752307972854531, 22.88541666666666430, -28.01184896238303423 ) ) ;
#31349=CARTESIAN_POINT ( 'NONE',  ( 30.02300923189239867, 35.91368083240935505, -0.04044903255044467877 ) ) ;
#31351=CARTESIAN_POINT ( 'NONE',  ( -26.00068869287340334, 35.34635416666666430, 15.01150461594643559 ) ) ;
#31358=CARTESIAN_POINT ( 'NONE',  ( -13.94119854578892514, 50.80951416574269075, 24.22776226481266448 ) ) ;
#31371=CARTESIAN_POINT ( 'NONE',  ( -19.11951029504797006, 17.43711833240935505, -19.06425588902558133 ) ) ;
#31375=CARTESIAN_POINT ( 'NONE',  ( -26.07999730980490583, 42.65104166666666430, -6.988114217767815717 ) ) ;
#31379=CARTESIAN_POINT ( 'NONE',  ( -15.01150461594595775, 48.80989583333332860, 26.00068869287368756 ) ) ;
#31381=CARTESIAN_POINT ( 'NONE',  ( -20.50609665441004736, 15.43749999999999645, -20.50609665440969565 ) ) ;
#31382=CARTESIAN_POINT ( 'NONE',  ( 14.97647472619947351, 11.86236083425730925, 26.02091320914850314 ) ) ;
#31390=CARTESIAN_POINT ( 'NONE',  ( 26.00068869287340334, 64.56510416666667140, -15.01150461594642316 ) ) ;
#31404=CARTESIAN_POINT ( 'NONE',  ( 14.01125832528286352, 27.90402750092397355, -24.18731323226246843 ) ) ;
#31412=CARTESIAN_POINT ( 'NONE',  ( 28.00173670424535644, 49.52045166574269075, -7.543491769121920321 ) ) ;
#31415=FILL_AREA_STYLE_COLOUR ( '', #17819 ) ;
#31416=CARTESIAN_POINT ( 'NONE',  ( -6.988114217767819270, 21.16666666666666430, 26.07999730980490583 ) ) ;
#31419=CARTESIAN_POINT ( 'NONE',  ( 7.505752307973351023, 20.88020833333333215, 28.01184896238290278 ) ) ;
#31423=CARTESIAN_POINT ( 'NONE',  ( -20.47846945139902175, 44.37538166759063785, -20.53372385742072481 ) ) ;
#31425=CARTESIAN_POINT ( 'NONE',  ( -28.01184896238304134, 56.40104166666666430, -7.505752307972844761 ) ) ;
#31436=CARTESIAN_POINT ( 'NONE',  ( -15.01150461594595775, 24.74739583333332860, 26.00068869287368756 ) ) ;
#31441=CARTESIAN_POINT ( 'NONE',  ( -24.18731323226221974, 30.47097249907602290, 14.01125832528330406 ) ) ;
#31448=CARTESIAN_POINT ( 'NONE',  ( 2.584737979205441561E-13, 62.27343749999999289, 27.95245687107222921 ) ) ;
#31452=CARTESIAN_POINT ( 'NONE',  ( -27.95245687107223276, 39.07031249999998579, 2.498001805406602216E-13 ) ) ;
#31453=CARTESIAN_POINT ( 'NONE',  ( -7.543491769121417612, 26.04204833425729859, 28.00173670424549499 ) ) ;
#31454=CARTESIAN_POINT ( 'NONE',  ( -0.04044903255044120238, 17.86680583240935860, -30.02300923189239867 ) ) ;
#31459=CARTESIAN_POINT ( 'NONE',  ( 19.06425588902558133, 45.79649333240935505, -19.11951029504797006 ) ) ;
#31466=CARTESIAN_POINT ( 'NONE',  ( -6.950374756619716266, 37.78684000092396644, -26.09010956794232428 ) ) ;
#31471=CARTESIAN_POINT ( 'NONE',  ( 2.740863092043355209E-13, 17.58593749999999645, 30.02300923189239512 ) ) ;
#31475=CARTESIAN_POINT ( 'NONE',  ( 28.01184896238304134, 44.36979166666666430, 7.505752307972846538 ) ) ;
#31481=CARTESIAN_POINT ( 'NONE',  ( -28.00173670424535644, 64.98920166574268364, 7.543491769121936308 ) ) ;
#31486=CARTESIAN_POINT ( 'NONE',  ( 19.09188309203694800, 65.28125000000000000, 19.09188309203660694 ) ) ;
#31489=CARTESIAN_POINT ( 'NONE',  ( -6.988114217767819270, 28.04166666666666075, 26.07999730980490583 ) ) ;
#31495=CARTESIAN_POINT ( 'NONE',  ( -26.06988505166735237, 57.83892333425730214, -7.025853678916388567 ) ) ;
#31507=CARTESIAN_POINT ( 'NONE',  ( -19.11951029504763611, 12.57850666759064140, 19.06425588902592239 ) ) ;
#31511=CARTESIAN_POINT ( 'NONE',  ( -26.00068869287340334, 42.22135416666666430, 15.01150461594643382 ) ) ;
#31515=CARTESIAN_POINT ( 'NONE',  ( 28.01184896238304134, 20.30729166666666430, 7.505752307972846538 ) ) ;
#31521=CARTESIAN_POINT ( 'NONE',  ( -7.468012846824272799, 30.04128499907601224, 28.02196122052058413 ) ) ;
#31523=CARTESIAN_POINT ( 'NONE',  ( -15.01150461594642316, 43.08072916666666430, -26.00068869287341045 ) ) ;
#31528=CARTESIAN_POINT ( 'NONE',  ( -19.11951029504797006, 65.56211833240934084, -19.06425588902558133 ) ) ;
#31535=CARTESIAN_POINT ( 'NONE',  ( 24.20753774853756113, 17.01302083333332504, 13.97622843553589789 ) ) ;
#31540=CARTESIAN_POINT ( 'NONE',  ( -6.950374756619247307, 16.29128499907601579, 26.09010956794245217 ) ) ;
#31543=CARTESIAN_POINT ( 'NONE',  ( -13.97622843553588901, 41.93489583333333570, 24.20753774853756823 ) ) ;
#31547=CARTESIAN_POINT ( 'NONE',  ( -30.02300923189239867, 64.57069416759065916, -0.04044903254991731589 ) ) ;
#31548=CARTESIAN_POINT ( 'NONE',  ( 28.02196122052045268, 14.58371500092397710, -7.468012846824774620 ) ) ;
#31567=CARTESIAN_POINT ( 'NONE',  ( 13.94119854578937812, 32.48736083425731636, 24.22776226481240514 ) ) ;
#31574=CARTESIAN_POINT ( 'NONE',  ( 28.00173670424535644, 46.08295166574269075, -7.543491769121920321 ) ) ;
#31578=CARTESIAN_POINT ( 'NONE',  ( 13.97622843553589966, 19.59114583333332149, -24.20753774853756113 ) ) ;
#31581=CARTESIAN_POINT ( 'NONE',  ( -28.01184896238290278, 25.17708333333332860, 7.505752307973363457 ) ) ;
#31585=CARTESIAN_POINT ( 'NONE',  ( -25.98046417659859486, 44.23215250092398065, -15.04653450569291628 ) ) ;
#31588=CARTESIAN_POINT ( 'NONE',  ( -26.00068869287340334, 49.09635416666665719, 15.01150461594643382 ) ) ;
#31599=CARTESIAN_POINT ( 'NONE',  ( 2.740863092043355209E-13, 17.58593749999999645, 30.02300923189239867 ) ) ;
#31604=CARTESIAN_POINT ( 'NONE',  ( 6.950374756619257965, 35.19753499907601935, -26.09010956794244507 ) ) ;
#31612=CARTESIAN_POINT ( 'NONE',  ( -26.07999730980477437, 59.55208333333332149, 6.988114217768305103 ) ) ;
#31616=CARTESIAN_POINT ( 'NONE',  ( 27.95245687107223276, 44.22656249999999289, -2.463307335887066074E-13 ) ) ;
#31617=CARTESIAN_POINT ( 'NONE',  ( -7.543491769121417612, 32.91704833425729504, 28.00173670424549499 ) ) ;
#31618=CARTESIAN_POINT ( 'NONE',  ( -0.04044903255044120238, 21.30430583240935860, -30.02300923189239867 ) ) ;
#31622=CARTESIAN_POINT ( 'NONE',  ( -26.09010956794245217, 48.08815999907601935, -6.950374756619243755 ) ) ;
#31628=CARTESIAN_POINT ( 'NONE',  ( 27.95245687107223986, 55.97694416759064495, 0.04044903254993640479 ) ) ;
#31632=CARTESIAN_POINT ( 'NONE',  ( -20.50609665441004736, 22.31250000000000000, -20.50609665440969565 ) ) ;
#31636=CARTESIAN_POINT ( 'NONE',  ( 28.01184896238304134, 47.80729166666666430, 7.505752307972846538 ) ) ;
#31643=CARTESIAN_POINT ( 'NONE',  ( 14.97647472619900455, 62.84076416574269786, -26.02091320914876960 ) ) ;
#31648=CARTESIAN_POINT ( 'NONE',  ( -24.20753774853730889, 59.40885416666666430, 13.97622843553634020 ) ) ;
#31651=CARTESIAN_POINT ( 'NONE',  ( 13.97622843553589966, 33.34114583333332860, -24.20753774853756113 ) ) ;
#31658=CARTESIAN_POINT ( 'NONE',  ( -26.06988505166735237, 61.27642333425730925, -7.025853678916388567 ) ) ;
#31670=CARTESIAN_POINT ( 'NONE',  ( 24.22776226481241224, 11.00298583425731103, -13.94119854578936923 ) ) ;
#31675=CARTESIAN_POINT ( 'NONE',  ( -28.01184896238304134, 39.21354166666666430, -7.505752307972844761 ) ) ;
#31679=CARTESIAN_POINT ( 'NONE',  ( 2.740863092043355209E-13, 21.02343749999999645, 30.02300923189239512 ) ) ;
#31685=CARTESIAN_POINT ( 'NONE',  ( 0.04044903255045854962, 33.33555583240935505, 30.02300923189239867 ) ) ;
#31687=CARTESIAN_POINT ( 'NONE',  ( 2.740863092043355209E-13, 51.96093750000000000, 30.02300923189239867 ) ) ;
#31694=CARTESIAN_POINT ( 'NONE',  ( -24.18731323226221974, 64.84597249907602645, 14.01125832528330406 ) ) ;
#31701=CARTESIAN_POINT ( 'NONE',  ( -6.988114217768288228, 19.16145833333332860, -26.07999730980477437 ) ) ;
#31708=CARTESIAN_POINT ( 'NONE',  ( -6.950374756619247307, 23.16628499907601579, 26.09010956794245217 ) ) ;
#31712=CARTESIAN_POINT ( 'NONE',  ( 27.95245687107222921, 44.22656249999997868, -2.463307335887066074E-13 ) ) ;
#31716=CARTESIAN_POINT ( 'NONE',  ( 26.00068869287340334, 13.00260416666666430, -15.01150461594642316 ) ) ;
#31717=CARTESIAN_POINT ( 'NONE',  ( 28.02196122052045268, 18.02121500092397710, -7.468012846824774620 ) ) ;
#31737=CARTESIAN_POINT ( 'NONE',  ( -26.09010956794232428, 33.48996500092397355, 6.950374756619732253 ) ) ;
#31744=CARTESIAN_POINT ( 'NONE',  ( 0.04044903255045854962, 43.64805583240936215, 30.02300923189239867 ) ) ;
#31747=CARTESIAN_POINT ( 'NONE',  ( -27.95245687107222921, 18.44531249999999645, 2.498001805406602216E-13 ) ) ;
#31749=CARTESIAN_POINT ( 'NONE',  ( 20.50609665441005092, 17.15624999999999645, 20.50609665440969209 ) ) ;
#31754=CARTESIAN_POINT ( 'NONE',  ( -15.04653450569291984, 39.93527750092397355, 25.98046417659859486 ) ) ;
#31756=CARTESIAN_POINT ( 'NONE',  ( 28.01184896238304134, 54.68229166666665719, 7.505752307972846538 ) ) ;
#31765=CARTESIAN_POINT ( 'NONE',  ( 15.01150461594643382, 20.73697916666666075, 26.00068869287340334 ) ) ;
#31770=CARTESIAN_POINT ( 'NONE',  ( -0.04044903255042732459, 38.49180583240935505, -27.95245687107223986 ) ) ;
#31777=CARTESIAN_POINT ( 'NONE',  ( -24.20753774853756823, 59.98177083333332149, -13.97622843553588723 ) ) ;
#31781=CARTESIAN_POINT ( 'NONE',  ( 13.97622843553589966, 43.65364583333332860, -24.20753774853756113 ) ) ;
#31782=CARTESIAN_POINT ( 'NONE',  ( 30.02300923189239867, 31.91444416759064495, 0.04044903254992252006 ) ) ;
#31784=CARTESIAN_POINT ( 'NONE',  ( 20.47846945139867003, 21.73399333240935505, -20.53372385742107653 ) ) ;
#31788=CARTESIAN_POINT ( 'NONE',  ( 13.94119854578893580, 42.21576416574269075, -24.22776226481265383 ) ) ;
#31795=CARTESIAN_POINT ( 'NONE',  ( -0.04044903254992426173, 49.96131916759065206, 27.95245687107223276 ) ) ;
#31800=CARTESIAN_POINT ( 'NONE',  ( 7.505752307973351023, 20.88020833333333215, 28.01184896238290278 ) ) ;
#31804=CARTESIAN_POINT ( 'NONE',  ( 15.01150461594596308, 47.09114583333332860, -26.00068869287367335 ) ) ;
#31810=CARTESIAN_POINT ( 'NONE',  ( -7.468012846824272799, 57.54128499907602645, 28.02196122052058413 ) ) ;
#31815=CARTESIAN_POINT ( 'NONE',  ( -13.97622843553588901, 59.12239583333333570, 24.20753774853756823 ) ) ;
#31818=CARTESIAN_POINT ( 'NONE',  ( -27.95245687107222921, 35.63281249999998579, 2.498001805406602216E-13 ) ) ;
#31824=CARTESIAN_POINT ( 'NONE',  ( -6.950374756619716266, 54.97434000092398065, -26.09010956794232428 ) ) ;
#31835=CARTESIAN_POINT ( 'NONE',  ( 24.22776226481241224, 24.75298583425730925, -13.94119854578936923 ) ) ;
#31841=CARTESIAN_POINT ( 'NONE',  ( 28.01184896238290278, 40.64583333333332860, -7.505752307973347470 ) ) ;
#31845=CARTESIAN_POINT ( 'NONE',  ( -28.01184896238290278, 21.73958333333332860, 7.505752307973363457 ) ) ;
#31851=CARTESIAN_POINT ( 'NONE',  ( 7.468012846824281681, 31.76003499907602290, -28.02196122052058058 ) ) ;
#31854=CARTESIAN_POINT ( 'NONE',  ( 26.00068869287341045, 47.37760416666666430, -15.01150461594642493 ) ) ;
#31857=CARTESIAN_POINT ( 'NONE',  ( 27.95245687107223276, 59.97618083240934794, -0.04044903255042905932 ) ) ;
#31863=CARTESIAN_POINT ( 'NONE',  ( 24.20753774853756113, 23.88802083333332504, 13.97622843553589789 ) ) ;
#31869=CARTESIAN_POINT ( 'NONE',  ( 24.22776226481265383, 29.32513916574269075, 13.94119854578893580 ) ) ;
#31873=CARTESIAN_POINT ( 'NONE',  ( -26.07999730980477437, 49.23958333333332860, 6.988114217768305103 ) ) ;
#31878=CARTESIAN_POINT ( 'NONE',  ( 7.505752307973351023, 17.44270833333333215, 28.01184896238290278 ) ) ;
#31879=CARTESIAN_POINT ( 'NONE',  ( 14.97647472619947351, 15.29986083425731280, 26.02091320914850314 ) ) ;
#31900=CARTESIAN_POINT ( 'NONE',  ( -26.06988505166735237, 40.65142333425730214, -7.025853678916388567 ) ) ;
#31908=CARTESIAN_POINT ( 'NONE',  ( 15.04653450569339945, 57.11159749907603356, 25.98046417659831775 ) ) ;
#31913=CARTESIAN_POINT ( 'NONE',  ( -13.97622843553588901, 14.43489583333332682, 24.20753774853756823 ) ) ;
#31917=CARTESIAN_POINT ( 'NONE',  ( 7.505752307972854531, 33.19791666666665719, -28.01184896238303423 ) ) ;
#31921=CARTESIAN_POINT ( 'NONE',  ( 30.02300923189239867, 38.78944416759064495, 0.04044903254992252006 ) ) ;
#31923=CARTESIAN_POINT ( 'NONE',  ( -20.50609665440969209, 48.95312500000000000, 20.50609665441005092 ) ) ;
#31933=CARTESIAN_POINT ( 'NONE',  ( -7.505752307972844761, 17.72916666666666430, 28.01184896238304134 ) ) ;
#31945=CARTESIAN_POINT ( 'NONE',  ( 24.20753774853731244, 61.12760416666665719, -13.97622843553632599 ) ) ;
#31949=CARTESIAN_POINT ( 'NONE',  ( 6.988114217767829928, 40.07291666666666430, -26.07999730980489872 ) ) ;
#31950=CARTESIAN_POINT ( 'NONE',  ( -28.02196122052045268, 33.48996500092397355, 7.468012846824790607 ) ) ;
#31952=CARTESIAN_POINT ( 'NONE',  ( 0.04044903255045854962, 23.02305583240935860, 30.02300923189239867 ) ) ;
#31956=CARTESIAN_POINT ( 'NONE',  ( 24.22776226481265383, 49.95013916574269786, 13.94119854578893580 ) ) ;
#31962=CARTESIAN_POINT ( 'NONE',  ( -19.11951029504763611, 50.39100666759063785, 19.06425588902592239 ) ) ;
#31968=CARTESIAN_POINT ( 'NONE',  ( -7.505752307973343918, 29.47395833333332860, -28.01184896238290989 ) ) ;
#31971=CARTESIAN_POINT ( 'NONE',  ( 15.01150461594596308, 50.52864583333333570, -26.00068869287367335 ) ) ;
#31977=CARTESIAN_POINT ( 'NONE',  ( 20.47846945139867003, 66.42149333240935505, -20.53372385742107653 ) ) ;
#31984=CARTESIAN_POINT ( 'NONE',  ( -19.09188309203694445, 36.06250000000000000, -19.09188309203661049 ) ) ;
#31990=CARTESIAN_POINT ( 'NONE',  ( -19.11951029504763611, 53.82850666759064495, 19.06425588902592239 ) ) ;
#32002=CARTESIAN_POINT ( 'NONE',  ( 6.950374756619721595, 25.75559000092397710, 26.09010956794232428 ) ) ;
#32008=CARTESIAN_POINT ( 'NONE',  ( 28.01184896238290278, 47.52083333333332860, -7.505752307973347470 ) ) ;
#32012=CARTESIAN_POINT ( 'NONE',  ( 15.01150461594643204, 17.29947916666666430, 26.00068869287340334 ) ) ;
#32019=CARTESIAN_POINT ( 'NONE',  ( -26.02091320914878025, 37.91888916574269075, -14.97647472619899389 ) ) ;
#32021=CARTESIAN_POINT ( 'NONE',  ( -28.01184896238290278, 45.80208333333333570, 7.505752307973363457 ) ) ;
#32025=CARTESIAN_POINT ( 'NONE',  ( -13.94119854578892514, 57.68451416574269075, 24.22776226481266448 ) ) ;
#32031=CARTESIAN_POINT ( 'NONE',  ( 26.07999730980477437, 23.45833333333333215, -6.988114217768290004 ) ) ;
#32038=CARTESIAN_POINT ( 'NONE',  ( -7.025853678916861966, 31.47357666574268364, -26.06988505166722803 ) ) ;
#32041=CARTESIAN_POINT ( 'NONE',  ( -13.97622843553588901, 55.68489583333332860, 24.20753774853756823 ) ) ;
#32045=CARTESIAN_POINT ( 'NONE',  ( 2.740863092043355209E-13, 21.02343749999999645, 30.02300923189239512 ) ) ;
#32046=CARTESIAN_POINT ( 'NONE',  ( 30.02300923189239867, 25.03944416759064495, 0.04044903254992252006 ) ) ;
#32067=CARTESIAN_POINT ( 'NONE',  ( -13.94119854578936923, 41.08111083425730214, -24.22776226481241224 ) ) ;
#32077=CARTESIAN_POINT ( 'NONE',  ( -20.53372385742107653, 58.68711833240935505, -20.47846945139867003 ) ) ;
#32081=( NAMED_UNIT ( * ) PLANE_ANGLE_UNIT ( ) SI_UNIT ( $, .RADIAN. ) );
#32082=CARTESIAN_POINT ( 'NONE',  ( 13.97622843553633665, 27.61197916666666430, 24.20753774853730889 ) ) ;
#32085=CARTESIAN_POINT ( 'NONE',  ( 28.01184896238290278, 30.33333333333332860, -7.505752307973347470 ) ) ;
#32088=CARTESIAN_POINT ( 'NONE',  ( 28.00173670424549499, 52.68267333425730214, 7.543491769121417612 ) ) ;
#32090=CARTESIAN_POINT ( 'NONE',  ( -7.505752307972844761, 52.10416666666666430, 28.01184896238304134 ) ) ;
#32108=CARTESIAN_POINT ( 'NONE',  ( 24.18731323226247554, 11.57590250092397355, 14.01125832528285997 ) ) ;
#32115=CARTESIAN_POINT ( 'NONE',  ( 6.988114217767829928, 53.82291666666666430, -26.07999730980489872 ) ) ;
#32117=CARTESIAN_POINT ( 'NONE',  ( -0.04044903254990864921, 43.08631916759065916, 30.02300923189239867 ) ) ;
#32119=CARTESIAN_POINT ( 'NONE',  ( -28.02196122052058413, 27.46315999907601935, -7.468012846824272799 ) ) ;
#32123=CARTESIAN_POINT ( 'NONE',  ( -0.04044903255042732459, 59.11680583240937636, -27.95245687107223986 ) ) ;
#32130=CARTESIAN_POINT ( 'NONE',  ( 13.94119854578937812, 53.11236083425731636, 24.22776226481240514 ) ) ;
#32134=CARTESIAN_POINT ( 'NONE',  ( 26.00068869287367335, 23.88802083333331794, 15.01150461594596308 ) ) ;
#32138=CARTESIAN_POINT ( 'NONE',  ( 20.50609665440969565, 54.10937499999999289, -20.50609665441004736 ) ) ;
#32145=CARTESIAN_POINT ( 'NONE',  ( -26.06988505166722803, 20.30170166574269075, 7.025853678916877953 ) ) ;
#32153=CARTESIAN_POINT ( 'NONE',  ( 26.07999730980490227, 37.49479166666666430, 6.988114217767821046 ) ) ;
#32159=CARTESIAN_POINT ( 'NONE',  ( -6.950374756619716266, 61.84934000092397355, -26.09010956794232428 ) ) ;
#32161=CARTESIAN_POINT ( 'NONE',  ( 30.02300923189239512, 54.53906249999998579, -2.619432448724977703E-13 ) ) ;
#32173=CARTESIAN_POINT ( 'NONE',  ( -6.950374756619716266, 27.47434000092397000, -26.09010956794232428 ) ) ;
#32178=CARTESIAN_POINT ( 'NONE',  ( 26.00068869287340334, 47.37760416666666430, -15.01150461594642316 ) ) ;
#32182=CARTESIAN_POINT ( 'NONE',  ( 20.50609665440969565, 30.04687500000000000, -20.50609665441004736 ) ) ;
#32186=MANIFOLD_SOLID_BREP ( 'Sweep1', #19408 ) ;
#32189=CARTESIAN_POINT ( 'NONE',  ( -14.97647472619899389, 40.49701416574269786, 26.02091320914878025 ) ) ;
#32191=CARTESIAN_POINT ( 'NONE',  ( -26.00068869287368756, 46.23177083333332149, -15.01150461594595775 ) ) ;
#32194=CARTESIAN_POINT ( 'NONE',  ( -14.01125832528328985, 65.70534749907602645, -24.18731323226223040 ) ) ;
#32201=CARTESIAN_POINT ( 'NONE',  ( -2.428612866367529427E-13, 22.74218749999999645, -27.95245687107223276 ) ) ;
#32208=CARTESIAN_POINT ( 'NONE',  ( 26.09010956794244507, 29.18190999907601579, 6.950374756619249084 ) ) ;
#32212=CARTESIAN_POINT ( 'NONE',  ( 24.20753774853756113, 51.38802083333332149, 13.97622843553589789 ) ) ;
#32219=CARTESIAN_POINT ( 'NONE',  ( -26.00068869287340334, 25.03385416666666785, 15.01150461594643382 ) ) ;
#32220=CARTESIAN_POINT ( 'NONE',  ( 25.98046417659858420, 25.32590250092397710, 15.04653450569292872 ) ) ;
#32229=CARTESIAN_POINT ( 'NONE',  ( 7.468012846824777284, 53.25559000092396644, 28.02196122052045268 ) ) ;
#32239=CARTESIAN_POINT ( 'NONE',  ( -24.22776226481240514, 36.78423583425730214, 13.94119854578937812 ) ) ;
#32248=CARTESIAN_POINT ( 'NONE',  ( 7.543491769121922985, 53.81732666574268364, 28.00173670424535644 ) ) ;
#32251=CARTESIAN_POINT ( 'NONE',  ( 13.97622843553589966, 29.90364583333332504, -24.20753774853756113 ) ) ;
#32253=CARTESIAN_POINT ( 'NONE',  ( -28.01184896238290278, 32.05208333333332860, 7.505752307973363457 ) ) ;
#32256=CARTESIAN_POINT ( 'NONE',  ( 15.04653450569292872, 51.96652750092398065, -25.98046417659857710 ) ) ;
#32258=CARTESIAN_POINT ( 'NONE',  ( 7.505752307972854531, 60.69791666666667140, -28.01184896238303423 ) ) ;
#32277=CARTESIAN_POINT ( 'NONE',  ( -19.11951029504763611, 16.01600666759064140, 19.06425588902592239 ) ) ;
#32282=CARTESIAN_POINT ( 'NONE',  ( -26.07999730980490583, 52.96354166666666430, -6.988114217767815717 ) ) ;
#32283=CARTESIAN_POINT ( 'NONE',  ( 20.47846945139902530, 39.21913166759063785, 20.53372385742071771 ) ) ;
#32284=CARTESIAN_POINT ( 'NONE',  ( 20.47846945139867003, 32.04649333240934084, -20.53372385742107653 ) ) ;
#32287=CARTESIAN_POINT ( 'NONE',  ( -13.94119854578892514, 57.68451416574269075, 24.22776226481266448 ) ) ;
#32293=CARTESIAN_POINT ( 'NONE',  ( -14.01125832528285109, 50.24777750092398065, 24.18731323226248264 ) ) ;
#32297=CARTESIAN_POINT ( 'NONE',  ( -28.01184896238304134, 25.46354166666666430, -7.505752307972844761 ) ) ;
#32303=CARTESIAN_POINT ( 'NONE',  ( -15.01150461594595775, 59.12239583333333570, 26.00068869287368756 ) ) ;
#32310=CARTESIAN_POINT ( 'NONE',  ( 26.09010956794244507, 18.86940999907601935, 6.950374756619249084 ) ) ;
#32319=CARTESIAN_POINT ( 'NONE',  ( 26.07999730980477437, 44.08333333333332860, -6.988114217768290004 ) ) ;
#32325=CARTESIAN_POINT ( 'NONE',  ( -15.04653450569291984, 12.43527750092397532, 25.98046417659859486 ) ) ;
#32326=CARTESIAN_POINT ( 'NONE',  ( 2.740863092043355209E-13, 55.39843749999999289, 30.02300923189239512 ) ) ;
#32337=CARTESIAN_POINT ( 'NONE',  ( 0.04044903254993986036, 24.18006916759064140, -27.95245687107223986 ) ) ;
#32341=VERTEX_POINT ( 'NONE', #25554 ) ;
#32342=CARTESIAN_POINT ( 'NONE',  ( 30.02300923189239512, 54.53906249999998579, -2.619432448724977703E-13 ) ) ;
#32346=CARTESIAN_POINT ( 'NONE',  ( -26.00068869287340334, 28.47135416666666075, 15.01150461594643382 ) ) ;
#32353=CARTESIAN_POINT ( 'NONE',  ( 7.543491769121922985, 46.94232666574269075, 28.00173670424535644 ) ) ;
#32355=CARTESIAN_POINT ( 'NONE',  ( -30.02300923189239867, 45.94531249999998579, 2.654126918244514854E-13 ) ) ;
#32358=CARTESIAN_POINT ( 'NONE',  ( 19.09188309203661049, 16.29687499999999645, -19.09188309203694445 ) ) ;
#32364=CARTESIAN_POINT ( 'NONE',  ( 26.07999730980477437, 20.02083333333332860, -6.988114217768290004 ) ) ;
#32371=CARTESIAN_POINT ( 'NONE',  ( 26.06988505166722803, 25.45795166574268364, -7.025853678916862854 ) ) ;
#32375=CARTESIAN_POINT ( 'NONE',  ( -26.07999730980477437, 56.11458333333332860, 6.988114217768305103 ) ) ;
#32380=CARTESIAN_POINT ( 'NONE',  ( 7.505752307972854531, 26.32291666666666075, -28.01184896238303423 ) ) ;
#32381=CARTESIAN_POINT ( 'NONE',  ( -0.04044903254990864921, 22.46131916759064850, 30.02300923189239867 ) ) ;
#32391=CARTESIAN_POINT ( 'NONE',  ( 7.468012846824777284, 60.13059000092398065, 28.02196122052045268 ) ) ;
#32397=CARTESIAN_POINT ( 'NONE',  ( -13.94119854578892514, 40.49701416574269786, 24.22776226481266448 ) ) ;
#32402=CARTESIAN_POINT ( 'NONE',  ( -7.025853678916393008, 39.79204833425731636, 26.06988505166735592 ) ) ;
#32410=CARTESIAN_POINT ( 'NONE',  ( -30.02300923189239867, 51.38243083240936215, 0.04044903255044988294 ) ) ;
#32415=CARTESIAN_POINT ( 'NONE',  ( -19.09188309203660694, 28.32812499999999645, 19.09188309203694800 ) ) ;
#32417=CARTESIAN_POINT ( 'NONE',  ( -26.00068869287340334, 28.47135416666666075, 15.01150461594643382 ) ) ;
#32420=CARTESIAN_POINT ( 'NONE',  ( 20.47846945139902530, 46.09413166759064495, 20.53372385742071771 ) ) ;
#32422=CARTESIAN_POINT ( 'NONE',  ( 7.505752307972854531, 64.13541666666667140, -28.01184896238303423 ) ) ;
#32442=CARTESIAN_POINT ( 'NONE',  ( 2.584737979205441561E-13, 65.71093749999997158, 27.95245687107222921 ) ) ;
#32447=CARTESIAN_POINT ( 'NONE',  ( 6.988114217768294445, 48.38020833333332860, 26.07999730980477437 ) ) ;
#32448=CARTESIAN_POINT ( 'NONE',  ( 15.04653450569292872, 41.65402750092398065, -25.98046417659857710 ) ) ;
#32449=CARTESIAN_POINT ( 'NONE',  ( -7.543491769121917656, 28.03607666574268364, -28.00173670424536354 ) ) ;
#32452=CARTESIAN_POINT ( 'NONE',  ( -24.18731323226221974, 57.97097249907601935, 14.01125832528330406 ) ) ;
#32461=CARTESIAN_POINT ( 'NONE',  ( -2.584737979205441561E-13, 29.61718749999999645, -30.02300923189239512 ) ) ;
#32465=CARTESIAN_POINT ( 'NONE',  ( -15.01150461594642138, 56.83072916666665009, -26.00068869287340334 ) ) ;
#32472=CARTESIAN_POINT ( 'NONE',  ( -0.04044903255042732459, 14.42930583240935505, -27.95245687107223986 ) ) ;
#32480=CARTESIAN_POINT ( 'NONE',  ( -26.07999730980490583, 39.21354166666666430, -6.988114217767815717 ) ) ;
#32486=CARTESIAN_POINT ( 'NONE',  ( 0.04044903254992426173, 13.86756916759064318, -30.02300923189239867 ) ) ;
#32487=CARTESIAN_POINT ( 'NONE',  ( -15.01150461594595775, 55.68489583333332860, 26.00068869287368756 ) ) ;
#32500=CARTESIAN_POINT ( 'NONE',  ( 19.06425588902592239, 22.03163166759064495, 19.11951029504763611 ) ) ;
#32505=CARTESIAN_POINT ( 'NONE',  ( -20.50609665440969209, 55.82812499999999289, 20.50609665441005092 ) ) ;
#32509=CARTESIAN_POINT ( 'NONE',  ( 28.01184896238304134, 34.05729166666666430, 7.505752307972846538 ) ) ;
#32514=CARTESIAN_POINT ( 'NONE',  ( 28.00173670424535644, 42.64545166574268364, -7.543491769121920321 ) ) ;
#32516=CARTESIAN_POINT ( 'NONE',  ( -20.50609665440969209, 62.70312500000000000, 20.50609665441005092 ) ) ;
#32521=CARTESIAN_POINT ( 'NONE',  ( -19.09188309203694445, 15.43749999999999645, -19.09188309203661049 ) ) ;
#32527=CARTESIAN_POINT ( 'NONE',  ( -13.97622843553588901, 35.05989583333332860, 24.20753774853756823 ) ) ;
#32534=CARTESIAN_POINT ( 'NONE',  ( 28.02196122052058413, 29.18190999907601579, 7.468012846824272799 ) ) ;
#32536=CARTESIAN_POINT ( 'NONE',  ( -26.06988505166722803, 30.61420166574267654, 7.025853678916877953 ) ) ;
#32541=CARTESIAN_POINT ( 'NONE',  ( 19.09188309203661049, 50.67187500000000000, -19.09188309203694445 ) ) ;
#32546=CARTESIAN_POINT ( 'NONE',  ( -7.505752307972844761, 28.04166666666666075, 28.01184896238304134 ) ) ;
#32547=CARTESIAN_POINT ( 'NONE',  ( -7.468012846824771955, 27.47434000092397000, -28.02196122052045624 ) ) ;
#32556=CARTESIAN_POINT ( 'NONE',  ( -0.04044903254990864921, 53.39881916759064495, 30.02300923189239867 ) ) ;
#32559=CARTESIAN_POINT ( 'NONE',  ( -28.01184896238304134, 18.58854166666666430, -7.505752307972844761 ) ) ;
#32563=CARTESIAN_POINT ( 'NONE',  ( -0.04044903255042732459, 45.36680583240934794, -27.95245687107223986 ) ) ;
#32569=CARTESIAN_POINT ( 'NONE',  ( 6.950374756619721595, 42.94309000092397355, 26.09010956794232428 ) ) ;
#32577=CARTESIAN_POINT ( 'NONE',  ( -7.543491769121917656, 58.97357666574269786, -28.00173670424536354 ) ) ;
#32580=CARTESIAN_POINT ( 'NONE',  ( 27.95245687107222921, 27.03906250000000000, -2.463307335887066074E-13 ) ) ;
#32583=CARTESIAN_POINT ( 'NONE',  ( -7.505752307973343918, 32.91145833333332860, -28.01184896238290989 ) ) ;
#32587=CARTESIAN_POINT ( 'NONE',  ( -26.02091320914849959, 53.97173583425732346, 14.97647472619947528 ) ) ;
#32589=CARTESIAN_POINT ( 'NONE',  ( -20.50609665441004736, 63.56249999999999289, -20.50609665440969565 ) ) ;
#32609=CARTESIAN_POINT ( 'NONE',  ( 6.950374756619721595, 12.00559000092397532, 26.09010956794232428 ) ) ;
#32615=CARTESIAN_POINT ( 'NONE',  ( -2.428612866367529427E-13, 46.80468750000000000, -27.95245687107223276 ) ) ;
#32616=CARTESIAN_POINT ( 'NONE',  ( -28.02196122052045268, 40.36496500092396644, 7.468012846824790607 ) ) ;
#32617=CARTESIAN_POINT ( 'NONE',  ( 30.02300923189239867, 29.03868083240935505, -0.04044903255044467877 ) ) ;
#32621=CARTESIAN_POINT ( 'NONE',  ( -26.09010956794245217, 54.96315999907602645, -6.950374756619243755 ) ) ;
#32631=CARTESIAN_POINT ( 'NONE',  ( 15.01150461594643204, 37.92447916666666430, 26.00068869287340334 ) ) ;
#32636=CARTESIAN_POINT ( 'NONE',  ( 7.505752307972854531, 57.26041666666666430, -28.01184896238303423 ) ) ;
#32643=CARTESIAN_POINT ( 'NONE',  ( -26.09010956794245217, 17.15065999907602290, -6.950374756619243755 ) ) ;
#32651=CARTESIAN_POINT ( 'NONE',  ( -13.97622843553632421, 43.08072916666666430, -24.20753774853731599 ) ) ;
#32656=CARTESIAN_POINT ( 'NONE',  ( 15.04653450569292872, 10.71652750092397888, -25.98046417659857710 ) ) ;
#32657=CARTESIAN_POINT ( 'NONE',  ( 26.00068869287340334, 50.81510416666667140, -15.01150461594642316 ) ) ;
#32668=CARTESIAN_POINT ( 'NONE',  ( 13.94119854578937812, 35.92486083425730214, 24.22776226481240514 ) ) ;
#32672=CARTESIAN_POINT ( 'NONE',  ( 15.01150461594643204, 65.42447916666667140, 26.00068869287340334 ) ) ;
#32676=CARTESIAN_POINT ( 'NONE',  ( 20.50609665440969565, 33.48437500000000000, -20.50609665441004736 ) ) ;
#32682=CARTESIAN_POINT ( 'NONE',  ( -26.02091320914878025, 44.79388916574269075, -14.97647472619899389 ) ) ;
#32684=CARTESIAN_POINT ( 'NONE',  ( 26.00068869287341045, 61.12760416666666430, -15.01150461594642493 ) ) ;
#32688=CARTESIAN_POINT ( 'NONE',  ( 27.95245687107223276, 66.85118083240935505, -0.04044903255042905932 ) ) ;
#32694=CARTESIAN_POINT ( 'NONE',  ( 6.988114217768294445, 34.63020833333332860, 26.07999730980477437 ) ) ;
#32699=CARTESIAN_POINT ( 'NONE',  ( -26.02091320914878025, 27.60638916574269075, -14.97647472619899389 ) ) ;
#32701=CARTESIAN_POINT ( 'NONE',  ( -0.04044903255042732459, 41.92930583240936215, -27.95245687107223986 ) ) ;
#32704=CARTESIAN_POINT ( 'NONE',  ( 27.95245687107222921, 64.85156249999998579, -2.463307335887066074E-13 ) ) ;
#32709=CARTESIAN_POINT ( 'NONE',  ( -15.01150461594595775, 21.30989583333331794, 26.00068869287368756 ) ) ;
#32710=CARTESIAN_POINT ( 'NONE',  ( -30.02300923189239867, 26.75819416759064495, -0.04044903254991731589 ) ) ;
#32720=CARTESIAN_POINT ( 'NONE',  ( 15.04653450569292872, 55.40402750092397355, -25.98046417659857710 ) ) ;
#32723=CARTESIAN_POINT ( 'NONE',  ( -20.50609665441004736, 32.62500000000000000, -20.50609665440969565 ) ) ;
#32730=CARTESIAN_POINT ( 'NONE',  ( 7.025853678916867295, 43.50482666574268364, 26.06988505166722803 ) ) ;
#32736=CARTESIAN_POINT ( 'NONE',  ( 19.11951029504763611, 52.10975666759065206, -19.06425588902591173 ) ) ;
#32743=CARTESIAN_POINT ( 'NONE',  ( -20.47846945139866648, 64.70274333240935505, 20.53372385742108008 ) ) ;
#32747=CARTESIAN_POINT ( 'NONE',  ( -13.97622843553588901, 24.74739583333332504, 24.20753774853756823 ) ) ;
#32750=CARTESIAN_POINT ( 'NONE',  ( 20.50609665440969565, 43.79687500000000000, -20.50609665441004736 ) ) ;
#32754=CARTESIAN_POINT ( 'NONE',  ( 28.00173670424549499, 49.24517333425730925, 7.543491769121417612 ) ) ;
#32756=CARTESIAN_POINT ( 'NONE',  ( 26.00068869287340334, 64.56510416666667140, -15.01150461594642316 ) ) ;
#32775=CARTESIAN_POINT ( 'NONE',  ( 26.06988505166735592, 11.43267333425730925, 7.025853678916393896 ) ) ;
#32780=CARTESIAN_POINT ( 'NONE',  ( 26.07999730980490227, 54.68229166666665719, 6.988114217767821046 ) ) ;
#32781=CARTESIAN_POINT ( 'NONE',  ( 0.04044903254992426173, 37.93006916759064495, -30.02300923189239867 ) ) ;
#32782=CARTESIAN_POINT ( 'NONE',  ( 7.543491769121922985, 26.31732666574268364, 28.00173670424535644 ) ) ;
#32786=CARTESIAN_POINT ( 'NONE',  ( 13.94119854578893580, 52.52826416574268364, -24.22776226481265383 ) ) ;
#32794=CARTESIAN_POINT ( 'NONE',  ( -15.01150461594642138, 32.76822916666666430, -26.00068869287340334 ) ) ;
#32798=CARTESIAN_POINT ( 'NONE',  ( -15.01150461594642138, 60.26822916666665009, -26.00068869287340334 ) ) ;
#32806=CARTESIAN_POINT ( 'NONE',  ( -26.09010956794245217, 24.02565999907602290, -6.950374756619243755 ) ) ;
#32814=CARTESIAN_POINT ( 'NONE',  ( 27.95245687107222921, 37.35156249999997868, -2.463307335887066074E-13 ) ) ;
#32820=CARTESIAN_POINT ( 'NONE',  ( -19.06425588902591173, 65.00038166759063074, -19.11951029504763611 ) ) ;
#32822=CARTESIAN_POINT ( 'NONE',  ( -26.00068869287368756, 49.66927083333330728, -15.01150461594595775 ) ) ;
#32833=CARTESIAN_POINT ( 'NONE',  ( -0.04044903254992426173, 36.21131916759064495, 27.95245687107223276 ) ) ;
#32838=CARTESIAN_POINT ( 'NONE',  ( -15.01150461594642138, 56.83072916666665009, -26.00068869287340334 ) ) ;
#32842=CARTESIAN_POINT ( 'NONE',  ( -15.01150461594595775, 28.18489583333332860, 26.00068869287368756 ) ) ;
#32847=CARTESIAN_POINT ( 'NONE',  ( -14.97647472619899389, 43.93451416574269075, 26.02091320914878025 ) ) ;
#32849=CARTESIAN_POINT ( 'NONE',  ( 20.50609665440969565, 57.54687500000000000, -20.50609665441004736 ) ) ;
#32852=CARTESIAN_POINT ( 'NONE',  ( 24.18731323226221974, 66.56472249907604066, -14.01125832528328985 ) ) ;
#32862=CARTESIAN_POINT ( 'NONE',  ( 14.97647472619900455, 21.59076416574269430, -26.02091320914876960 ) ) ;
#32864=CARTESIAN_POINT ( 'NONE',  ( -13.94119854578892514, 40.49701416574269786, 24.22776226481266448 ) ) ;
#32868=CARTESIAN_POINT ( 'NONE',  ( 6.988114217768294445, 58.69270833333332860, 26.07999730980477437 ) ) ;
#32873=CARTESIAN_POINT ( 'NONE',  ( 7.505752307973351023, 31.19270833333333215, 28.01184896238290278 ) ) ;
#32874=CARTESIAN_POINT ( 'NONE',  ( -30.02300923189239867, 30.19569416759064140, -0.04044903254991731589 ) ) ;
#32883=CARTESIAN_POINT ( 'NONE',  ( 15.04653450569292872, 58.84152750092397355, -25.98046417659857710 ) ) ;
#32886=CARTESIAN_POINT ( 'NONE',  ( 28.01184896238290278, 30.33333333333332860, -7.505752307973347470 ) ) ;
#32890=CARTESIAN_POINT ( 'NONE',  ( 19.11951029504797006, 43.21836833240935505, 19.06425588902558133 ) ) ;
#32896=CARTESIAN_POINT ( 'NONE',  ( -13.94119854578936923, 44.51861083425730214, -24.22776226481241224 ) ) ;
#32904=CARTESIAN_POINT ( 'NONE',  ( -20.53372385742107653, 65.56211833240934084, -20.47846945139867003 ) ) ;
#32910=CARTESIAN_POINT ( 'NONE',  ( -2.428612866367529427E-13, 33.05468750000000000, -27.95245687107222921 ) ) ;
#32913=CARTESIAN_POINT ( 'NONE',  ( -7.505752307972844761, 38.35416666666666430, 28.01184896238304134 ) ) ;
#32916=CARTESIAN_POINT ( 'NONE',  ( 14.97647472619947351, 63.42486083425730925, 26.02091320914850314 ) ) ;
#32917=CARTESIAN_POINT ( 'NONE',  ( -26.09010956794232428, 64.42746500092397355, 6.950374756619732253 ) ) ;
#32919=CARTESIAN_POINT ( 'NONE',  ( -7.505752307972844761, 65.85416666666665719, 28.01184896238304134 ) ) ;
#32940=CARTESIAN_POINT ( 'NONE',  ( -19.11951029504763611, 22.89100666759064495, 19.06425588902592239 ) ) ;
#32945=CARTESIAN_POINT ( 'NONE',  ( -26.02091320914849959, 47.09673583425730214, 14.97647472619947528 ) ) ;
#32946=CARTESIAN_POINT ( 'NONE',  ( -28.00173670424535644, 34.05170166574267654, 7.543491769121936308 ) ) ;
#32949=CARTESIAN_POINT ( 'NONE',  ( 24.18731323226221974, 63.12722249907601224, -14.01125832528328985 ) ) ;
#32953=CARTESIAN_POINT ( 'NONE',  ( 28.01184896238304134, 13.43229166666666607, 7.505752307972846538 ) ) ;
#32960=CARTESIAN_POINT ( 'NONE',  ( -28.01184896238304134, 35.77604166666666430, -7.505752307972844761 ) ) ;
#32966=CARTESIAN_POINT ( 'NONE',  ( -7.505752307973343918, 63.84895833333332860, -28.01184896238290989 ) ) ;
#32974=CARTESIAN_POINT ( 'NONE',  ( 0.04044903255044120238, 26.46055583240935505, 27.95245687107223276 ) ) ;
#32982=CARTESIAN_POINT ( 'NONE',  ( 26.07999730980477437, 47.52083333333332860, -6.988114217768290004 ) ) ;
#32987=CARTESIAN_POINT ( 'NONE',  ( 7.468012846824777284, 12.00559000092397532, 28.02196122052045268 ) ) ;
#32988=CARTESIAN_POINT ( 'NONE',  ( 7.505752307973351023, 62.13020833333334281, 28.01184896238290278 ) ) ;
#32998=CARTESIAN_POINT ( 'NONE',  ( -19.11951029504763611, 36.64100666759062364, 19.06425588902592239 ) ) ;
#33005=CARTESIAN_POINT ( 'NONE',  ( 7.505752307972854531, 57.26041666666666430, -28.01184896238303423 ) ) ;
#33009=CARTESIAN_POINT ( 'NONE',  ( 28.01184896238290278, 40.64583333333332860, -7.505752307973347470 ) ) ;
#33014=CARTESIAN_POINT ( 'NONE',  ( 15.04653450569339945, 53.67409749907601935, 25.98046417659831775 ) ) ;
#33016=CARTESIAN_POINT ( 'NONE',  ( 30.02300923189239867, 54.53906249999999289, -2.619432448724978208E-13 ) ) ;
#33021=CARTESIAN_POINT ( 'NONE',  ( -26.07999730980477437, 18.30208333333332860, 6.988114217768305103 ) ) ;
#33033=CARTESIAN_POINT ( 'NONE',  ( -7.468012846824272799, 26.60378499907601579, 28.02196122052058413 ) ) ;
#33035=CARTESIAN_POINT ( 'NONE',  ( 7.025853678916867295, 40.06732666574268364, 26.06988505166722803 ) ) ;
#33040=CARTESIAN_POINT ( 'NONE',  ( 26.07999730980477437, 61.27083333333332860, -6.988114217768290004 ) ) ;
#33046=CARTESIAN_POINT ( 'NONE',  ( 15.01150461594643204, 31.04947916666666075, 26.00068869287340334 ) ) ;
#33047=CARTESIAN_POINT ( 'NONE',  ( -7.468012846824771955, 30.91184000092396644, -28.02196122052045624 ) ) ;
#33058=CARTESIAN_POINT ( 'NONE',  ( -30.02300923189239512, 15.00781249999999467, 2.654126918244515359E-13 ) ) ;
#33061=CARTESIAN_POINT ( 'NONE',  ( 20.50609665441005092, 27.46875000000000000, 20.50609665440969209 ) ) ;
#33066=CARTESIAN_POINT ( 'NONE',  ( 26.06988505166722803, 39.20795166574269075, -7.025853678916862854 ) ) ;
#33073=CARTESIAN_POINT ( 'NONE',  ( -19.06425588902591173, 44.37538166759063785, -19.11951029504763611 ) ) ;
#33078=CARTESIAN_POINT ( 'NONE',  ( -19.79898987322349768, 11.99999999999999645, -19.79898987322315307 ) ) ;
#33082=CARTESIAN_POINT ( 'NONE',  ( -28.02196122052058413, 61.83815999907601935, -7.468012846824272799 ) ) ;
#33087=CARTESIAN_POINT ( 'NONE',  ( -19.09188309203694445, 36.06250000000000000, -19.09188309203661049 ) ) ;
#33090=CARTESIAN_POINT ( 'NONE',  ( -20.50609665440969209, 38.64062500000000000, 20.50609665441005092 ) ) ;
#33093=CARTESIAN_POINT ( 'NONE',  ( -30.02300923189239867, 57.69569416759065206, -0.04044903254991731589 ) ) ;
#33094=CARTESIAN_POINT ( 'NONE',  ( 14.01125832528286352, 62.27902750092396644, -24.18731323226246843 ) ) ;
#33096=CARTESIAN_POINT ( 'NONE',  ( -15.04653450569338524, 17.58034749907602290, -25.98046417659831775 ) ) ;
#33116=CARTESIAN_POINT ( 'NONE',  ( 0.04044903254993986036, 20.74256916759064495, -27.95245687107223986 ) ) ;
#33121=CARTESIAN_POINT ( 'NONE',  ( -14.97647472619946285, 44.51861083425730214, -26.02091320914851025 ) ) ;
#33122=CARTESIAN_POINT ( 'NONE',  ( -20.47846945139866648, 40.64024333240936215, 20.53372385742108008 ) ) ;
#33125=CARTESIAN_POINT ( 'NONE',  ( 0.04044903255044120238, 60.83555583240935505, 27.95245687107223276 ) ) ;
#33128=CARTESIAN_POINT ( 'NONE',  ( 26.00068869287367335, 17.01302083333332504, 15.01150461594596308 ) ) ;
#33136=CARTESIAN_POINT ( 'NONE',  ( -30.02300923189239512, 32.19531250000000000, 2.654126918244515359E-13 ) ) ;
#33151=CARTESIAN_POINT ( 'NONE',  ( 13.94119854578893580, 25.02826416574268720, -24.22776226481265383 ) ) ;
#33160=CARTESIAN_POINT ( 'NONE',  ( -26.07999730980490583, 52.96354166666666430, -6.988114217767815717 ) ) ;
#33165=CARTESIAN_POINT ( 'NONE',  ( -7.468012846824771955, 20.59934000092397355, -28.02196122052045624 ) ) ;
#33166=CARTESIAN_POINT ( 'NONE',  ( -7.505752307972844761, 62.41666666666666430, 28.01184896238304134 ) ) ;
#33178=CARTESIAN_POINT ( 'NONE',  ( -14.01125832528285109, 29.62277750092397355, 24.18731323226248264 ) ) ;
#33186=CARTESIAN_POINT ( 'NONE',  ( -7.505752307973343918, 43.22395833333332860, -28.01184896238290989 ) ) ;
#33191=CARTESIAN_POINT ( 'NONE',  ( -30.02300923189239867, 54.81993083240935505, 0.04044903255044988294 ) ) ;
#33193=CARTESIAN_POINT ( 'NONE',  ( 7.505752307973351023, 58.69270833333332860, 28.01184896238290278 ) ) ;
#33198=CARTESIAN_POINT ( 'NONE',  ( 13.97622843553633665, 27.61197916666666430, 24.20753774853730889 ) ) ;
#33211=CARTESIAN_POINT ( 'NONE',  ( 26.09010956794244507, 36.05690999907600514, 6.950374756619249084 ) ) ;
#33217=CARTESIAN_POINT ( 'NONE',  ( -19.09188309203694445, 60.12500000000000000, -19.09188309203661049 ) ) ;
#33222=CARTESIAN_POINT ( 'NONE',  ( -7.505752307973343918, 29.47395833333332860, -28.01184896238290989 ) ) ;
#33223=CARTESIAN_POINT ( 'NONE',  ( -28.00173670424549499, 33.77642333425730214, -7.543491769121417612 ) ) ;
#33233=CARTESIAN_POINT ( 'NONE',  ( -14.97647472619946285, 61.70611083425731636, -26.02091320914851025 ) ) ;
#33236=CARTESIAN_POINT ( 'NONE',  ( -2.584737979205442066E-13, 33.05468750000000000, -30.02300923189239867 ) ) ;
#33242=CARTESIAN_POINT ( 'NONE',  ( -7.025853678916861966, 55.53607666574269075, -26.06988505166722803 ) ) ;
#33251=CARTESIAN_POINT ( 'NONE',  ( -0.04044903254992426173, 46.52381916759065206, 27.95245687107223276 ) ) ;
#33260=CARTESIAN_POINT ( 'NONE',  ( -7.543491769121917656, 62.41107666574269075, -28.00173670424536354 ) ) ;
#33265=CARTESIAN_POINT ( 'NONE',  ( 13.97622843553633665, 31.04947916666666075, 24.20753774853730889 ) ) ;
#33269=CARTESIAN_POINT ( 'NONE',  ( 20.50609665440969565, 40.35937499999999289, -20.50609665441004736 ) ) ;
#33272=CARTESIAN_POINT ( 'NONE',  ( 30.02300923189239867, 59.41444416759064495, 0.04044903254992252006 ) ) ;
#33273=CARTESIAN_POINT ( 'NONE',  ( -24.22776226481240514, 57.40923583425731636, 13.94119854578937812 ) ) ;
#33275=CARTESIAN_POINT ( 'NONE',  ( 7.543491769121922985, 16.00482666574268720, 28.00173670424535644 ) ) ;
#33295=CARTESIAN_POINT ( 'NONE',  ( -7.025853678916393008, 19.16704833425730570, 26.06988505166735592 ) ) ;
#33300=CARTESIAN_POINT ( 'NONE',  ( 20.47846945139902530, 49.53163166759063785, 20.53372385742071771 ) ) ;
#33302=CARTESIAN_POINT ( 'NONE',  ( -7.468012846824272799, 36.91628499907601224, 28.02196122052058413 ) ) ;
#33306=CARTESIAN_POINT ( 'NONE',  ( 6.950374756619257965, 62.69753499907601224, -26.09010956794244507 ) ) ;
#33315=CARTESIAN_POINT ( 'NONE',  ( -26.00068869287340334, 45.65885416666666430, 15.01150461594643382 ) ) ;
#33324=CARTESIAN_POINT ( 'NONE',  ( 15.01150461594596486, 16.15364583333333215, -26.00068869287367690 ) ) ;
#33330=CARTESIAN_POINT ( 'NONE',  ( 19.11951029504797006, 26.03086833240935860, 19.06425588902558133 ) ) ;
#33338=CARTESIAN_POINT ( 'NONE',  ( -19.09188309203660694, 52.39062499999999289, 19.09188309203694800 ) ) ;
#33342=CARTESIAN_POINT ( 'NONE',  ( -24.20753774853730889, 28.47135416666666430, 13.97622843553634020 ) ) ;
#33344=CARTESIAN_POINT ( 'NONE',  ( 15.04653450569292872, 24.46652750092397355, -25.98046417659857710 ) ) ;
#33345=CARTESIAN_POINT ( 'NONE',  ( -20.50609665441004736, 60.12500000000000000, -20.50609665440969565 ) ) ;
#33356=CARTESIAN_POINT ( 'NONE',  ( -19.11951029504763611, 33.20350666759063074, 19.06425588902592239 ) ) ;
#33365=CARTESIAN_POINT ( 'NONE',  ( -28.01184896238304134, 42.65104166666666430, -7.505752307972844761 ) ) ;
#33370=CARTESIAN_POINT ( 'NONE',  ( -26.02091320914878025, 55.10638916574269786, -14.97647472619899389 ) ) ;
#33372=CARTESIAN_POINT ( 'NONE',  ( 15.01150461594596486, 64.27864583333332860, -26.00068869287367690 ) ) ;
#33377=CARTESIAN_POINT ( 'NONE',  ( -24.20753774853730889, 21.59635416666666785, 13.97622843553633842 ) ) ;
#33389=CARTESIAN_POINT ( 'NONE',  ( 24.22776226481265383, 39.63763916574268364, 13.94119854578893580 ) ) ;
#33393=CARTESIAN_POINT ( 'NONE',  ( -19.09188309203660694, 66.14062500000000000, 19.09188309203694800 ) ) ;
#33400=CARTESIAN_POINT ( 'NONE',  ( 28.01184896238304134, 34.05729166666666430, 7.505752307972846538 ) ) ;
#33401=CARTESIAN_POINT ( 'NONE',  ( 20.47846945139902530, 28.90663166759063785, 20.53372385742071771 ) ) ;
#33411=CARTESIAN_POINT ( 'NONE',  ( -15.01150461594595775, 14.43489583333332682, 26.00068869287368756 ) ) ;
#33414=CARTESIAN_POINT ( 'NONE',  ( 28.01184896238304134, 44.36979166666666430, 7.505752307972846538 ) ) ;
#33419=CARTESIAN_POINT ( 'NONE',  ( -26.09010956794245217, 51.52565999907602645, -6.950374756619243755 ) ) ;
#33425=CARTESIAN_POINT ( 'NONE',  ( 26.07999730980490227, 13.43229166666666607, 6.988114217767821046 ) ) ;
#33433=CARTESIAN_POINT ( 'NONE',  ( 20.53372385742108008, 67.28086833240935505, 20.47846945139866648 ) ) ;
#33438=CARTESIAN_POINT ( 'NONE',  ( 6.988114217768294445, 38.06770833333332860, 26.07999730980477437 ) ) ;
#33439=EDGE_LOOP ( 'NONE', ( #11615, #28082 ) ) ;
#33441=CARTESIAN_POINT ( 'NONE',  ( 26.00068869287340334, 40.50260416666666430, -15.01150461594642316 ) ) ;
#33444=CARTESIAN_POINT ( 'NONE',  ( -25.98046417659859486, 54.54465250092398776, -15.04653450569291628 ) ) ;
#33445=CARTESIAN_POINT ( 'NONE',  ( -24.18731323226248264, 61.41965250092398776, -14.01125832528284931 ) ) ;
#33448=CARTESIAN_POINT ( 'NONE',  ( -30.02300923189239867, 20.44493083240935150, 0.04044903255044988294 ) ) ;
#33467=CARTESIAN_POINT ( 'NONE',  ( -6.950374756619716266, 24.03684000092397000, -26.09010956794232428 ) ) ;
#33472=CARTESIAN_POINT ( 'NONE',  ( 25.98046417659858420, 45.95090250092398065, 15.04653450569292872 ) ) ;
#33474=CARTESIAN_POINT ( 'NONE',  ( -25.98046417659831420, 33.90847249907601935, 15.04653450569339945 ) ) ;
#33478=CARTESIAN_POINT ( 'NONE',  ( 27.95245687107223276, 63.41368083240934794, -0.04044903255042905932 ) ) ;
#33481=CARTESIAN_POINT ( 'NONE',  ( -20.50609665441004736, 11.99999999999999645, -20.50609665440969565 ) ) ;
#33489=CARTESIAN_POINT ( 'NONE',  ( -28.01184896238304134, 42.65104166666666430, -7.505752307972844761 ) ) ;
#33498=CARTESIAN_POINT ( 'NONE',  ( 30.02300923189239867, 16.72656249999999645, -2.619432448724978208E-13 ) ) ;
#33503=CARTESIAN_POINT ( 'NONE',  ( -26.09010956794245217, 27.46315999907601935, -6.950374756619243755 ) ) ;
#33511=CARTESIAN_POINT ( 'NONE',  ( -24.20753774853756823, 53.10677083333331439, -13.97622843553588723 ) ) ;
#33515=CARTESIAN_POINT ( 'NONE',  ( -6.988114217768288228, 32.91145833333332860, -26.07999730980477437 ) ) ;
#33517=CARTESIAN_POINT ( 'NONE',  ( 0.04044903254992426173, 17.30506916759064140, -30.02300923189239867 ) ) ;
#33518=CARTESIAN_POINT ( 'NONE',  ( -28.01184896238304134, 66.71354166666665719, -7.505752307972844761 ) ) ;
#33530=CARTESIAN_POINT ( 'NONE',  ( 0.04044903254993986036, 41.36756916759064495, -27.95245687107223986 ) ) ;
#33534=CARTESIAN_POINT ( 'NONE',  ( -15.01150461594595775, 14.43489583333332682, 26.00068869287368756 ) ) ;
#33538=CARTESIAN_POINT ( 'NONE',  ( -26.00068869287368756, 42.79427083333331439, -15.01150461594595775 ) ) ;
#33543=CARTESIAN_POINT ( 'NONE',  ( -14.97647472619899389, 50.80951416574269075, 26.02091320914878025 ) ) ;
#33550=CARTESIAN_POINT ( 'NONE',  ( -24.20753774853756823, 18.73177083333332149, -13.97622843553588723 ) ) ;
#33569=CARTESIAN_POINT ( 'NONE',  ( -26.06988505166735237, 16.58892333425730570, -7.025853678916388567 ) ) ;
#33573=CARTESIAN_POINT ( 'NONE',  ( 26.00068869287340334, 33.62760416666665719, -15.01150461594642316 ) ) ;
#33584=CARTESIAN_POINT ( 'NONE',  ( 15.01150461594596308, 16.15364583333333215, -26.00068869287367335 ) ) ;
#33587=CARTESIAN_POINT ( 'NONE',  ( 15.01150461594643382, 41.36197916666665719, 26.00068869287340334 ) ) ;
#33594=CARTESIAN_POINT ( 'NONE',  ( 24.22776226481265383, 56.82513916574268364, 13.94119854578893580 ) ) ;
#33599=CARTESIAN_POINT ( 'NONE',  ( 13.97622843553589966, 12.71614583333333037, -24.20753774853756113 ) ) ;
#33607=CARTESIAN_POINT ( 'NONE',  ( -27.95245687107223986, 20.44493083240935150, 0.04044903255043252877 ) ) ;
#33611=CARTESIAN_POINT ( 'NONE',  ( 2.584737979205441561E-13, 34.77343750000000000, 27.95245687107222921 ) ) ;
#33615=CARTESIAN_POINT ( 'NONE',  ( -28.01184896238290278, 49.23958333333332860, 7.505752307973363457 ) ) ;
#33618=CARTESIAN_POINT ( 'NONE',  ( -14.97647472619946285, 61.70611083425731636, -26.02091320914851025 ) ) ;
#33619=CARTESIAN_POINT ( 'NONE',  ( 6.950374756619721595, 56.69309000092396644, 26.09010956794232428 ) ) ;
#33622=CARTESIAN_POINT ( 'NONE',  ( 0.04044903255045854962, 19.58555583240935860, 30.02300923189239867 ) ) ;
#33627=CARTESIAN_POINT ( 'NONE',  ( -30.02300923189239512, 66.57031250000000000, 2.654126918244515359E-13 ) ) ;
#33644=CARTESIAN_POINT ( 'NONE',  ( 24.18731323226247554, 25.32590250092397710, 14.01125832528285997 ) ) ;
#33650=CARTESIAN_POINT ( 'NONE',  ( 14.97647472619900455, 35.34076416574268364, -26.02091320914876960 ) ) ;
#33654=CARTESIAN_POINT ( 'NONE',  ( -26.06988505166722803, 64.98920166574268364, 7.025853678916877953 ) ) ;
#33657=CARTESIAN_POINT ( 'NONE',  ( -28.01184896238290278, 14.86458333333333037, 7.505752307973363457 ) ) ;
#33664=CARTESIAN_POINT ( 'NONE',  ( -20.50609665441004736, 39.49999999999999289, -20.50609665440969565 ) ) ;
#33665=CARTESIAN_POINT ( 'NONE',  ( -2.584737979205441561E-13, 63.99218749999997868, -30.02300923189239512 ) ) ;
#33675=CARTESIAN_POINT ( 'NONE',  ( 28.01184896238290278, 13.14583333333332860, -7.505752307973347470 ) ) ;
#33680=CARTESIAN_POINT ( 'NONE',  ( -7.025853678916861966, 31.47357666574268364, -26.06988505166722803 ) ) ;
#33689=CARTESIAN_POINT ( 'NONE',  ( 24.20753774853756113, 47.95052083333331439, 13.97622843553589789 ) ) ;
#33693=CARTESIAN_POINT ( 'NONE',  ( 6.988114217767829928, 33.19791666666665719, -26.07999730980489872 ) ) ;
#33694=CARTESIAN_POINT ( 'NONE',  ( -20.47846945139902175, 23.75038166759064140, -20.53372385742072481 ) ) ;
#33696=CARTESIAN_POINT ( 'NONE',  ( -26.00068869287340334, 62.84635416666667851, 15.01150461594643382 ) ) ;
#33703=EDGE_CURVE ( 'NONE', #32341, #16033, #25503, .T. ) ;
#33708=CARTESIAN_POINT ( 'NONE',  ( 13.94119854578937812, 46.23736083425730925, 24.22776226481240514 ) ) ;
#33713=CARTESIAN_POINT ( 'NONE',  ( -28.01184896238290278, 14.86458333333333037, 7.505752307973363457 ) ) ;
#33718=CARTESIAN_POINT ( 'NONE',  ( -2.584737979205441561E-13, 39.92968750000000000, -30.02300923189239512 ) ) ;
#33719=CARTESIAN_POINT ( 'NONE',  ( -19.09188309203694445, 11.99999999999999645, -19.09188309203661049 ) ) ;
#33723=CARTESIAN_POINT ( 'NONE',  ( 26.02091320914876960, 56.82513916574268364, 14.97647472619900455 ) ) ;
#33730=CARTESIAN_POINT ( 'NONE',  ( 26.07999730980490227, 20.30729166666666430, 6.988114217767821046 ) ) ;
#33749=CARTESIAN_POINT ( 'NONE',  ( 24.18731323226247554, 18.45090250092397355, 14.01125832528285997 ) ) ;
#33756=CARTESIAN_POINT ( 'NONE',  ( -7.505752307973343918, 39.78645833333332860, -28.01184896238290989 ) ) ;
#33767=CARTESIAN_POINT ( 'NONE',  ( -28.00173670424549499, 61.27642333425730925, -7.543491769121417612 ) ) ;
#33769=CARTESIAN_POINT ( 'NONE',  ( 2.740863092043355209E-13, 38.21093750000000000, 30.02300923189239867 ) ) ;
#33775=CARTESIAN_POINT ( 'NONE',  ( 24.22776226481265383, 53.38763916574269786, 13.94119854578893580 ) ) ;
#33780=CARTESIAN_POINT ( 'NONE',  ( 24.20753774853731244, 13.00260416666666430, -13.97622843553633132 ) ) ;
#33788=CARTESIAN_POINT ( 'NONE',  ( -24.22776226481266448, 17.29388916574268720, -13.94119854578892514 ) ) ;
#33792=CARTESIAN_POINT ( 'NONE',  ( -24.20753774853730889, 45.65885416666666430, 13.97622843553633842 ) ) ;
#33795=CARTESIAN_POINT ( 'NONE',  ( 7.505752307972854531, 46.94791666666666430, -28.01184896238303423 ) ) ;
#33797=CARTESIAN_POINT ( 'NONE',  ( -28.01184896238304134, 15.15104166666666252, -7.505752307972844761 ) ) ;
#33798=CARTESIAN_POINT ( 'NONE',  ( -26.02091320914849959, 12.72173583425731458, 14.97647472619947528 ) ) ;
#33809=( NAMED_UNIT ( * ) SI_UNIT ( $, .STERADIAN. ) SOLID_ANGLE_UNIT ( ) );
#33818=CARTESIAN_POINT ( 'NONE',  ( -0.04044903254992426173, 25.89881916759064140, 27.95245687107223276 ) ) ;
#33824=CARTESIAN_POINT ( 'NONE',  ( 15.04653450569339945, 50.23659749907603356, 25.98046417659831775 ) ) ;
#33827=CARTESIAN_POINT ( 'NONE',  ( 19.09188309203694800, 17.15624999999999645, 19.09188309203660694 ) ) ;
#33831=CARTESIAN_POINT ( 'NONE',  ( -15.01150461594642138, 19.01822916666666785, -26.00068869287340334 ) ) ;
#33837=CARTESIAN_POINT ( 'NONE',  ( -26.00068869287368756, 46.23177083333331439, -15.01150461594595775 ) ) ;
#33838=CARTESIAN_POINT ( 'NONE',  ( -2.584737979205441561E-13, 57.11718750000000711, -30.02300923189239512 ) ) ;
#33849=CARTESIAN_POINT ( 'NONE',  ( 7.505752307973351023, 14.00520833333333215, 28.01184896238290278 ) ) ;
#33854=CARTESIAN_POINT ( 'NONE',  ( -24.22776226481266448, 34.48138916574268364, -13.94119854578892514 ) ) ;
#33861=CARTESIAN_POINT ( 'NONE',  ( -26.07999730980490583, 59.83854166666666430, -6.988114217767815717 ) ) ;
#33866=CARTESIAN_POINT ( 'NONE',  ( -6.988114217767819270, 45.22916666666665719, 26.07999730980490583 ) ) ;
#33867=CARTESIAN_POINT ( 'NONE',  ( 25.98046417659858420, 25.32590250092397710, 15.04653450569292872 ) ) ;
#33868=CARTESIAN_POINT ( 'NONE',  ( 25.98046417659831775, 21.87722249907602290, -15.04653450569338879 ) ) ;
#33877=CARTESIAN_POINT ( 'NONE',  ( 24.22776226481241224, 38.50298583425730925, -13.94119854578936923 ) ) ;
#33886=CARTESIAN_POINT ( 'NONE',  ( -26.00068869287368756, 46.23177083333331439, -15.01150461594595775 ) ) ;
#33891=CARTESIAN_POINT ( 'NONE',  ( -0.04044903255044120238, 62.55430583240935505, -30.02300923189239867 ) ) ;
#33893=CARTESIAN_POINT ( 'NONE',  ( 20.50609665440969565, 64.42187499999998579, -20.50609665441004736 ) ) ;
#33897=CARTESIAN_POINT ( 'NONE',  ( 13.97622843553589966, 64.27864583333332860, -24.20753774853756113 ) ) ;
#33900=CARTESIAN_POINT ( 'NONE',  ( -19.09188309203694445, 29.18749999999999645, -19.09188309203661049 ) ) ;
#33906=CARTESIAN_POINT ( 'NONE',  ( 27.95245687107223986, 45.66444416759065916, 0.04044903254993640479 ) ) ;
#33918=CARTESIAN_POINT ( 'NONE',  ( -14.01125832528285109, 19.31027750092397710, 24.18731323226248264 ) ) ;
#33922=CARTESIAN_POINT ( 'NONE',  ( 7.505752307973351023, 44.94270833333332860, 28.01184896238290278 ) ) ;
#33932=CARTESIAN_POINT ( 'NONE',  ( 25.98046417659831775, 35.62722249907602645, -15.04653450569338879 ) ) ;
#33934=CARTESIAN_POINT ( 'NONE',  ( 15.01150461594596486, 43.65364583333332860, -26.00068869287367690 ) ) ;
#33940=CARTESIAN_POINT ( 'NONE',  ( -7.025853678916861966, 52.09857666574269075, -26.06988505166722803 ) ) ;
#33945=CARTESIAN_POINT ( 'NONE',  ( -24.20753774853756823, 15.29427083333332860, -13.97622843553588723 ) ) ;
#33952=CARTESIAN_POINT ( 'NONE',  ( -26.06988505166722803, 16.86420166574268720, 7.025853678916877953 ) ) ;
#33956=CARTESIAN_POINT ( 'NONE',  ( 24.20753774853756113, 44.51302083333331439, 13.97622843553589789 ) ) ;
#33959=CARTESIAN_POINT ( 'NONE',  ( 30.02300923189239512, 47.66406249999998579, -2.619432448724977703E-13 ) ) ;
#33961=CARTESIAN_POINT ( 'NONE',  ( -0.04044903254990864921, 63.71131916759064495, 30.02300923189239867 ) ) ;
#33962=CARTESIAN_POINT ( 'NONE',  ( 30.02300923189239867, 14.72694416759064318, 0.04044903254992252006 ) ) ;
#33983=CARTESIAN_POINT ( 'NONE',  ( -24.18731323226248264, 27.04465250092397000, -14.01125832528284931 ) ) ;
ENDSEC;
END-ISO-10303-21;
